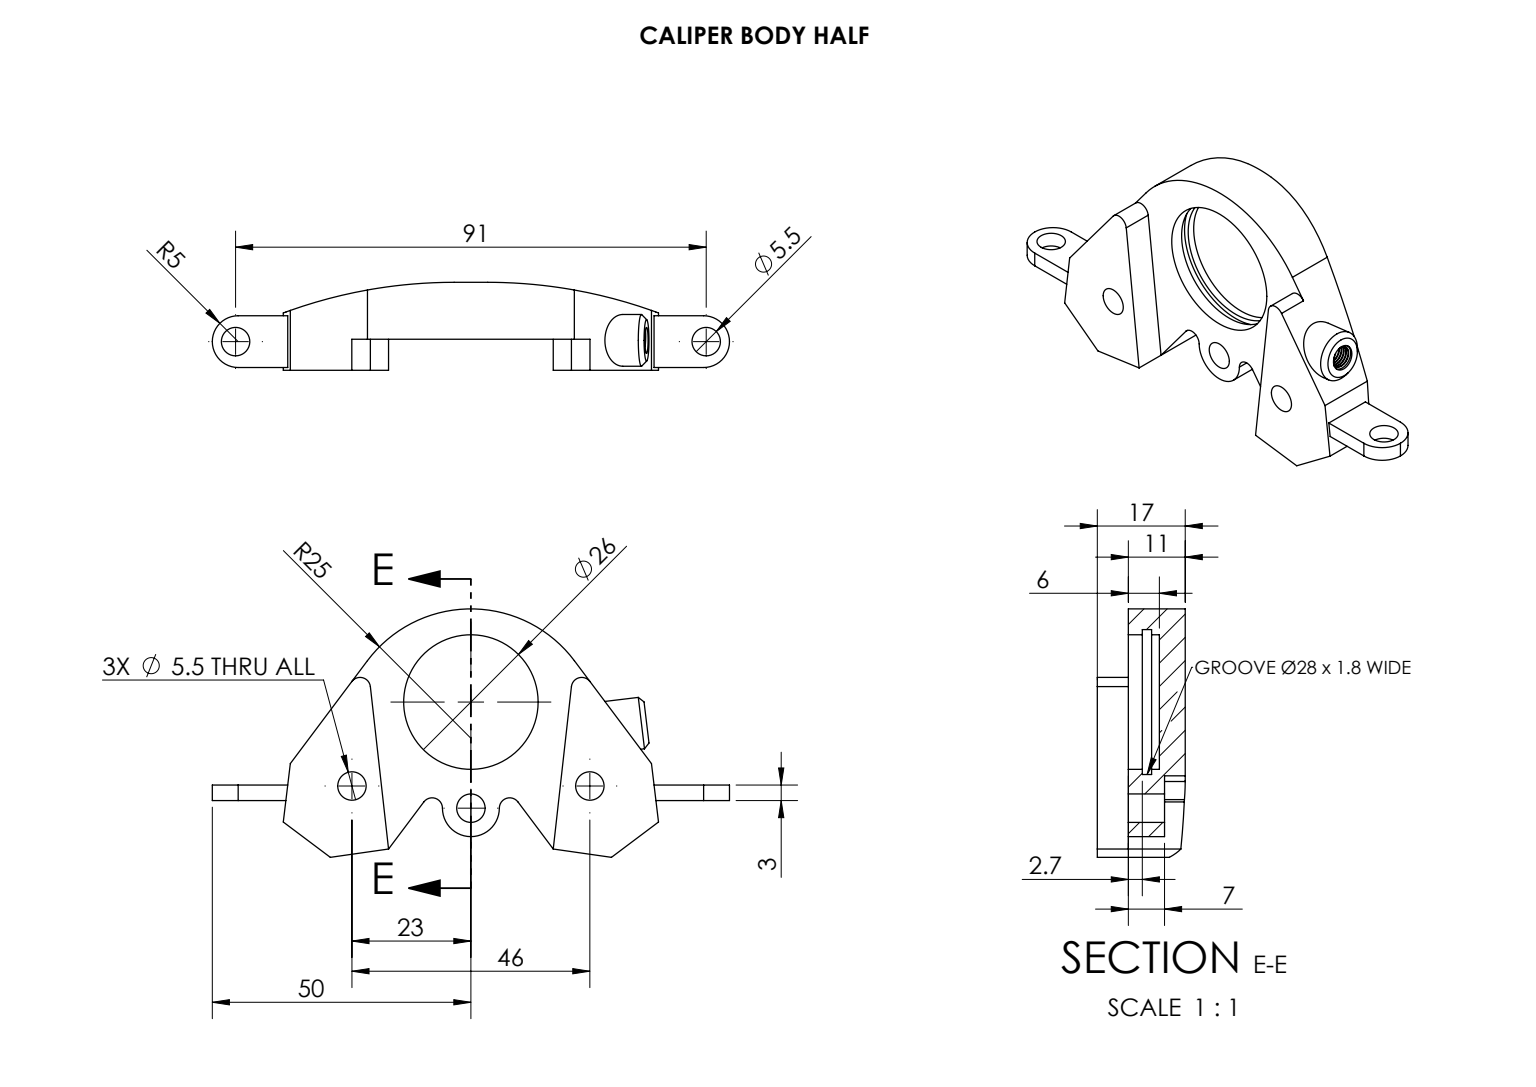
ISO-10303-21;
HEADER;
FILE_DESCRIPTION (('STEP AP214'),
    '1' );
FILE_NAME ('Caliper Body Half.step',
    '2026-09-24T10:28:59',
    ( '' ),
    ( '' ),
    'SwSTEP 2.0',
    'SolidWorks 2026',
    '' );
FILE_SCHEMA (( 'AUTOMOTIVE_DESIGN' ));
ENDSEC;

DATA;
#1=DIRECTION ( 'NONE',  ( 0.000000000000000000, 0.000000000000000000, 1.000000000000000000 ) ) ;
#7=CARTESIAN_POINT ( 'NONE',  ( 27.21934464581372737, -3.303641803799556964, -8.283357778048658915 ) ) ;
#8=CARTESIAN_POINT ( 'NONE',  ( 31.38469755857769528, -2.374701023479507178, -4.705209693361161349 ) ) ;
#10=DIRECTION ( 'NONE',  ( -0.1196152422706611984, 0.9928203230275510771, 0.000000000000000000 ) ) ;
#13=VECTOR ( 'NONE', #4443, 1000.000000000000000 ) ;
#14=EDGE_CURVE ( 'NONE', #9007, #1609, #16081, .T. ) ;
#19=AXIS2_PLACEMENT_3D ( 'NONE', #16442, #1032, #9441 ) ;
#22=CARTESIAN_POINT ( 'NONE',  ( 30.63309003953906995, -6.864245478665264244, -5.783357778048663356 ) ) ;
#23=ORIENTED_EDGE ( 'NONE', *, *, #13213, .T. ) ;
#25=ORIENTED_EDGE ( 'NONE', *, *, #5037, .F. ) ;
#26=CARTESIAN_POINT ( 'NONE',  ( 30.41294626588012306, -6.253601060580800564, -6.861505862736167138 ) ) ;
#29=VERTEX_POINT ( 'NONE', #10521 ) ;
#30=CARTESIAN_POINT ( 'NONE',  ( 26.73899421642883567, -2.634607751922174224, -4.533357778048659803 ) ) ;
#31=VECTOR ( 'NONE', #7104, 1000.000000000000114 ) ;
#36=EDGE_LOOP ( 'NONE', ( #1932, #7211, #3460, #1817 ) ) ;
#37=CARTESIAN_POINT ( 'NONE',  ( 16.95685998530892746, -17.86641812890577796, -16.00584995567978908 ) ) ;
#42=AXIS2_PLACEMENT_3D ( 'NONE', #3726, #1281, #2807 ) ;
#47=EDGE_CURVE ( 'NONE', #1330, #15856, #15716, .T. ) ;
#48=ORIENTED_EDGE ( 'NONE', *, *, #12351, .T. ) ;
#49=CARTESIAN_POINT ( 'NONE',  ( 33.55383270609817714, -5.448088258586239796, -3.283357778048667797 ) ) ;
#50=CARTESIAN_POINT ( 'NONE',  ( 29.97942892559193950, -4.424919740341219487, -3.627061608673664672 ) ) ;
#51=VECTOR ( 'NONE', #5337, 1000.000000000000000 ) ;
#52=FACE_OUTER_BOUND ( 'NONE', #13800, .T. ) ;
#70=CARTESIAN_POINT ( 'NONE',  ( 26.01652455409633902, -4.902371455920928156, -5.783357778048663356 ) ) ;
#75=ADVANCED_FACE ( 'NONE', ( #15989 ), #17272, .F. ) ;
#77=CIRCLE ( 'NONE', #17181, 2.000000000000001776 ) ;
#78=CARTESIAN_POINT ( 'NONE',  ( 16.79147592569384173, -15.38964587861223166, -16.02981638571824163 ) ) ;
#91=CARTESIAN_POINT ( 'NONE',  ( 26.87106449706838873, -6.053357334259913181, -3.627061608673667781 ) ) ;
#92=DIRECTION ( 'NONE',  ( 0.000000000000000000, 0.000000000000000000, 1.000000000000000000 ) ) ;
#93=CARTESIAN_POINT ( 'NONE',  ( 25.76466184735054910, -2.811881907026620553, -6.248149982130924762 ) ) ;
#94=CARTESIAN_POINT ( 'NONE',  ( 34.91600907648203389, -11.88801210197604341, -11.56671555609732671 ) ) ;
#99=CARTESIAN_POINT ( 'NONE',  ( 25.11802603177690330, -16.03270077640482683, -0.5379818257722508434 ) ) ;
#101=CARTESIAN_POINT ( 'NONE',  ( 28.51030546511822195, -6.055733689321201041, -3.283357778048667797 ) ) ;
#103=CARTESIAN_POINT ( 'NONE',  ( 30.62726312072365431, -1.838986382273682718, -5.783357778048658027 ) ) ;
#106=EDGE_CURVE ( 'NONE', #16432, #2761, #668, .T. ) ;
#110=ORIENTED_EDGE ( 'NONE', *, *, #14522, .T. ) ;
#113=ORIENTED_EDGE ( 'NONE', *, *, #12527, .T. ) ;
#115=ORIENTED_EDGE ( 'NONE', *, *, #562, .T. ) ;
#116=CARTESIAN_POINT ( 'NONE',  ( 28.26310972651430120, -2.123820177930694442, -5.783357778048658915 ) ) ;
#120=CARTESIAN_POINT ( 'NONE',  ( 30.15026255541241440, -6.285249260098253465, -4.705209693361168455 ) ) ;
#127=ADVANCED_FACE ( 'NONE', ( #4081 ), #12055, .F. ) ;
#134=CARTESIAN_POINT ( 'NONE',  ( -3.248936832696171617, 7.999999999999989342, -17.00000000000000000 ) ) ;
#138=CARTESIAN_POINT ( 'NONE',  ( 27.02867472334902033, -6.034368414549446058, -3.627061608673668225 ) ) ;
#139=CARTESIAN_POINT ( 'NONE',  ( 33.14105852333657509, -6.224726188408045147, -4.533357778048668685 ) ) ;
#140=CARTESIAN_POINT ( 'NONE',  ( -2.016448651773435938E-27, -20.49999999999999645, -13.00000000000000178 ) ) ;
#141=CARTESIAN_POINT ( 'NONE',  ( 31.03206908560819954, -5.751910973953721751, -3.283357778048667797 ) ) ;
#144=CARTESIAN_POINT ( 'NONE',  ( 30.66050125466253107, -2.889050389913576655, -3.283357778048662023 ) ) ;
#146=ORIENTED_EDGE ( 'NONE', *, *, #8317, .T. ) ;
#163=CARTESIAN_POINT ( 'NONE',  ( 28.29479612530171551, -12.89112598890823946, -13.63906826012424922 ) ) ;
#164=DIRECTION ( 'NONE',  ( 1.000000000000000000, 0.000000000000000000, 0.000000000000000000 ) ) ;
#167=EDGE_LOOP ( 'NONE', ( #6855, #14181, #5684, #15430, #4604, #9201, #7856, #12095, #740, #13288, #12189, #5777, #2747, #13452, #12769, #7783, #17571, #8793, #8444, #8354, #17242, #15258, #14922, #10965, #8092, #5094, #9620, #17228, #363 ) ) ;
#169=FACE_BOUND ( 'NONE', #9729, .T. ) ;
#170=ORIENTED_EDGE ( 'NONE', *, *, #10749, .T. ) ;
#176=CARTESIAN_POINT ( 'NONE',  ( 25.99795558426325215, -4.648046406214923820, -3.627061608673664228 ) ) ;
#177=FACE_OUTER_BOUND ( 'NONE', #11097, .T. ) ;
#181=CARTESIAN_POINT ( 'NONE',  ( 31.97277696464621854, -6.702839660918840536, -5.783357778048663356 ) ) ;
#182=EDGE_CURVE ( 'NONE', #5342, #17048, #16351, .T. ) ;
#183=DIRECTION ( 'NONE',  ( 1.000000000000000000, 0.000000000000000000, 0.000000000000000000 ) ) ;
#185=CARTESIAN_POINT ( 'NONE',  ( -27.17934203385504333, -30.00000000000000355, -13.93658524716016878 ) ) ;
#186=CARTESIAN_POINT ( 'NONE',  ( 29.18195272205665347, -2.340279496617377664, -4.533357778048659803 ) ) ;
#188=CARTESIAN_POINT ( 'NONE',  ( 31.41114436565740320, -6.133337902414513820, -4.705209693361168455 ) ) ;
#194=EDGE_CURVE ( 'NONE', #11172, #2496, #13438, .T. ) ;
#206=( BOUNDED_CURVE ( )  B_SPLINE_CURVE ( 2, ( #6130, #9128, #12848, #438, #15840, #5943, #14486, #14392, #13119 ),
 .UNSPECIFIED., .F., .T. ) 
 B_SPLINE_CURVE_WITH_KNOTS ( ( 3, 2, 2, 2, 3 ),
 ( 0.6730769230769231282, 0.6794871794871795156, 0.6923076923076922906, 0.7051282051282051766, 0.7115384615384615641 ),
 .UNSPECIFIED. ) 
 CURVE ( )  GEOMETRIC_REPRESENTATION_ITEM ( )  RATIONAL_B_SPLINE_CURVE ( ( 0.9330127018922192983, 0.9330127018922198534, 1.000000000000000000, 0.8660254037844387076, 1.000000000000000000, 0.8660254037844387076, 1.000000000000000000, 0.9330127018922194093, 0.9330127018922194093 ) ) 
 REPRESENTATION_ITEM ( '' )  );
#208=CARTESIAN_POINT ( 'NONE',  ( 28.86293393808771057, -2.678523738846987357, -4.705209693361161349 ) ) ;
#213=ORIENTED_EDGE ( 'NONE', *, *, #17178, .T. ) ;
#218=EDGE_CURVE ( 'NONE', #17680, #17749, #13335, .T. ) ;
#222=CARTESIAN_POINT ( 'NONE',  ( -25.11802603177690330, -19.03270077640482683, -10.53798182577225084 ) ) ;
#227=VERTEX_POINT ( 'NONE', #1284 ) ;
#229=CARTESIAN_POINT ( 'NONE',  ( 25.93488947238681774, -5.606027099510431988, -7.939653947423663816 ) ) ;
#231=CARTESIAN_POINT ( 'NONE',  ( 31.74131510559286085, -5.666460835049168310, -3.283357778048667797 ) ) ;
#236=DIRECTION ( 'NONE',  ( 0.000000000000000000, 0.000000000000000000, 1.000000000000000000 ) ) ;
#244=CARTESIAN_POINT ( 'NONE',  ( 26.00347982711925710, -2.723222710571018279, -7.033357778048658027 ) ) ;
#257=CARTESIAN_POINT ( 'NONE',  ( 19.43845002722867221, 2.988003976273735596, -6.000000000000000000 ) ) ;
#261=VECTOR ( 'NONE', #7073, 1000.000000000000227 ) ;
#263=CARTESIAN_POINT ( 'NONE',  ( -9.099998387031003944, -19.29508120620799616, -16.81964500401478091 ) ) ;
#270=CARTESIAN_POINT ( 'NONE',  ( 23.00000000000000000, -16.21813761408365195, -13.00000000000000178 ) ) ;
#278=EDGE_CURVE ( 'NONE', #1298, #15606, #15319, .T. ) ;
#282=CARTESIAN_POINT ( 'NONE',  ( 28.88938074516742205, -6.437160617781993999, -4.705209693361168455 ) ) ;
#287=DIRECTION ( 'NONE',  ( -0.1196152422706621005, -0.9928203230275509661, 0.000000000000000000 ) ) ;
#292=CARTESIAN_POINT ( 'NONE',  ( -35.77680296528374271, -19.03270077640482683, -10.53798182577225084 ) ) ;
#294=CARTESIAN_POINT ( 'NONE',  ( -19.22778933661430756, -11.21824206523807099, -15.64718775662042560 ) ) ;
#295=ORIENTED_EDGE ( 'NONE', *, *, #12061, .T. ) ;
#298=CARTESIAN_POINT ( 'NONE',  ( 26.51200394741821498, -4.842675973971495296, -7.939653947423662039 ) ) ;
#301=CARTESIAN_POINT ( 'NONE',  ( 30.45225960443380231, -4.367952981209816343, -3.627061608673664672 ) ) ;
#307=EDGE_CURVE ( 'NONE', #987, #12566, #1185, .T. ) ;
#319=DIRECTION ( 'NONE',  ( -0.000000000000000000, 1.000000000000000000, 0.000000000000000000 ) ) ;
#325=CARTESIAN_POINT ( 'NONE',  ( 27.28266178881210280, -7.257709054644824853, -5.783357778048669573 ) ) ;
#326=ADVANCED_FACE ( 'NONE', ( #3086 ), #2732, .F. ) ;
#327=CARTESIAN_POINT ( 'NONE',  ( 31.11087420047036289, -5.742416513891037688, -3.283357778048667797 ) ) ;
#329=FACE_BOUND ( 'NONE', #8817, .T. ) ;
#331=CARTESIAN_POINT ( 'NONE',  ( 29.04699097144805364, -6.418171698071525100, -4.705209693361169343 ) ) ;
#338=VECTOR ( 'NONE', #16087, 1000.000000000000000 ) ;
#343=CARTESIAN_POINT ( 'NONE',  ( -36.27615609941022257, -23.17738945083361557, 0.000000000000000000 ) ) ;
#349=CARTESIAN_POINT ( 'NONE',  ( 33.56434302664245450, -9.029166375164061620, -5.783357778048662468 ) ) ;
#350=FACE_OUTER_BOUND ( 'NONE', #12268, .T. ) ;
#353=CARTESIAN_POINT ( 'NONE',  ( -23.00000000000000000, -16.21813761408365195, -13.00000000000000178 ) ) ;
#354=AXIS2_PLACEMENT_3D ( 'NONE', #5840, #1963, #15742 ) ;
#363=ORIENTED_EDGE ( 'NONE', *, *, #1585, .T. ) ;
#376=AXIS2_PLACEMENT_3D ( 'NONE', #11104, #8407, #9745 ) ;
#380=CARTESIAN_POINT ( 'NONE',  ( 29.62036837594175154, -3.214238380052812261, -3.627061608673662896 ) ) ;
#382=DIRECTION ( 'NONE',  ( -0.000000000000000000, -0.000000000000000000, 1.000000000000000000 ) ) ;
#383=CARTESIAN_POINT ( 'NONE',  ( 25.97837335112617652, -4.585712065882579402, -3.626324104489874411 ) ) ;
#386=FACE_OUTER_BOUND ( 'NONE', #5358, .T. ) ;
#393=CYLINDRICAL_SURFACE ( 'NONE', #607, 6.249999999999998224 ) ;
#396=CARTESIAN_POINT ( 'NONE',  ( 28.54354359905709160, -7.105797696961086096, -5.783357778048669573 ) ) ;
#398=CARTESIAN_POINT ( 'NONE',  ( 31.25770402584614516, -1.763030703431812674, -5.783357778048658027 ) ) ;
#399=CARTESIAN_POINT ( 'NONE',  ( 33.95908713831674675, -3.945449517755636126, -5.783357778048663356 ) ) ;
#400=CARTESIAN_POINT ( 'NONE',  ( 25.71748644841968456, -2.420320648352051851, -5.783357778048663356 ) ) ;
#401=DIRECTION ( 'NONE',  ( 0.000000000000000000, 0.000000000000000000, -1.000000000000000000 ) ) ;
#402=ORIENTED_EDGE ( 'NONE', *, *, #10796, .T. ) ;
#404=DIRECTION ( 'NONE',  ( -0.6000000000000000888, -0.7999999999999999334, 0.000000000000000000 ) ) ;
#405=ORIENTED_EDGE ( 'NONE', *, *, #3183, .F. ) ;
#411=CARTESIAN_POINT ( 'NONE',  ( 25.71748644841968456, -2.420320648352051851, -5.783357778048663356 ) ) ;
#420=CARTESIAN_POINT ( 'NONE',  ( 25.76326615456878244, -3.051972493152843580, -6.861505862736158257 ) ) ;
#421=CARTESIAN_POINT ( 'NONE',  ( 30.38277803966508372, -1.468696967828331701, -5.783357778048658027 ) ) ;
#424=CARTESIAN_POINT ( 'NONE',  ( 29.76058531221316628, -5.705227139567997874, -7.939653947423664704 ) ) ;
#436=CARTESIAN_POINT ( 'NONE',  ( 25.98779870451785001, -2.387753359738024272, -6.453230759126469707 ) ) ;
#438=CARTESIAN_POINT ( 'NONE',  ( 28.51030546511822195, -6.055733689321201041, -3.283357778048667797 ) ) ;
#443=EDGE_CURVE ( 'NONE', #1609, #16681, #2190, .T. ) ;
#453=ORIENTED_EDGE ( 'NONE', *, *, #654, .T. ) ;
#456=CARTESIAN_POINT ( 'NONE',  ( 26.45077056032005913, -6.103994453487816330, -7.939653947423662927 ) ) ;
#458=FACE_BOUND ( 'NONE', #16476, .T. ) ;
#466=CARTESIAN_POINT ( 'NONE',  ( 33.56515079149260572, -5.873822666371450119, -6.861505862736167138 ) ) ;
#468=DIRECTION ( 'NONE',  ( -1.000000000000000000, 0.000000000000000000, 0.000000000000000000 ) ) ;
#474=CARTESIAN_POINT ( 'NONE',  ( -45.00000000000000711, -19.03270077640483038, -5.537981825772250843 ) ) ;
#479=CARTESIAN_POINT ( 'NONE',  ( 25.86833963875586306, -3.039313213345869791, -4.705209693361160461 ) ) ;
#481=CARTESIAN_POINT ( 'NONE',  ( 30.88125018618674744, -3.062327022369072171, -3.627061608673662896 ) ) ;
#487=CARTESIAN_POINT ( 'NONE',  ( -23.00000000000000000, -16.21813761408365195, 0.000000000000000000 ) ) ;
#491=ORIENTED_EDGE ( 'NONE', *, *, #2769, .T. ) ;
#492=FACE_OUTER_BOUND ( 'NONE', #1631, .T. ) ;
#495=CARTESIAN_POINT ( 'NONE',  ( -36.27615609941022257, -23.17738945083361557, 0.000000000000000000 ) ) ;
#496=VERTEX_POINT ( 'NONE', #3169 ) ;
#497=DIRECTION ( 'NONE',  ( 0.000000000000000000, 0.000000000000000000, 1.000000000000000000 ) ) ;
#498=ADVANCED_FACE ( 'NONE', ( #4791 ), #9064, .T. ) ;
#505=DIRECTION ( 'NONE',  ( 0.7999999999999999334, -0.6000000000000001998, 0.000000000000000000 ) ) ;
#510=EDGE_CURVE ( 'NONE', #9324, #14027, #3441, .T. ) ;
#512=VERTEX_POINT ( 'NONE', #11862 ) ;
#521=CARTESIAN_POINT ( 'NONE',  ( 26.79905070906539777, -3.354278923027479209, -3.283357778048662023 ) ) ;
#538=DIRECTION ( 'NONE',  ( -1.000000000000000000, 0.000000000000000000, 0.000000000000000000 ) ) ;
#546=ORIENTED_EDGE ( 'NONE', *, *, #3072, .T. ) ;
#548=VERTEX_POINT ( 'NONE', #6338 ) ;
#550=CARTESIAN_POINT ( 'NONE',  ( 25.62757597683262034, -3.695291012717980994, -7.939653947423660263 ) ) ;
#559=CARTESIAN_POINT ( 'NONE',  ( 32.54050588463559990, -2.235448945602741766, -6.861505862736159145 ) ) ;
#562=EDGE_CURVE ( 'NONE', #5268, #9522, #10410, .T. ) ;
#565=CARTESIAN_POINT ( 'NONE',  ( 26.63030083514515312, -6.709335133632020387, -6.861505862736167138 ) ) ;
#566=CARTESIAN_POINT ( 'NONE',  ( 27.89118264539014547, -6.557423775948280742, -6.861505862736167138 ) ) ;
#570=CARTESIAN_POINT ( 'NONE',  ( 27.51889869220010354, -3.467423976192371082, -7.939653947423660263 ) ) ;
#572=CARTESIAN_POINT ( 'NONE',  ( 33.52375369703867847, -2.544085015380856518, -8.283357778048660691 ) ) ;
#573=DIRECTION ( 'NONE',  ( 0.000000000000000000, 0.000000000000000000, 1.000000000000000000 ) ) ;
#575=VECTOR ( 'NONE', #16775, 1000.000000000000000 ) ;
#582=EDGE_LOOP ( 'NONE', ( #8490, #11002, #7089, #14364 ) ) ;
#589=CARTESIAN_POINT ( 'NONE',  ( 27.89480254248674740, -2.495355674045408367, -7.033357778048658027 ) ) ;
#607=AXIS2_PLACEMENT_3D ( 'NONE', #12704, #14260, #1658 ) ;
#608=EDGE_CURVE ( 'NONE', #17849, #6537, #15603, .T. ) ;
#610=VECTOR ( 'NONE', #16049, 1000.000000000000000 ) ;
#613=B_SPLINE_CURVE_WITH_KNOTS ( 'NONE', 3,
 ( #7742, #1957, #7477, #13001 ),
 .UNSPECIFIED., .F., .F.,
 ( 4, 4 ),
 ( 4.336808689942017736E-19, 0.0003446252387907799432 ),
 .UNSPECIFIED. ) ;
#615=CARTESIAN_POINT ( 'NONE',  ( 33.46007730730551799, -5.886481946178435010, -4.705209693361169343 ) ) ;
#618=DIRECTION ( 'NONE',  ( -0.000000000000000000, 0.000000000000000000, -1.000000000000000000 ) ) ;
#621=AXIS2_PLACEMENT_3D ( 'NONE', #3165, #7357, #17152 ) ;
#622=CARTESIAN_POINT ( 'NONE',  ( 26.85044460880409645, -7.319979551716484067, -5.783357778048668685 ) ) ;
#630=FACE_OUTER_BOUND ( 'NONE', #1139, .T. ) ;
#637=CARTESIAN_POINT ( 'NONE',  ( 26.31284730449749532, -7.327874027665321144, -6.311983372246984914 ) ) ;
#640=EDGE_CURVE ( 'NONE', #12566, #987, #8142, .T. ) ;
#644=CARTESIAN_POINT ( 'NONE',  ( 26.46816385032927599, -3.594016774262162706, -3.627061608673662896 ) ) ;
#646=DIRECTION ( 'NONE',  ( 0.9928203230275512992, 0.1196152422706614898, -0.000000000000000000 ) ) ;
#650=CARTESIAN_POINT ( 'NONE',  ( 29.08935247050201767, -2.014077381790315702, -5.783357778048658027 ) ) ;
#651=CARTESIAN_POINT ( 'NONE',  ( 30.65370992780335868, -5.597623261208692469, -3.627061608673667781 ) ) ;
#654=EDGE_CURVE ( 'NONE', #11172, #12535, #8280, .T. ) ;
#656=CARTESIAN_POINT ( 'NONE',  ( 25.76466184735054910, -2.811881907026620553, -6.248149982130924762 ) ) ;
#660=CARTESIAN_POINT ( 'NONE',  ( 25.60565592828815440, -3.070961412863312034, -6.861505862736159145 ) ) ;
#661=DIRECTION ( 'NONE',  ( 0.9928203230275511881, 0.1196152422706614760, 0.000000000000000000 ) ) ;
#662=CARTESIAN_POINT ( 'NONE',  ( 27.21934464581372737, -3.303641803799556964, -8.283357778048660691 ) ) ;
#665=DIRECTION ( 'NONE',  ( -1.000000000000000000, 0.000000000000000000, 0.000000000000000000 ) ) ;
#668=( BOUNDED_CURVE ( )  B_SPLINE_CURVE ( 2, ( #3728, #6807, #10599, #14882, #17820, #3994, #2388, #2468, #7905 ),
 .UNSPECIFIED., .F., .T. ) 
 B_SPLINE_CURVE_WITH_KNOTS ( ( 3, 2, 2, 2, 3 ),
 ( 0.5961538461538461453, 0.6025641025641025328, 0.6153846153846154188, 0.6282051282051281937, 0.6346153846153846922 ),
 .UNSPECIFIED. ) 
 CURVE ( )  GEOMETRIC_REPRESENTATION_ITEM ( )  RATIONAL_B_SPLINE_CURVE ( ( 0.9330127018922194093, 0.9330127018922194093, 1.000000000000000000, 0.8660254037844387076, 1.000000000000000000, 0.8660254037844387076, 1.000000000000000000, 0.9330127018922187432, 0.9330127018922192983 ) ) 
 REPRESENTATION_ITEM ( '' )  );
#669=ORIENTED_EDGE ( 'NONE', *, *, #13024, .T. ) ;
#672=CARTESIAN_POINT ( 'NONE',  ( 33.78529456515154550, -6.484467084455913799, -5.783357778048663356 ) ) ;
#680=CARTESIAN_POINT ( 'NONE',  ( 28.76917853929504432, -3.116917426439186123, -3.283357778048662023 ) ) ;
#681=DIRECTION ( 'NONE',  ( 0.000000000000000000, 3.469446951953614189E-16, -1.000000000000000000 ) ) ;
#687=CARTESIAN_POINT ( 'NONE',  ( 27.42949161418789217, -3.278323244185609830, -3.283357778048662023 ) ) ;
#689=VECTOR ( 'NONE', #8945, 999.9999999999998863 ) ;
#703=CARTESIAN_POINT ( 'NONE',  ( 16.75000000000000000, -16.21813761408365195, -16.03574476417184513 ) ) ;
#706=CYLINDRICAL_SURFACE ( 'NONE', #12142, 2.499999999999999112 ) ;
#708=ORIENTED_EDGE ( 'NONE', *, *, #6551, .F. ) ;
#720=CARTESIAN_POINT ( 'NONE',  ( -18.31859240410168255, -20.37927276054855596, -15.79761704335050077 ) ) ;
#724=( BOUNDED_CURVE ( )  B_SPLINE_CURVE ( 2, ( #2368, #1077, #16328, #7886, #2524, #10922, #2617, #16488, #13677 ),
 .UNSPECIFIED., .F., .T. ) 
 B_SPLINE_CURVE_WITH_KNOTS ( ( 3, 2, 2, 2, 3 ),
 ( 0.5576923076923077094, 0.5641025641025640969, 0.5769230769230768718, 0.5897435897435897578, 0.5961538461538461453 ),
 .UNSPECIFIED. ) 
 CURVE ( )  GEOMETRIC_REPRESENTATION_ITEM ( )  RATIONAL_B_SPLINE_CURVE ( ( 0.9330127018922194093, 0.9330127018922194093, 1.000000000000000000, 0.8660254037844387076, 1.000000000000000000, 0.8660254037844387076, 1.000000000000000000, 0.9330127018922194093, 0.9330127018922194093 ) ) 
 REPRESENTATION_ITEM ( '' )  );
#728=ORIENTED_EDGE ( 'NONE', *, *, #15440, .F. ) ;
#730=CARTESIAN_POINT ( 'NONE',  ( 27.62849893492243325, -6.589071975465733644, -4.705209693361168455 ) ) ;
#736=EDGE_LOOP ( 'NONE', ( #2850, #16797, #4603, #10052 ) ) ;
#739=CARTESIAN_POINT ( 'NONE',  ( 30.25080928106424594, -3.138282701210941994, -3.627061608673662896 ) ) ;
#740=ORIENTED_EDGE ( 'NONE', *, *, #17456, .F. ) ;
#742=CARTESIAN_POINT ( 'NONE',  ( 45.50000000000000000, -16.03270077640482683, -8.287981825772241962 ) ) ;
#745=CARTESIAN_POINT ( 'NONE',  ( 27.65911562847151117, -5.958412735707574015, -3.627061608673668225 ) ) ;
#747=CARTESIAN_POINT ( 'NONE',  ( 27.47505859511117521, -2.218764776483033163, -5.783357778048658027 ) ) ;
#754=ORIENTED_EDGE ( 'NONE', *, *, #7062, .T. ) ;
#756=EDGE_CURVE ( 'NONE', #1298, #13310, #2088, .T. ) ;
#760=DIRECTION ( 'NONE',  ( 0.000000000000000000, 0.000000000000000000, -1.000000000000000000 ) ) ;
#761=VERTEX_POINT ( 'NONE', #2823 ) ;
#762=LINE ( 'NONE', #10269, #2689 ) ;
#765=CARTESIAN_POINT ( 'NONE',  ( 32.04575515724927470, -1.668086104879473730, -5.783357778048658915 ) ) ;
#767=CARTESIAN_POINT ( 'NONE',  ( 27.95866967485789090, -6.122194908100387245, -3.283357778048667797 ) ) ;
#774=FACE_OUTER_BOUND ( 'NONE', #2018, .T. ) ;
#782=EDGE_LOOP ( 'NONE', ( #7919, #8135, #1228, #9710 ) ) ;
#798=ORIENTED_EDGE ( 'NONE', *, *, #7563, .F. ) ;
#799=ORIENTED_EDGE ( 'NONE', *, *, #2607, .T. ) ;
#805=CARTESIAN_POINT ( 'NONE',  ( -16.96458082634299558, -17.85487492059188597, -16.00470661676384054 ) ) ;
#810=CARTESIAN_POINT ( 'NONE',  ( 30.00264913441657555, -6.940201157507134511, -5.783357778048657138 ) ) ;
#813=CARTESIAN_POINT ( 'NONE',  ( 33.35047706458318828, -2.764833946905071560, -7.939653947423660263 ) ) ;
#815=EDGE_LOOP ( 'NONE', ( #969, #7998, #5616, #17835 ) ) ;
#820=AXIS2_PLACEMENT_3D ( 'NONE', #12110, #886, #3877 ) ;
#824=CARTESIAN_POINT ( 'NONE',  ( 31.53813789838894621, -6.745008222462202774, -5.783357778048668685 ) ) ;
#826=EDGE_CURVE ( 'NONE', #11736, #17680, #13359, .T. ) ;
#828=CARTESIAN_POINT ( 'NONE',  ( 31.00199007654869732, -2.847907730748336697, -8.283357778048660691 ) ) ;
#835=CARTESIAN_POINT ( 'NONE',  ( 32.47301885516785092, -2.670677813450649474, -3.283357778048662023 ) ) ;
#836=CARTESIAN_POINT ( 'NONE',  ( 26.99805802979993885, -6.665027654307603022, -4.705209693361168455 ) ) ;
#838=CARTESIAN_POINT ( 'NONE',  ( -50.00000000000000000, -16.03270077640482683, -5.537981825772250843 ) ) ;
#846=ORIENTED_EDGE ( 'NONE', *, *, #2531, .T. ) ;
#847=DIRECTION ( 'NONE',  ( -0.000000000000000000, 1.000000000000000000, -0.000000000000000000 ) ) ;
#854=CARTESIAN_POINT ( 'NONE',  ( 30.25524682244395436, -4.391689130744175884, -3.283357778048664688 ) ) ;
#857=DIRECTION ( 'NONE',  ( 1.000000000000000000, 0.000000000000000000, 0.000000000000000000 ) ) ;
#859=ORIENTED_EDGE ( 'NONE', *, *, #7991, .T. ) ;
#866=ORIENTED_EDGE ( 'NONE', *, *, #16999, .T. ) ;
#868=EDGE_LOOP ( 'NONE', ( #110, #4824, #5826, #15634 ) ) ;
#871=DIRECTION ( 'NONE',  ( 0.9928203230275510771, 0.1196152422706614621, -0.000000000000000000 ) ) ;
#877=CARTESIAN_POINT ( 'NONE',  ( 32.72003615946069743, -2.840789625746940938, -7.939653947423660263 ) ) ;
#878=( BOUNDED_CURVE ( )  B_SPLINE_CURVE ( 3, ( #12266, #2658, #4104, #17834 ),
 .UNSPECIFIED., .F., .T. ) 
 B_SPLINE_CURVE_WITH_KNOTS ( ( 4, 4 ),
 ( 4.715434792643774742, 4.769085813125753859 ),
 .UNSPECIFIED. ) 
 CURVE ( )  GEOMETRIC_REPRESENTATION_ITEM ( )  RATIONAL_B_SPLINE_CURVE ( ( 1.000000000000000000, 0.9997601450507493936, 0.9997601450507493936, 1.000000000000000000 ) ) 
 REPRESENTATION_ITEM ( '' )  );
#885=CARTESIAN_POINT ( 'NONE',  ( 32.47301885516785092, -2.670677813450649918, -3.283357778048662023 ) ) ;
#886=DIRECTION ( 'NONE',  ( 0.000000000000000000, 1.000000000000000000, 3.469446951953614189E-16 ) ) ;
#900=CARTESIAN_POINT ( 'NONE',  ( 27.26436163736424945, -2.571311352887278190, -7.033357778048658027 ) ) ;
#905=CARTESIAN_POINT ( 'NONE',  ( 27.23882169172318513, -6.009049854935478052, -7.939653947423664704 ) ) ;
#907=CARTESIAN_POINT ( 'NONE',  ( 29.74110826630371207, -2.999819088432076786, -8.283357778048660691 ) ) ;
#910=CARTESIAN_POINT ( 'NONE',  ( 31.02146712245815507, -5.553315781884258229, -7.939653947423664704 ) ) ;
#913=CARTESIAN_POINT ( 'NONE',  ( -9.099998387031003944, -19.29508120620799616, -12.00000000000000000 ) ) ;
#917=ORIENTED_EDGE ( 'NONE', *, *, #307, .T. ) ;
#919=COLOUR_RGB ( '', 0.40784314, 0.44705882, 0.49803922) ;
#920=CARTESIAN_POINT ( 'NONE',  ( 33.42946061375642586, -6.517141185936593750, -5.783357778048668685 ) ) ;
#923=CARTESIAN_POINT ( 'NONE',  ( 31.24221605398236079, -5.726592414339752857, -8.283357778048664244 ) ) ;
#927=CARTESIAN_POINT ( 'NONE',  ( 30.80688261270428541, -4.325227911964988792, -3.283357778048664688 ) ) ;
#929=CARTESIAN_POINT ( 'NONE',  ( 28.14933959732260149, -3.391468297350501260, -7.939653947423660263 ) ) ;
#931=DIRECTION ( 'NONE',  ( 1.000000000000000000, 0.000000000000000000, 0.000000000000000000 ) ) ;
#933=CARTESIAN_POINT ( 'NONE',  ( 20.00000000000000000, 7.999999999999996447, -15.51150668642334374 ) ) ;
#938=EDGE_CURVE ( 'NONE', #6497, #761, #8426, .T. ) ;
#941=ORIENTED_EDGE ( 'NONE', *, *, #14365, .T. ) ;
#943=DIRECTION ( 'NONE',  ( -0.9937818688019538493, -0.1113444980252557837, 0.000000000000000000 ) ) ;
#947=VERTEX_POINT ( 'NONE', #13962 ) ;
#948=CARTESIAN_POINT ( 'NONE',  ( 26.92924972366625980, -7.310485091653801781, -5.783357778048657138 ) ) ;
#951=AXIS2_PLACEMENT_3D ( 'NONE', #9490, #8145, #8230 ) ;
#952=CARTESIAN_POINT ( 'NONE',  ( 29.98885399772409954, -6.604504582617394703, -4.533357778048668685 ) ) ;
#953=FACE_OUTER_BOUND ( 'NONE', #4533, .T. ) ;
#958=CARTESIAN_POINT ( 'NONE',  ( 25.76466184735054910, -2.811881907026620553, -6.248149982130924762 ) ) ;
#963=VERTEX_POINT ( 'NONE', #7084 ) ;
#969=ORIENTED_EDGE ( 'NONE', *, *, #6749, .F. ) ;
#970=CARTESIAN_POINT ( 'NONE',  ( -14.00000000000000178, 0.000000000000000000, -10.50000000000000000 ) ) ;
#974=CARTESIAN_POINT ( 'NONE',  ( 33.54323074294813267, -5.249493066516778050, -7.939653947423664704 ) ) ;
#977=DIRECTION ( 'NONE',  ( 0.000000000000000000, 1.000000000000000000, 0.000000000000000000 ) ) ;
#978=DIRECTION ( 'NONE',  ( 0.9928203230275511881, 0.1196152422706614482, 0.000000000000000000 ) ) ;
#980=CARTESIAN_POINT ( 'NONE',  ( 30.08145424927873535, -6.930706697444451336, -5.783357778048663356 ) ) ;
#981=CARTESIAN_POINT ( 'NONE',  ( 33.06225340847440464, -6.234220648470727433, -4.533357778048668685 ) ) ;
#985=EDGE_CURVE ( 'NONE', #8671, #5626, #17505, .T. ) ;
#987=VERTEX_POINT ( 'NONE', #5692 ) ;
#992=EDGE_CURVE ( 'NONE', #12531, #11629, #15318, .T. ) ;
#993=ORIENTED_EDGE ( 'NONE', *, *, #16072, .T. ) ;
#995=CARTESIAN_POINT ( 'NONE',  ( -1.917618200156724081E-28, -7.000000000000001776, 0.000000000000000000 ) ) ;
#997=CARTESIAN_POINT ( 'NONE',  ( 45.50000000000000000, -19.03270077640483038, -2.787981825772258837 ) ) ;
#1002=CARTESIAN_POINT ( 'NONE',  ( 26.37178701114681800, -2.351687214456304353, -5.783357778048658027 ) ) ;
#1005=CARTESIAN_POINT ( 'NONE',  ( 32.08959525433819238, -2.916745304588811649, -7.939653947423660263 ) ) ;
#1014=CARTESIAN_POINT ( 'NONE',  ( 27.49697864365563760, -2.843094376337701679, -6.861505862736159145 ) ) ;
#1015=( BOUNDED_CURVE ( )  B_SPLINE_CURVE ( 2, ( #2395, #4004, #11890, #2216, #3919, #7910, #7995, #9432, #7729 ),
 .UNSPECIFIED., .F., .T. ) 
 B_SPLINE_CURVE_WITH_KNOTS ( ( 3, 2, 2, 2, 3 ),
 ( 0.1346153846153846367, 0.1410256410256410242, 0.1538461538461538547, 0.1666666666666666574, 0.1730769230769231004 ),
 .UNSPECIFIED. ) 
 CURVE ( )  GEOMETRIC_REPRESENTATION_ITEM ( )  RATIONAL_B_SPLINE_CURVE ( ( 0.9330127018922194093, 0.9330127018922196314, 1.000000000000000000, 0.8660254037844387076, 1.000000000000000000, 0.8660254037844387076, 1.000000000000000000, 0.9330127018922190762, 0.9330127018922194093 ) ) 
 REPRESENTATION_ITEM ( '' )  );
#1016=CARTESIAN_POINT ( 'NONE',  ( 26.14833026707293939, -5.996374093462653931, -8.004211544232147091 ) ) ;
#1019=EDGE_CURVE ( 'NONE', #12756, #8671, #10603, .T. ) ;
#1020=CARTESIAN_POINT ( 'NONE',  ( 33.13353876934984754, -5.498725377814142945, -8.283357778048662468 ) ) ;
#1023=CARTESIAN_POINT ( 'NONE',  ( 32.02836186724004364, -4.178063784105134459, -7.939653947423662039 ) ) ;
#1024=CARTESIAN_POINT ( 'NONE',  ( -13.00000000000000178, 1.592040838891559293E-15, -12.00000000000000000 ) ) ;
#1025=FACE_OUTER_BOUND ( 'NONE', #3424, .T. ) ;
#1026=CARTESIAN_POINT ( 'NONE',  ( 18.99795248260418745, 9.336063356527739998, -15.69100717631305031 ) ) ;
#1030=FACE_OUTER_BOUND ( 'NONE', #16056, .T. ) ;
#1032=DIRECTION ( 'NONE',  ( 0.9928203230275512992, 0.1196152422706614898, -0.000000000000000000 ) ) ;
#1040=CARTESIAN_POINT ( 'NONE',  ( 27.46709037723411839, -6.908327297984874882, -4.533357778048668685 ) ) ;
#1041=DIRECTION ( 'NONE',  ( 1.000000000000000000, 0.000000000000000000, 0.000000000000000000 ) ) ;
#1053=ORIENTED_EDGE ( 'NONE', *, *, #7902, .T. ) ;
#1056=EDGE_CURVE ( 'NONE', #13311, #2108, #11302, .T. ) ;
#1058=CARTESIAN_POINT ( 'NONE',  ( 30.30787278169304244, -6.266260340387784566, -4.705209693361169343 ) ) ;
#1063=CARTESIAN_POINT ( 'NONE',  ( 0.000000000000000000, 0.000000000000000000, -10.50000000000000000 ) ) ;
#1064=ADVANCED_FACE ( 'NONE', ( #3085 ), #7359, .F. ) ;
#1073=ORIENTED_EDGE ( 'NONE', *, *, #2262, .F. ) ;
#1075=LINE ( 'NONE', #6598, #7885 ) ;
#1077=CARTESIAN_POINT ( 'NONE',  ( 28.50956232500783472, -2.083930644370540985, -6.453230759126464378 ) ) ;
#1079=EDGE_CURVE ( 'NONE', #5626, #14839, #12411, .T. ) ;
#1081=CARTESIAN_POINT ( 'NONE',  ( 27.86926259684567597, -5.933094176093606897, -7.939653947423664704 ) ) ;
#1082=CARTESIAN_POINT ( 'NONE',  ( 29.71979337562451207, -1.938121702948446323, -5.783357778048664244 ) ) ;
#1083=CARTESIAN_POINT ( 'NONE',  ( 30.80679339554874119, -2.444327062417882779, -6.861505862736158257 ) ) ;
#1089=CARTESIAN_POINT ( 'NONE',  ( -2.016448651773435938E-27, -20.49999999999999645, -17.00000000000000000 ) ) ;
#1091=CIRCLE ( 'NONE', #3704, 2.000000000000001776 ) ;
#1092=ORIENTED_EDGE ( 'NONE', *, *, #6411, .F. ) ;
#1094=CARTESIAN_POINT ( 'NONE',  ( 27.75549246765397271, -7.200742295513424374, -5.783357778048668685 ) ) ;
#1100=CARTESIAN_POINT ( 'NONE',  ( 30.67935139548315604, -7.248220074880824981, -5.783357778048669573 ) ) ;
#1101=CIRCLE ( 'NONE', #12980, 2.749999999999988454 ) ;
#1111=ADVANCED_FACE ( 'NONE', ( #3631 ), #15964, .F. ) ;
#1112=ORIENTED_EDGE ( 'NONE', *, *, #278, .T. ) ;
#1114=ORIENTED_EDGE ( 'NONE', *, *, #13801, .T. ) ;
#1115=DIRECTION ( 'NONE',  ( -0.1196152422706611984, 0.9928203230275510771, 0.000000000000000000 ) ) ;
#1119=FILL_AREA_STYLE ('',( #13542 ) ) ;
#1120=CARTESIAN_POINT ( 'NONE',  ( 32.81641299864316608, -4.083119185552795294, -7.939653947423662039 ) ) ;
#1122=CARTESIAN_POINT ( 'NONE',  ( 27.10304229683147526, -4.771467524953526329, -3.283357778048664688 ) ) ;
#1123=FACE_BOUND ( 'NONE', #12437, .T. ) ;
#1131=DIRECTION ( 'NONE',  ( -0.5999999999999999778, 0.7999999999999999334, -0.000000000000000000 ) ) ;
#1137=CARTESIAN_POINT ( 'NONE',  ( 13.00000000000000178, 0.000000000000000000, -6.000000000000000000 ) ) ;
#1138=EDGE_CURVE ( 'NONE', #9324, #12386, #9302, .T. ) ;
#1139=EDGE_LOOP ( 'NONE', ( #14257, #12890, #1424, #3754, #13267, #12091 ) ) ;
#1140=CARTESIAN_POINT ( 'NONE',  ( 32.87199790123699472, -1.558343308739095656, -5.783357778048663356 ) ) ;
#1141=EDGE_CURVE ( 'NONE', #11286, #5484, #11940, .T. ) ;
#1142=CARTESIAN_POINT ( 'NONE',  ( 29.14753769709988518, -3.271205139184214516, -3.627061608673662008 ) ) ;
#1145=DIRECTION ( 'NONE',  ( -0.000000000000000000, -0.000000000000000000, 1.000000000000000000 ) ) ;
#1157=ADVANCED_FACE ( 'NONE', ( #14513 ), #7792, .T. ) ;
#1161=VERTEX_POINT ( 'NONE', #7972 ) ;
#1168=CARTESIAN_POINT ( 'NONE',  ( 29.39961944441754227, -3.040961747597316744, -3.283357778048662023 ) ) ;
#1175=CARTESIAN_POINT ( 'NONE',  ( 23.43390247958827288, -9.970148115950962620, -14.83177094038517652 ) ) ;
#1178=CARTESIAN_POINT ( 'NONE',  ( 33.13163345120441505, -4.045141346131868154, -3.627061608673664672 ) ) ;
#1181=AXIS2_PLACEMENT_3D ( 'NONE', #7932, #13466, #1041 ) ;
#1185=CIRCLE ( 'NONE', #14801, 2.749999999999991118 ) ;
#1189=CARTESIAN_POINT ( 'NONE',  ( 28.14933959732260149, -3.391468297350500372, -7.939653947423660263 ) ) ;
#1191=CARTESIAN_POINT ( 'NONE',  ( -45.50000000000000000, -16.03270077640482683, -8.287981825772238409 ) ) ;
#1194=EDGE_CURVE ( 'NONE', #17090, #11418, #15122, .T. ) ;
#1195=DIRECTION ( 'NONE',  ( 0.000000000000000000, 0.000000000000000000, 1.000000000000000000 ) ) ;
#1196=CARTESIAN_POINT ( 'NONE',  ( 29.07687923786957285, -2.352938776424351008, -7.033357778048658027 ) ) ;
#1201=CARTESIAN_POINT ( 'NONE',  ( 30.49166216014303643, -4.363205751385915931, -8.283357778048662468 ) ) ;
#1202=CARTESIAN_POINT ( 'NONE',  ( 27.90727577511918867, -2.156494279411373061, -5.783357778048670461 ) ) ;
#1203=( BOUNDED_CURVE ( )  B_SPLINE_CURVE ( 2, ( #13490, #8126, #10907, #3786, #6418, #7870, #10825, #15012, #6769 ),
 .UNSPECIFIED., .F., .T. ) 
 B_SPLINE_CURVE_WITH_KNOTS ( ( 3, 2, 2, 2, 3 ),
 ( 0.6730769230769231282, 0.6794871794871795156, 0.6923076923076922906, 0.7051282051282051766, 0.7115384615384615641 ),
 .UNSPECIFIED. ) 
 CURVE ( )  GEOMETRIC_REPRESENTATION_ITEM ( )  RATIONAL_B_SPLINE_CURVE ( ( 0.9330127018922192983, 0.9330127018922198534, 1.000000000000000000, 0.8660254037844387076, 1.000000000000000000, 0.8660254037844387076, 1.000000000000000000, 0.9330127018922194093, 0.9330127018922194093 ) ) 
 REPRESENTATION_ITEM ( '' )  );
#1207=AXIS2_PLACEMENT_3D ( 'NONE', #15325, #4498, #15560 ) ;
#1217=CARTESIAN_POINT ( 'NONE',  ( 29.15206445563513071, -6.405512418264540209, -6.861505862736167138 ) ) ;
#1218=DIRECTION ( 'NONE',  ( 0.9928203230275511881, 0.1196152422706614898, 0.000000000000000000 ) ) ;
#1220=CIRCLE ( 'NONE', #12162, 25.00000000000000000 ) ;
#1221=CARTESIAN_POINT ( 'NONE',  ( 26.00347982711925710, -2.723222710571018279, -7.033357778048658027 ) ) ;
#1228=ORIENTED_EDGE ( 'NONE', *, *, #11996, .F. ) ;
#1233=ORIENTED_EDGE ( 'NONE', *, *, #16362, .F. ) ;
#1238=CARTESIAN_POINT ( 'NONE',  ( 9.099998387031005720, -19.29508120620799971, -16.81964500401478091 ) ) ;
#1239=CARTESIAN_POINT ( 'NONE',  ( 29.34898802046944155, -4.500875419183088866, -3.627061608673664672 ) ) ;
#1241=DIRECTION ( 'NONE',  ( -0.8243186046180107640, -0.5661261679878573094, 0.000000000000000000 ) ) ;
#1242=CIRCLE ( 'NONE', #15137, 2.749999999999991118 ) ;
#1245=LINE ( 'NONE', #16555, #5173 ) ;
#1249=CARTESIAN_POINT ( 'NONE',  ( -3.538288549924106796, -15.34800872113743431, -13.00000000000000178 ) ) ;
#1251=AXIS2_PLACEMENT_3D ( 'NONE', #8210, #8025, #13562 ) ;
#1253=ADVANCED_FACE ( 'NONE', ( #5403 ), #4162, .T. ) ;
#1255=ORIENTED_EDGE ( 'NONE', *, *, #3739, .F. ) ;
#1259=VERTEX_POINT ( 'NONE', #14780 ) ;
#1265=DIRECTION ( 'NONE',  ( -1.000000000000000000, 0.000000000000000000, 0.000000000000000000 ) ) ;
#1268=EDGE_CURVE ( 'NONE', #4798, #16432, #724, .T. ) ;
#1269=CARTESIAN_POINT ( 'NONE',  ( 27.95350797341489368, -12.38528642892598342, -13.73189064827997541 ) ) ;
#1272=CARTESIAN_POINT ( 'NONE',  ( 32.82963640218302004, -5.962437625020304388, -4.705209693361169343 ) ) ;
#1274=VERTEX_POINT ( 'NONE', #13589 ) ;
#1279=CARTESIAN_POINT ( 'NONE',  ( 28.34209327568754944, -5.876127416962207306, -7.939653947423662927 ) ) ;
#1280=CARTESIAN_POINT ( 'NONE',  ( 25.80685721358263152, -3.162108319002908896, -4.519686641326834398 ) ) ;
#1281=DIRECTION ( 'NONE',  ( 0.000000000000000000, 0.000000000000000000, -1.000000000000000000 ) ) ;
#1284=CARTESIAN_POINT ( 'NONE',  ( -5.499998387031001634, -20.49508120620799900, -6.000000000000000000 ) ) ;
#1286=ADVANCED_FACE ( 'NONE', ( #5143 ), #13418, .F. ) ;
#1287=CARTESIAN_POINT ( 'NONE',  ( 29.32081432955537892, -3.050456207659999475, -3.283357778048662023 ) ) ;
#1292=CARTESIAN_POINT ( 'NONE',  ( 26.01652455409633902, -4.902371455920928156, -5.783357778048663356 ) ) ;
#1293=ORIENTED_EDGE ( 'NONE', *, *, #12859, .F. ) ;
#1298=VERTEX_POINT ( 'NONE', #3975 ) ;
#1299=FACE_OUTER_BOUND ( 'NONE', #12715, .T. ) ;
#1301=CARTESIAN_POINT ( 'NONE',  ( 29.13014440709066832, -5.781182818409868140, -7.939653947423662927 ) ) ;
#1306=CARTESIAN_POINT ( 'NONE',  ( 25.63782166807609997, -6.407846580969937200, -7.820349034508990549 ) ) ;
#1316=CARTESIAN_POINT ( 'NONE',  ( 32.46178999037268653, -4.125844254797621957, -8.283357778048662468 ) ) ;
#1319=VERTEX_POINT ( 'NONE', #11722 ) ;
#1320=CARTESIAN_POINT ( 'NONE',  ( 30.80679339554874119, -2.444327062417882779, -6.861505862736158257 ) ) ;
#1322=DIRECTION ( 'NONE',  ( 1.000000000000000000, 0.000000000000000000, 0.000000000000000000 ) ) ;
#1327=DIRECTION ( 'NONE',  ( 0.9928203230275510771, 0.1196152422706614621, -0.000000000000000000 ) ) ;
#1328=CARTESIAN_POINT ( 'NONE',  ( 26.24741491880506672, -3.420740141806666301, -3.283357778048662023 ) ) ;
#1330=VERTEX_POINT ( 'NONE', #12825 ) ;
#1331=EDGE_LOOP ( 'NONE', ( #7762, #3457, #12304, #16903, #9576 ) ) ;
#1333=ADVANCED_FACE ( 'NONE', ( #8924 ), #14465, .F. ) ;
#1336=VERTEX_POINT ( 'NONE', #17292 ) ;
#1340=DIRECTION ( 'NONE',  ( -0.1196152422706611984, 0.9928203230275510771, 0.000000000000000000 ) ) ;
#1348=CARTESIAN_POINT ( 'NONE',  ( 29.78250536075762867, -6.329556739422670830, -6.861505862736167138 ) ) ;
#1351=CARTESIAN_POINT ( 'NONE',  ( 26.01652455409633902, -4.902371455920928156, -5.783357778048663356 ) ) ;
#1353=ORIENTED_EDGE ( 'NONE', *, *, #11046, .T. ) ;
#1358=CARTESIAN_POINT ( 'NONE',  ( 29.01637427789896151, -7.048830937829682064, -5.783357778048668685 ) ) ;
#1367=CARTESIAN_POINT ( 'NONE',  ( 28.12379965168153362, -6.829206799398704675, -7.033357778048666908 ) ) ;
#1370=CARTESIAN_POINT ( 'NONE',  ( 30.15026255541241440, -6.285249260098253465, -4.705209693361168455 ) ) ;
#1371=CARTESIAN_POINT ( 'NONE',  ( 36.27615609941022257, -23.17738945083361557, -11.07596365154449636 ) ) ;
#1375=AXIS2_PLACEMENT_3D ( 'NONE', #3181, #1841, #8814 ) ;
#1377=VERTEX_POINT ( 'NONE', #4564 ) ;
#1383=DIRECTION ( 'NONE',  ( 0.000000000000000000, -1.000000000000000000, -3.469446951953614189E-16 ) ) ;
#1387=CARTESIAN_POINT ( 'NONE',  ( 31.65190802758064592, -5.477360103042387074, -7.939653947423662927 ) ) ;
#1390=CARTESIAN_POINT ( 'NONE',  ( 26.20620856698912604, -7.060238655668615415, -4.533357778048668685 ) ) ;
#1400=LINE ( 'NONE', #9630, #8117 ) ;
#1402=ORIENTED_EDGE ( 'NONE', *, *, #10595, .F. ) ;
#1406=CARTESIAN_POINT ( 'NONE',  ( 32.90015225647083952, -1.554951264938056132, -5.113484796970854340 ) ) ;
#1407=CARTESIAN_POINT ( 'NONE',  ( 31.67382807612511542, -6.101689702897060030, -6.861505862736167138 ) ) ;
#1412=CARTESIAN_POINT ( 'NONE',  ( 34.91600907648203389, -11.88801210197604341, 0.000000000000000000 ) ) ;
#1417=VECTOR ( 'NONE', #15217, 1000.000000000000000 ) ;
#1419=AXIS2_PLACEMENT_3D ( 'NONE', #3389, #11806, #15730 ) ;
#1420=EDGE_CURVE ( 'NONE', #963, #1502, #1958, .T. ) ;
#1423=CARTESIAN_POINT ( 'NONE',  ( -45.50000000000000000, -16.03270077640482683, -2.787981825772262390 ) ) ;
#1424=ORIENTED_EDGE ( 'NONE', *, *, #11515, .F. ) ;
#1427=CYLINDRICAL_SURFACE ( 'NONE', #8088, 2.499999999999999112 ) ;
#1433=EDGE_CURVE ( 'NONE', #7967, #2890, #1775, .T. ) ;
#1436=CARTESIAN_POINT ( 'NONE',  ( 16.96391960790757736, -14.58372395263535282, -16.00480323547922978 ) ) ;
#1439=CARTESIAN_POINT ( 'NONE',  ( 28.39010325924584421, -2.735490497978389612, -4.705209693361160461 ) ) ;
#1441=DIRECTION ( 'NONE',  ( 0.000000000000000000, 0.000000000000000000, -1.000000000000000000 ) ) ;
#1446=EDGE_LOOP ( 'NONE', ( #9533, #453, #14937, #5270 ) ) ;
#1448=CARTESIAN_POINT ( 'NONE',  ( 28.45891156537951971, -2.090033060632186412, -5.783357778048670461 ) ) ;
#1449=DIRECTION ( 'NONE',  ( -0.8243186046180107640, 0.5661261679878573094, 0.000000000000000000 ) ) ;
#1451=CARTESIAN_POINT ( 'NONE',  ( 25.85239768453567066, -3.540099486550932983, -4.114102314938801186 ) ) ;
#1456=CARTESIAN_POINT ( 'NONE',  ( 30.04891049036066164, -7.324175753722694360, -5.783357778048669573 ) ) ;
#1459=EDGE_CURVE ( 'NONE', #8286, #11901, #12912, .T. ) ;
#1460=CARTESIAN_POINT ( 'NONE',  ( 29.38830135902312080, -2.615227339812091767, -6.861505862736159145 ) ) ;
#1462=PLANE ( 'NONE',  #17617 ) ;
#1463=DIRECTION ( 'NONE',  ( -0.000000000000000000, -1.000000000000000000, -0.000000000000000000 ) ) ;
#1474=CARTESIAN_POINT ( 'NONE',  ( -21.42089235853292806, -10.15736413759261048, -15.24668633003922658 ) ) ;
#1477=CARTESIAN_POINT ( 'NONE',  ( 29.55043834383900148, -5.730545699181964991, -3.627061608673668225 ) ) ;
#1478=DIRECTION ( 'NONE',  ( 1.000000000000000000, 0.000000000000000000, 0.000000000000000000 ) ) ;
#1482=CARTESIAN_POINT ( 'NONE',  ( 31.28415083292585663, -5.521667582366822202, -3.627061608673667781 ) ) ;
#1484=EDGE_CURVE ( 'NONE', #16203, #1319, #11637, .T. ) ;
#1489=CARTESIAN_POINT ( 'NONE',  ( 21.42986351335030548, -22.27113001973728146, -15.24426822127429659 ) ) ;
#1492=AXIS2_PLACEMENT_3D ( 'NONE', #7438, #13143, #12958 ) ;
#1496=AXIS2_PLACEMENT_3D ( 'NONE', #7257, #16878, #15316 ) ;
#1497=VERTEX_POINT ( 'NONE', #10357 ) ;
#1499=CARTESIAN_POINT ( 'NONE',  ( 32.29220775574281532, -1.628196571319322050, -6.453230759126467042 ) ) ;
#1502=VERTEX_POINT ( 'NONE', #948 ) ;
#1504=CARTESIAN_POINT ( 'NONE',  ( 27.26074174026764751, -6.633379454790151009, -6.861505862736167138 ) ) ;
#1506=CARTESIAN_POINT ( 'NONE',  ( 31.95146207396702565, -5.641142275435198528, -8.283357778048662468 ) ) ;
#1514=CARTESIAN_POINT ( 'NONE',  ( 27.27683486999669427, -2.232449958253242883, -5.783357778048658027 ) ) ;
#1520=CIRCLE ( 'NONE', #12232, 2.749999999999988454 ) ;
#1531=CARTESIAN_POINT ( 'NONE',  ( -34.91600907648203389, -11.88801210197604341, -11.56671555609732671 ) ) ;
#1533=CARTESIAN_POINT ( 'NONE',  ( 27.11150007966593733, -11.49307575575171469, -13.95470972894434780 ) ) ;
#1540=CARTESIAN_POINT ( 'NONE',  ( 29.89119874204131122, -2.254829357712824667, -4.533357778048659803 ) ) ;
#1547=FACE_OUTER_BOUND ( 'NONE', #13456, .T. ) ;
#1548=CARTESIAN_POINT ( 'NONE',  ( 25.75668387115780078, -2.745663783273349257, -5.690028976746116740 ) ) ;
#1549=CARTESIAN_POINT ( 'NONE',  ( -5.499998387031001634, -20.49508120620799900, -13.00000000000000178 ) ) ;
#1554=CARTESIAN_POINT ( 'NONE',  ( 27.38828526237195504, -6.917821758047558056, -4.533357778048668685 ) ) ;
#1557=CARTESIAN_POINT ( 'NONE',  ( 29.64681518302145591, -6.972875258987813574, -5.783357778048668685 ) ) ;
#1559=DIRECTION ( 'NONE',  ( 0.000000000000000000, 3.469446951953614189E-16, -1.000000000000000000 ) ) ;
#1564=ORIENTED_EDGE ( 'NONE', *, *, #1138, .T. ) ;
#1569=EDGE_CURVE ( 'NONE', #1274, #12756, #5097, .T. ) ;
#1571=CARTESIAN_POINT ( 'NONE',  ( -5.499998387031001634, -20.49508120620799900, -12.00000000000000000 ) ) ;
#1573=( BOUNDED_SURFACE ( )  B_SPLINE_SURFACE ( 1, 2, ( 
 ( #12339, #15155, #10777, #3833, #14804, #5258, #13707, #12060, #9430, #14886, #3734, #3917, #2392, #15059, #2472, #13529, #10864, #11981, #10684, #17564, #10605, #16172, #16262, #7908, #13443, #4001, #13616, #9515, #14968, #6813, #1023, #2555, #12256, #5343, #4270, #3174, #12784, #13970, #8, #12518, #15236, #11044, #4530, #8713, #16887, #4185, #188, #16693, #11409, #10048, #2814, #103, #9686, #8528, #16974, #5697, #9771, #8340, #12608, #15509, #6989, #4355, #15324, #16609, #11213, #13873, #9959, #2902, #8433, #5795, #1370, #5611, #5886, #380, #15598, #11126, #1460, #6894, #4449, #3006, #11310, #1557, #3091, #12422, #7090, #5525, #7267, #16787, #9867, #15421, #14060, #1646, #7180, #12689, #282, #8613, #14145, #1735, #17067, #13058, #11596, #6345, #17447, #15694, #12965, #4620, #3450, #4981, #10143, #7629, #10508, #17163, #11868, #8892, #6257, #8979, #17349, #13151, #730, #14523, #11775, #5972, #16069, #4711, #14426, #3543, #3275, #7536, #15784, #3638, #14247, #8808, #2010, #644, #14339, #4886, #10416, #9073, #1925, #15974, #14617, #13236, #7445, #2197, #11496, #2106, #10238, #6167, #11690, #550, #1833, #6067, #3361 ),
 ( #15875, #17260, #7710, #4796, #10318, #813, #7365, #12880, #466, #6608, #13330, #13685, #1178, #9160, #3716, #6444, #13427, #16153, #7977, #17886, #8059, #2532, #1272, #5324, #6792, #6697, #14699, #9240, #11962, #1005, #14786, #13513, #5414, #13596, #12234, #12320, #10848, #2375, #16416, #3981, #17806, #17546, #10929, #6530, #14952, #16495, #5066, #2281, #7799, #10668, #12044, #7892, #1083, #17631, #5149, #910, #9497, #10586, #8153, #12138, #17717, #3814, #16242, #15037, #3896, #9329, #5239, #14868, #2457, #10759, #16337, #9413, #2626, #11453, #11361, #15549, #4168, #16931, #6871, #424, #1348, #4067, #13850, #3130, #5839, #15215, #12734, #9667, #4489, #2718, #2795, #10095, #8239, #8320, #331, #11023, #8664, #14192, #1439, #17020, #10003, #11779, #4574, #13771, #5929, #1785, #12402, #9577, #5501, #6966, #7316, #12836, #16586, #15132, #16238, #1081, #566, #14263, #15713, #13423, #5146, #14865, #3711, #9235, #8731, #10665, #13328, #905, #5988, #10251, #5234, #1853, #11514, #10163, #10583, #1002, #10755, #17628, #6527, #16150, #12135, #5063, #14444, #12041, #8908, #3291, #479, #11615, #17180, #6439, #11960, #7381, #6087 ) ),
 .UNSPECIFIED., .F., .F., .T. ) 
 B_SPLINE_SURFACE_WITH_KNOTS ( ( 2, 2 ),
 ( 3, 2, 2, 2, 2, 2, 2, 2, 2, 2, 2, 2, 2, 2, 2, 2, 2, 2, 2, 2, 2, 2, 2, 2, 2, 2, 2, 2, 2, 2, 2, 2, 2, 2, 2, 2, 2, 2, 2, 2, 2, 2, 2, 2, 2, 2, 2, 2, 2, 2, 2, 2, 2, 2, 2, 2, 2, 2, 2, 2, 2, 2, 2, 2, 2, 2, 2, 2, 2, 2, 2, 2, 2, 2, 2, 2, 3 ),
 ( 0.000000000000000000, 1.000000000000000000 ),
 ( 0.000000000000000000, 0.01282051282051282007, 0.02564102564102564014, 0.03846153846153846367, 0.05128205128205128027, 0.06410256410256409687, 0.07692307692307692735, 0.08974358974358974395, 0.1025641025641025605, 0.1153846153846153910, 0.1282051282051281937, 0.1410256410256410242, 0.1538461538461538547, 0.1666666666666666574, 0.1794871794871794879, 0.1923076923076923184, 0.2051282051282051211, 0.2179487179487179516, 0.2307692307692307820, 0.2435897435897435848, 0.2564102564102563875, 0.2692307692307692180, 0.2820512820512820484, 0.2948717948717948789, 0.3076923076923077094, 0.3205128205128205399, 0.3333333333333333148, 0.3461538461538461453, 0.3589743589743589758, 0.3717948717948718063, 0.3846153846153846367, 0.3974358974358974117, 0.4102564102564102422, 0.4230769230769230727, 0.4358974358974359031, 0.4487179487179487336, 0.4615384615384615641, 0.4743589743589743390, 0.4871794871794871695, 0.5000000000000000000, 0.5128205128205127750, 0.5256410256410256610, 0.5384615384615384359, 0.5512820512820513219, 0.5641025641025640969, 0.5769230769230768718, 0.5897435897435897578, 0.6025641025641025328, 0.6153846153846154188, 0.6282051282051281937, 0.6410256410256410797, 0.6538461538461538547, 0.6666666666666666297, 0.6794871794871795156, 0.6923076923076922906, 0.7051282051282051766, 0.7179487179487179516, 0.7307692307692307265, 0.7435897435897436125, 0.7564102564102563875, 0.7692307692307692735, 0.7820512820512820484, 0.7948717948717948234, 0.8076923076923077094, 0.8205128205128204844, 0.8333333333333333703, 0.8461538461538461453, 0.8589743589743589203, 0.8717948717948718063, 0.8846153846153845812, 0.8974358974358974672, 0.9102564102564102422, 0.9230769230769231282, 0.9358974358974359031, 0.9487179487179486781, 0.9615384615384615641, 0.9690838366659333403 ),
 .UNSPECIFIED. ) 
 GEOMETRIC_REPRESENTATION_ITEM ( )  RATIONAL_B_SPLINE_SURFACE ( (
 ( 1.000000000000000000, 0.8660254037844387076, 1.000000000000000000, 0.8660254037844387076, 1.000000000000000000, 0.8660254037844387076, 1.000000000000000000, 0.8660254037844387076, 1.000000000000000000, 0.8660254037844387076, 1.000000000000000000, 0.8660254037844387076, 1.000000000000000000, 0.8660254037844387076, 1.000000000000000000, 0.8660254037844387076, 1.000000000000000000, 0.8660254037844387076, 1.000000000000000000, 0.8660254037844387076, 1.000000000000000000, 0.8660254037844387076, 1.000000000000000000, 0.8660254037844387076, 1.000000000000000000, 0.8660254037844387076, 1.000000000000000000, 0.8660254037844387076, 1.000000000000000000, 0.8660254037844387076, 1.000000000000000000, 0.8660254037844387076, 1.000000000000000000, 0.8660254037844387076, 1.000000000000000000, 0.8660254037844387076, 1.000000000000000000, 0.8660254037844387076, 1.000000000000000000, 0.8660254037844387076, 1.000000000000000000, 0.8660254037844387076, 1.000000000000000000, 0.8660254037844387076, 1.000000000000000000, 0.8660254037844387076, 1.000000000000000000, 0.8660254037844387076, 1.000000000000000000, 0.8660254037844387076, 1.000000000000000000, 0.8660254037844387076, 1.000000000000000000, 0.8660254037844387076, 1.000000000000000000, 0.8660254037844387076, 1.000000000000000000, 0.8660254037844387076, 1.000000000000000000, 0.8660254037844387076, 1.000000000000000000, 0.8660254037844387076, 1.000000000000000000, 0.8660254037844387076, 1.000000000000000000, 0.8660254037844387076, 1.000000000000000000, 0.8660254037844387076, 1.000000000000000000, 0.8660254037844387076, 1.000000000000000000, 0.8660254037844387076, 1.000000000000000000, 0.8660254037844387076, 1.000000000000000000, 0.8660254037844387076, 1.000000000000000000, 0.8660254037844387076, 1.000000000000000000, 0.8660254037844387076, 1.000000000000000000, 0.8660254037844387076, 1.000000000000000000, 0.8660254037844387076, 1.000000000000000000, 0.8660254037844387076, 1.000000000000000000, 0.8660254037844387076, 1.000000000000000000, 0.8660254037844387076, 1.000000000000000000, 0.8660254037844387076, 1.000000000000000000, 0.8660254037844387076, 1.000000000000000000, 0.8660254037844387076, 1.000000000000000000, 0.8660254037844387076, 1.000000000000000000, 0.8660254037844387076, 1.000000000000000000, 0.8660254037844387076, 1.000000000000000000, 0.8660254037844387076, 1.000000000000000000, 0.8660254037844387076, 1.000000000000000000, 0.8660254037844387076, 1.000000000000000000, 0.8660254037844387076, 1.000000000000000000, 0.8660254037844387076, 1.000000000000000000, 0.8660254037844387076, 1.000000000000000000, 0.8660254037844387076, 1.000000000000000000, 0.8660254037844387076, 1.000000000000000000, 0.8660254037844387076, 1.000000000000000000, 0.8660254037844387076, 1.000000000000000000, 0.8660254037844387076, 1.000000000000000000, 0.8660254037844387076, 1.000000000000000000, 0.8660254037844387076, 1.000000000000000000, 0.8660254037844387076, 1.000000000000000000, 0.8660254037844387076, 1.000000000000000000, 0.8660254037844387076, 1.000000000000000000, 0.8660254037844387076, 1.000000000000000000, 0.8660254037844387076, 1.000000000000000000, 0.8660254037844387076, 1.000000000000000000, 0.8660254037844387076, 1.000000000000000000, 0.8660254037844387076, 1.000000000000000000, 0.8660254037844387076, 1.000000000000000000, 0.8660254037844387076, 1.000000000000000000, 0.8660254037844387076, 1.000000000000000000, 0.9211506902921580142, 0.9351132093492240394),
 ( 1.000000000000000000, 0.8660254037844387076, 1.000000000000000000, 0.8660254037844387076, 1.000000000000000000, 0.8660254037844387076, 1.000000000000000000, 0.8660254037844387076, 1.000000000000000000, 0.8660254037844387076, 1.000000000000000000, 0.8660254037844387076, 1.000000000000000000, 0.8660254037844387076, 1.000000000000000000, 0.8660254037844387076, 1.000000000000000000, 0.8660254037844387076, 1.000000000000000000, 0.8660254037844387076, 1.000000000000000000, 0.8660254037844387076, 1.000000000000000000, 0.8660254037844387076, 1.000000000000000000, 0.8660254037844387076, 1.000000000000000000, 0.8660254037844387076, 1.000000000000000000, 0.8660254037844387076, 1.000000000000000000, 0.8660254037844387076, 1.000000000000000000, 0.8660254037844387076, 1.000000000000000000, 0.8660254037844387076, 1.000000000000000000, 0.8660254037844387076, 1.000000000000000000, 0.8660254037844387076, 1.000000000000000000, 0.8660254037844387076, 1.000000000000000000, 0.8660254037844387076, 1.000000000000000000, 0.8660254037844387076, 1.000000000000000000, 0.8660254037844387076, 1.000000000000000000, 0.8660254037844387076, 1.000000000000000000, 0.8660254037844387076, 1.000000000000000000, 0.8660254037844387076, 1.000000000000000000, 0.8660254037844387076, 1.000000000000000000, 0.8660254037844387076, 1.000000000000000000, 0.8660254037844387076, 1.000000000000000000, 0.8660254037844387076, 1.000000000000000000, 0.8660254037844387076, 1.000000000000000000, 0.8660254037844387076, 1.000000000000000000, 0.8660254037844387076, 1.000000000000000000, 0.8660254037844387076, 1.000000000000000000, 0.8660254037844387076, 1.000000000000000000, 0.8660254037844387076, 1.000000000000000000, 0.8660254037844387076, 1.000000000000000000, 0.8660254037844387076, 1.000000000000000000, 0.8660254037844387076, 1.000000000000000000, 0.8660254037844387076, 1.000000000000000000, 0.8660254037844387076, 1.000000000000000000, 0.8660254037844387076, 1.000000000000000000, 0.8660254037844387076, 1.000000000000000000, 0.8660254037844387076, 1.000000000000000000, 0.8660254037844387076, 1.000000000000000000, 0.8660254037844387076, 1.000000000000000000, 0.8660254037844387076, 1.000000000000000000, 0.8660254037844387076, 1.000000000000000000, 0.8660254037844387076, 1.000000000000000000, 0.8660254037844387076, 1.000000000000000000, 0.8660254037844387076, 1.000000000000000000, 0.8660254037844387076, 1.000000000000000000, 0.8660254037844387076, 1.000000000000000000, 0.8660254037844387076, 1.000000000000000000, 0.8660254037844387076, 1.000000000000000000, 0.8660254037844387076, 1.000000000000000000, 0.8660254037844387076, 1.000000000000000000, 0.8660254037844387076, 1.000000000000000000, 0.8660254037844387076, 1.000000000000000000, 0.8660254037844387076, 1.000000000000000000, 0.8660254037844387076, 1.000000000000000000, 0.8660254037844387076, 1.000000000000000000, 0.8660254037844387076, 1.000000000000000000, 0.8660254037844387076, 1.000000000000000000, 0.8660254037844387076, 1.000000000000000000, 0.8660254037844387076, 1.000000000000000000, 0.8660254037844387076, 1.000000000000000000, 0.8660254037844387076, 1.000000000000000000, 0.8660254037844387076, 1.000000000000000000, 0.8660254037844387076, 1.000000000000000000, 0.8660254037844387076, 1.000000000000000000, 0.8660254037844387076, 1.000000000000000000, 0.8660254037844387076, 1.000000000000000000, 0.8660254037844387076, 1.000000000000000000, 0.9211506902921580142, 0.9351132093492240394) ) ) 
 REPRESENTATION_ITEM ( '' )  SURFACE ( )  );
#1574=CARTESIAN_POINT ( 'NONE',  ( 30.80679339554874119, -2.444327062417882779, -6.861505862736158257 ) ) ;
#1577=EDGE_LOOP ( 'NONE', ( #14715, #6873, #14999, #11550, #16139 ) ) ;
#1578=CARTESIAN_POINT ( 'NONE',  ( 30.23341599105502908, -5.648260380436597394, -7.939653947423664704 ) ) ;
#1579=CYLINDRICAL_SURFACE ( 'NONE', #8368, 2.499999999999999112 ) ;
#1585=EDGE_CURVE ( 'NONE', #2866, #3447, #17811, .T. ) ;
#1590=CARTESIAN_POINT ( 'NONE',  ( 26.30109267735093681, -7.264319738512599933, -6.611283024552371934 ) ) ;
#1592=PLANE ( 'NONE',  #14781 ) ;
#1597=CARTESIAN_POINT ( 'NONE',  ( 26.49878054387835746, -2.963357534503999968, -4.705209693361160461 ) ) ;
#1598=CARTESIAN_POINT ( 'NONE',  ( 32.58190297908952004, -5.565186596593329149, -8.283357778048662468 ) ) ;
#1606=CARTESIAN_POINT ( 'NONE',  ( -45.50000000000000000, -16.03270077640482683, -5.537981825772250843 ) ) ;
#1608=( BOUNDED_CURVE ( )  B_SPLINE_CURVE ( 3, ( #6366, #5085, #11796, #10685 ),
 .UNSPECIFIED., .F., .T. ) 
 B_SPLINE_CURVE_WITH_KNOTS ( ( 4, 4 ),
 ( 3.141592653589793116, 6.283185307179586232 ),
 .UNSPECIFIED. ) 
 CURVE ( )  GEOMETRIC_REPRESENTATION_ITEM ( )  RATIONAL_B_SPLINE_CURVE ( ( 1.000000000000000000, 0.3333333333333333703, 0.3333333333333333703, 1.000000000000000000 ) ) 
 REPRESENTATION_ITEM ( '' )  );
#1609=VERTEX_POINT ( 'NONE', #5715 ) ;
#1614=DIRECTION ( 'NONE',  ( 0.000000000000000000, 1.000000000000000000, -0.000000000000000000 ) ) ;
#1618=LINE ( 'NONE', #2973, #11821 ) ;
#1621=DIRECTION ( 'NONE',  ( 0.9928203230275512992, 0.1196152422706614898, -0.000000000000000000 ) ) ;
#1625=CARTESIAN_POINT ( 'NONE',  ( -9.099998387031005720, -19.29508120620799971, -6.000000000000000000 ) ) ;
#1628=ORIENTED_EDGE ( 'NONE', *, *, #11996, .T. ) ;
#1630=LINE ( 'NONE', #7346, #7510 ) ;
#1631=EDGE_LOOP ( 'NONE', ( #11424, #1747, #3079, #10057 ) ) ;
#1632=ORIENTED_EDGE ( 'NONE', *, *, #12695, .T. ) ;
#1636=CARTESIAN_POINT ( 'NONE',  ( 26.21417678486618641, -2.370676134166772808, -5.783357778048658915 ) ) ;
#1639=DIRECTION ( 'NONE',  ( 0.7999999999999999334, 0.6000000000000000888, -0.000000000000000000 ) ) ;
#1646=CARTESIAN_POINT ( 'NONE',  ( 28.97253418081003673, -5.800171738120336151, -7.939653947423664704 ) ) ;
#1653=VERTEX_POINT ( 'NONE', #15613 ) ;
#1654=CARTESIAN_POINT ( 'NONE',  ( 16.75000000000000000, -16.21813761408365195, -13.00000000000000178 ) ) ;
#1656=EDGE_CURVE ( 'NONE', #12969, #2761, #3193, .T. ) ;
#1658=DIRECTION ( 'NONE',  ( -1.000000000000000000, 0.000000000000000000, 0.000000000000000000 ) ) ;
#1660=CARTESIAN_POINT ( 'NONE',  ( 28.98992747081926069, -3.290194058894681639, -3.627061608673662896 ) ) ;
#1661=CARTESIAN_POINT ( 'NONE',  ( 26.82722439997946395, -4.804698134550569044, -3.627061608673664672 ) ) ;
#1663=AXIS2_PLACEMENT_3D ( 'NONE', #7669, #2236, #10710 ) ;
#1664=CARTESIAN_POINT ( 'NONE',  ( 30.13703915187255689, -4.405930820630744371, -7.939653947423662039 ) ) ;
#1669=CARTESIAN_POINT ( 'NONE',  ( 29.91004888286193619, -6.613999042680076990, -4.533357778048668685 ) ) ;
#1670=VERTEX_POINT ( 'NONE', #7725 ) ;
#1680=DIRECTION ( 'NONE',  ( 0.000000000000000000, 1.000000000000000000, 0.000000000000000000 ) ) ;
#1682=CARTESIAN_POINT ( 'NONE',  ( 26.67454832010805532, -2.305013593294074514, -5.113484796970851676 ) ) ;
#1683=CARTESIAN_POINT ( 'NONE',  ( 33.83155592109562804, -6.868441680671474536, -5.783357778048669573 ) ) ;
#1684=CARTESIAN_POINT ( 'NONE',  ( 32.61569110240115776, -6.288022587442930522, -7.033357778048666908 ) ) ;
#1687=DIRECTION ( 'NONE',  ( 0.000000000000000000, 0.000000000000000000, 1.000000000000000000 ) ) ;
#1692=VECTOR ( 'NONE', #7368, 1000.000000000000000 ) ;
#1695=( BOUNDED_CURVE ( )  B_SPLINE_CURVE ( 2, ( #5317, #3629, #900, #16145, #10750, #2522, #17878, #6688, #12221 ),
 .UNSPECIFIED., .F., .T. ) 
 B_SPLINE_CURVE_WITH_KNOTS ( ( 3, 2, 2, 2, 3 ),
 ( 0.7115384615384615641, 0.7179487179487179516, 0.7307692307692307265, 0.7435897435897436125, 0.7500000000000000000 ),
 .UNSPECIFIED. ) 
 CURVE ( )  GEOMETRIC_REPRESENTATION_ITEM ( )  RATIONAL_B_SPLINE_CURVE ( ( 0.9330127018922194093, 0.9330127018922194093, 1.000000000000000000, 0.8660254037844387076, 1.000000000000000000, 0.8660254037844387076, 1.000000000000000000, 0.9330127018922194093, 0.9330127018922194093 ) ) 
 REPRESENTATION_ITEM ( '' )  );
#1704=DIRECTION ( 'NONE',  ( 0.9899494936611662466, 0.1414213562373111965, 0.000000000000000000 ) ) ;
#1705=CARTESIAN_POINT ( 'NONE',  ( -50.00000000000000000, -19.03270077640483038, -5.537981825772250843 ) ) ;
#1714=CONICAL_SURFACE ( 'NONE', #17075, 3.999999999999986677, 0.7853981633974400633 ) ;
#1716=EDGE_CURVE ( 'NONE', #17066, #14839, #5080, .T. ) ;
#1724=LINE ( 'NONE', #7254, #3871 ) ;
#1729=CARTESIAN_POINT ( 'NONE',  ( 31.29094215978502902, -2.813094711071706389, -3.283357778048662023 ) ) ;
#1730=DIRECTION ( 'NONE',  ( 0.000000000000000000, 0.000000000000000000, -1.000000000000000000 ) ) ;
#1735=CARTESIAN_POINT ( 'NONE',  ( 28.35948656569675919, -3.366149737736551906, -3.627061608673662896 ) ) ;
#1737=CARTESIAN_POINT ( 'NONE',  ( 32.34851646621051202, -1.621412483717243447, -5.113484796970854340 ) ) ;
#1747=ORIENTED_EDGE ( 'NONE', *, *, #9946, .T. ) ;
#1750=CARTESIAN_POINT ( 'NONE',  ( 45.50000000000000000, -19.03270077640483038, -5.537981825772250843 ) ) ;
#1751=ORIENTED_EDGE ( 'NONE', *, *, #14289, .F. ) ;
#1752=CARTESIAN_POINT ( 'NONE',  ( -19.91444112663254984, -10.77903654349075246, -15.52697452096630748 ) ) ;
#1753=ORIENTED_EDGE ( 'NONE', *, *, #14588, .F. ) ;
#1755=CARTESIAN_POINT ( 'NONE',  ( 27.02414796481377124, -2.900061135469103490, -6.861505862736158257 ) ) ;
#1756=CARTESIAN_POINT ( 'NONE',  ( 31.93198502805756789, -2.935734224299280548, -7.939653947423660263 ) ) ;
#1759=DIRECTION ( 'NONE',  ( -1.000000000000000000, 0.000000000000000000, -0.000000000000000000 ) ) ;
#1761=EDGE_CURVE ( 'NONE', #6497, #8021, #12796, .T. ) ;
#1767=EDGE_CURVE ( 'NONE', #2633, #13499, #4683, .T. ) ;
#1770=CARTESIAN_POINT ( 'NONE',  ( 2.749999999999992895, -20.49999999999999645, -6.000000000000000000 ) ) ;
#1773=EDGE_LOOP ( 'NONE', ( #5510, #13248, #5935, #4030 ) ) ;
#1775=LINE ( 'NONE', #11444, #15386 ) ;
#1777=CARTESIAN_POINT ( 'NONE',  ( 26.90793483298705979, -6.248787706170159773, -8.283357778048664244 ) ) ;
#1778=VECTOR ( 'NONE', #16902, 1000.000000000000000 ) ;
#1780=CARTESIAN_POINT ( 'NONE',  ( 26.60838078660069428, -6.085005533777348319, -7.939653947423664704 ) ) ;
#1781=CARTESIAN_POINT ( 'NONE',  ( 31.83134908525019213, -4.201799933639492224, -8.283357778048662468 ) ) ;
#1785=CARTESIAN_POINT ( 'NONE',  ( 28.54354359905709870, -7.105797696961086096, -5.783357778048669573 ) ) ;
#1787=VECTOR ( 'NONE', #1827, 1000.000000000000000 ) ;
#1789=CARTESIAN_POINT ( 'NONE',  ( 20.00000000000000355, 7.999999999999996447, 0.000000000000000000 ) ) ;
#1795=ORIENTED_EDGE ( 'NONE', *, *, #16836, .F. ) ;
#1799=ORIENTED_EDGE ( 'NONE', *, *, #8255, .T. ) ;
#1801=ORIENTED_EDGE ( 'NONE', *, *, #8627, .T. ) ;
#1804=EDGE_CURVE ( 'NONE', #5110, #16117, #13702, .T. ) ;
#1810=AXIS2_PLACEMENT_3D ( 'NONE', #6953, #1621, #1340 ) ;
#1815=CARTESIAN_POINT ( 'NONE',  ( 29.79859849048667897, -1.928627242885762705, -5.783357778048664244 ) ) ;
#1816=VECTOR ( 'NONE', #17366, 1000.000000000000000 ) ;
#1817=ORIENTED_EDGE ( 'NONE', *, *, #14108, .F. ) ;
#1822=FACE_OUTER_BOUND ( 'NONE', #10493, .T. ) ;
#1823=CARTESIAN_POINT ( 'NONE',  ( -19.49912934580633106, 8.667827538924893105, -15.60122950519025409 ) ) ;
#1825=CARTESIAN_POINT ( 'NONE',  ( -28.59532824046058153, -19.01044845393195715, -13.55637998813296186 ) ) ;
#1827=DIRECTION ( 'NONE',  ( -0.000000000000000000, -0.000000000000000000, -1.000000000000000000 ) ) ;
#1829=CIRCLE ( 'NONE', #10767, 2.000000000000001776 ) ;
#1831=CARTESIAN_POINT ( 'NONE',  ( 26.14503574297738098, -5.691300421908874085, -8.283357778048664244 ) ) ;
#1833=CARTESIAN_POINT ( 'NONE',  ( 25.72395281601508898, -4.937620572523835349, -7.939653947423662039 ) ) ;
#1835=DIRECTION ( 'NONE',  ( 0.000000000000000000, 1.000000000000000000, 3.469446951953614189E-16 ) ) ;
#1837=LINE ( 'NONE', #9962, #1692 ) ;
#1841=DIRECTION ( 'NONE',  ( 0.000000000000000000, -0.000000000000000000, 1.000000000000000000 ) ) ;
#1844=ORIENTED_EDGE ( 'NONE', *, *, #1716, .F. ) ;
#1845=VERTEX_POINT ( 'NONE', #6808 ) ;
#1848=CARTESIAN_POINT ( 'NONE',  ( -17.40654580017221065, -13.42197210625884551, -15.93919332483364748 ) ) ;
#1850=EDGE_CURVE ( 'NONE', #16681, #13069, #16352, .T. ) ;
#1852=CARTESIAN_POINT ( 'NONE',  ( 27.89118264539014547, -6.557423775948280742, -6.861505862736167138 ) ) ;
#1853=CARTESIAN_POINT ( 'NONE',  ( 27.02867472334902033, -6.034368414549446058, -3.627061608673668225 ) ) ;
#1854=CARTESIAN_POINT ( 'NONE',  ( 29.60297508593253468, -5.724216059278466773, -7.939653947423664704 ) ) ;
#1856=CARTESIAN_POINT ( 'NONE',  ( 27.80031630502317341, -2.169380783275094426, -6.453230759126464378 ) ) ;
#1870=DIRECTION ( 'NONE',  ( 1.000000000000000000, 0.000000000000000000, -0.000000000000000000 ) ) ;
#1876=CARTESIAN_POINT ( 'NONE',  ( 31.64365984991007252, -1.316785610144591390, -5.783357778048658027 ) ) ;
#1878=ADVANCED_FACE ( 'NONE', ( #2643, #4266 ), #14964, .T. ) ;
#1890=DIRECTION ( 'NONE',  ( 0.000000000000000000, 0.000000000000000000, 1.000000000000000000 ) ) ;
#1891=ORIENTED_EDGE ( 'NONE', *, *, #9946, .F. ) ;
#1892=FACE_OUTER_BOUND ( 'NONE', #9347, .T. ) ;
#1895=CARTESIAN_POINT ( 'NONE',  ( 26.07857582428556853, -4.894895503279006022, -8.283357778048662468 ) ) ;
#1899=EDGE_CURVE ( 'NONE', #11176, #14870, #17899, .T. ) ;
#1908=EDGE_LOOP ( 'NONE', ( #4539, #14023, #8623, #6291 ) ) ;
#1914=CARTESIAN_POINT ( 'NONE',  ( -21.62109127008995557, -22.31747812791595464, -15.20678566061929615 ) ) ;
#1916=EDGE_CURVE ( 'NONE', #2334, #3411, #9512, .T. ) ;
#1917=DIRECTION ( 'NONE',  ( -1.000000000000000000, 0.000000000000000000, 0.000000000000000000 ) ) ;
#1925=CARTESIAN_POINT ( 'NONE',  ( 26.35439372113758694, -4.861664893681965083, -7.939653947423662039 ) ) ;
#1928=DIRECTION ( 'NONE',  ( 0.7999999999999999334, 0.6000000000000001998, -0.000000000000000000 ) ) ;
#1932=ORIENTED_EDGE ( 'NONE', *, *, #640, .T. ) ;
#1939=CARTESIAN_POINT ( 'NONE',  ( 28.28955653359400557, -5.882457056865704637, -3.627061608673668225 ) ) ;
#1941=CARTESIAN_POINT ( 'NONE',  ( 27.60205212784272177, -2.830435096530727446, -4.705209693361161349 ) ) ;
#1943=CARTESIAN_POINT ( 'NONE',  ( 33.79776779778399032, -6.145605689821873163, -7.033357778048666908 ) ) ;
#1952=CARTESIAN_POINT ( 'NONE',  ( -1.917618200156724081E-28, -7.000000000000001776, -17.00000000000000000 ) ) ;
#1954=VERTEX_POINT ( 'NONE', #185 ) ;
#1956=ORIENTED_EDGE ( 'NONE', *, *, #7800, .T. ) ;
#1957=CARTESIAN_POINT ( 'NONE',  ( 3.347071143357317702, -15.22052928361023127, -17.00000000000000000 ) ) ;
#1958=LINE ( 'NONE', #11102, #6988 ) ;
#1959=CARTESIAN_POINT ( 'NONE',  ( 26.78782184427022983, -4.809445364374452581, -8.283357778048662468 ) ) ;
#1960=CARTESIAN_POINT ( 'NONE',  ( 29.35841309260160159, -6.680460261459264970, -4.533357778048668685 ) ) ;
#1961=CARTESIAN_POINT ( 'NONE',  ( -3.248936832696171617, -15.16081378324841111, -17.00000000000000000 ) ) ;
#1963=DIRECTION ( 'NONE',  ( -0.000000000000000000, -0.000000000000000000, 1.000000000000000000 ) ) ;
#1964=CARTESIAN_POINT ( 'NONE',  ( 27.29063000668916672, -2.568146533142987575, -4.533357778048659803 ) ) ;
#1970=ORIENTED_EDGE ( 'NONE', *, *, #11657, .T. ) ;
#1980=CARTESIAN_POINT ( 'NONE',  ( 32.96626681528915981, -4.065064760026301016, -5.783357778048663356 ) ) ;
#1982=VECTOR ( 'NONE', #12816, 1000.000000000000000 ) ;
#1987=AXIS2_PLACEMENT_3D ( 'NONE', #1351, #6533, #17634 ) ;
#1991=ORIENTED_EDGE ( 'NONE', *, *, #15992, .T. ) ;
#1992=CIRCLE ( 'NONE', #6018, 2.749999999999988454 ) ;
#2006=CARTESIAN_POINT ( 'NONE',  ( 25.11802603177690330, -16.03270077640482683, -10.53798182577225084 ) ) ;
#2007=CARTESIAN_POINT ( 'NONE',  ( 30.00264913441657555, -6.940201157507134511, -5.783357778048657138 ) ) ;
#2010=CARTESIAN_POINT ( 'NONE',  ( 26.66961417369883591, -4.823687054261037055, -3.627061608673664672 ) ) ;
#2012=VERTEX_POINT ( 'NONE', #11208 ) ;
#2017=DIRECTION ( 'NONE',  ( -0.9928203230275510771, 0.1196152422706621282, 0.000000000000000000 ) ) ;
#2018=EDGE_LOOP ( 'NONE', ( #2444, #12565, #15569, #11349, #7141 ) ) ;
#2019=CARTESIAN_POINT ( 'NONE',  ( 32.67202617590239555, -5.981426544730773287, -4.705209693361168455 ) ) ;
#2021=AXIS2_PLACEMENT_3D ( 'NONE', #4297, #4559, #14280 ) ;
#2025=CARTESIAN_POINT ( 'NONE',  ( 27.26074174026764751, -6.633379454790151009, -6.861505862736167138 ) ) ;
#2027=CARTESIAN_POINT ( 'NONE',  ( 16.75000000000000000, -16.21813761408365195, -16.03574476417184513 ) ) ;
#2029=CARTESIAN_POINT ( 'NONE',  ( 27.73357241910951743, -6.576412695658750529, -6.861505862736166250 ) ) ;
#2033=AXIS2_PLACEMENT_3D ( 'NONE', #2874, #15205, #8310 ) ;
#2045=CARTESIAN_POINT ( 'NONE',  ( 26.01652455409633902, -4.902371455920928156, -5.783357778048663356 ) ) ;
#2050=CARTESIAN_POINT ( 'NONE',  ( 28.63031693179632242, -2.406740715396564756, -4.533357778048659803 ) ) ;
#2056=( BOUNDED_CURVE ( )  B_SPLINE_CURVE ( 2, ( #622, #2352, #7871, #13307, #14848, #6512, #15946, #7692, #13401 ),
 .UNSPECIFIED., .F., .T. ) 
 B_SPLINE_CURVE_WITH_KNOTS ( ( 3, 2, 2, 2, 3 ),
 ( 0.9038461538461538547, 0.9102564102564102422, 0.9230769230769231282, 0.9358974358974359031, 0.9423076923076922906 ),
 .UNSPECIFIED. ) 
 CURVE ( )  GEOMETRIC_REPRESENTATION_ITEM ( )  RATIONAL_B_SPLINE_CURVE ( ( 0.9330127018922194093, 0.9330127018922194093, 1.000000000000000000, 0.8660254037844387076, 1.000000000000000000, 0.8660254037844387076, 1.000000000000000000, 0.9330127018922194093, 0.9330127018922194093 ) ) 
 REPRESENTATION_ITEM ( '' )  );
#2059=DIRECTION ( 'NONE',  ( 0.9928203230275511881, 0.1196152422706614482, 0.000000000000000000 ) ) ;
#2063=ORIENTED_EDGE ( 'NONE', *, *, #10851, .T. ) ;
#2074=CARTESIAN_POINT ( 'NONE',  ( 32.28234893270314387, -5.401404424200516807, -7.939653947423664704 ) ) ;
#2079=CARTESIAN_POINT ( 'NONE',  ( 0.000000000000000000, 0.000000000000000000, -8.700000000000001066 ) ) ;
#2082=EDGE_CURVE ( 'NONE', #6537, #13858, #8523, .T. ) ;
#2084=AXIS2_PLACEMENT_3D ( 'NONE', #8243, #5992, #7288 ) ;
#2088=CIRCLE ( 'NONE', #6117, 13.00000000000000178 ) ;
#2090=DIRECTION ( 'NONE',  ( -0.1196152422706611984, 0.9928203230275510771, 0.000000000000000000 ) ) ;
#2092=CARTESIAN_POINT ( 'NONE',  ( 15.92260893619738837, -28.39189527176317540, -16.15082599432113142 ) ) ;
#2094=CARTESIAN_POINT ( 'NONE',  ( -17.40358024347774091, -19.00834140588416332, -15.93963985190277910 ) ) ;
#2096=AXIS2_PLACEMENT_3D ( 'NONE', #4505, #9013, #2405 ) ;
#2098=CARTESIAN_POINT ( 'NONE',  ( -8.632250723006720250, -18.84644399697197770, -13.00000000000000178 ) ) ;
#2104=VERTEX_POINT ( 'NONE', #16884 ) ;
#2106=CARTESIAN_POINT ( 'NONE',  ( 25.83772294520678159, -3.669972453104032084, -3.627061608673662896 ) ) ;
#2108=VERTEX_POINT ( 'NONE', #10045 ) ;
#2114=CARTESIAN_POINT ( 'NONE',  ( 29.07687923786957285, -2.352938776424351008, -7.033357778048658027 ) ) ;
#2115=CARTESIAN_POINT ( 'NONE',  ( 30.04066231269008469, -3.163601260824890904, -7.939653947423660263 ) ) ;
#2122=EDGE_CURVE ( 'NONE', #11176, #13499, #11590, .T. ) ;
#2124=CARTESIAN_POINT ( 'NONE',  ( 27.04606801335823718, -3.524390735323772006, -7.939653947423660263 ) ) ;
#2126=CARTESIAN_POINT ( 'NONE',  ( 25.81099976294218479, -6.186279776075334524, -7.540300355390971987 ) ) ;
#2127=CARTESIAN_POINT ( 'NONE',  ( 27.84978555093622177, -3.227686124957687586, -8.283357778048660691 ) ) ;
#2128=CARTESIAN_POINT ( 'NONE',  ( 27.18555652250208610, -2.580805812949960920, -7.033357778048658027 ) ) ;
#2133=ADVANCED_FACE ( 'NONE', ( #14241 ), #17160, .F. ) ;
#2136=CARTESIAN_POINT ( 'NONE',  ( 28.53771668024168662, -2.080538600569502794, -5.783357778048658027 ) ) ;
#2144=CARTESIAN_POINT ( 'NONE',  ( 32.82963640218302004, -5.962437625020304388, -4.705209693361169343 ) ) ;
#2145=LINE ( 'NONE', #2321, #7341 ) ;
#2148=CARTESIAN_POINT ( 'NONE',  ( 28.09753128235661279, -6.832371619143005503, -4.533357778048668685 ) ) ;
#2149=DIRECTION ( 'NONE',  ( 0.9928203230275512992, 0.1196152422706614482, 0.000000000000000000 ) ) ;
#2164=ORIENTED_EDGE ( 'NONE', *, *, #6228, .F. ) ;
#2168=EDGE_CURVE ( 'NONE', #15348, #7502, #4785, .T. ) ;
#2169=CARTESIAN_POINT ( 'NONE',  ( 32.50119254608192421, -4.121097024973739309, -3.627061608673664672 ) ) ;
#2170=( BOUNDED_CURVE ( )  B_SPLINE_CURVE ( 2, ( #3547, #12323, #8596, #16419, #8158, #5418, #12405, #11027, #9671 ),
 .UNSPECIFIED., .F., .T. ) 
 B_SPLINE_CURVE_WITH_KNOTS ( ( 3, 2, 2, 2, 3 ),
 ( 0.2500000000000000000, 0.2564102564102563875, 0.2692307692307692180, 0.2820512820512820484, 0.2884615384615384914 ),
 .UNSPECIFIED. ) 
 CURVE ( )  GEOMETRIC_REPRESENTATION_ITEM ( )  RATIONAL_B_SPLINE_CURVE ( ( 0.9330127018922194093, 0.9330127018922195203, 1.000000000000000000, 0.8660254037844387076, 1.000000000000000000, 0.8660254037844387076, 1.000000000000000000, 0.9330127018922190762, 0.9330127018922194093 ) ) 
 REPRESENTATION_ITEM ( '' )  );
#2175=CARTESIAN_POINT ( 'NONE',  ( 31.61111609099199171, -1.710254666422835745, -5.783357778048662468 ) ) ;
#2177=ORIENTED_EDGE ( 'NONE', *, *, #13897, .T. ) ;
#2183=CARTESIAN_POINT ( 'NONE',  ( -9.099998387031003944, -19.29508120620799616, -16.81964500401478091 ) ) ;
#2185=CARTESIAN_POINT ( 'NONE',  ( -45.50000000000000000, -19.03270077640483038, -8.287981825772241962 ) ) ;
#2190=LINE ( 'NONE', #7621, #15372 ) ;
#2193=( BOUNDED_CURVE ( )  B_SPLINE_CURVE ( 2, ( #3270, #15780, #8802, #14334, #11589, #3355, #8887, #5320, #13505 ),
 .UNSPECIFIED., .F., .T. ) 
 B_SPLINE_CURVE_WITH_KNOTS ( ( 3, 2, 2, 2, 3 ),
 ( 0.5192307692307692735, 0.5256410256410256610, 0.5384615384615384359, 0.5512820512820513219, 0.5576923076923077094 ),
 .UNSPECIFIED. ) 
 CURVE ( )  GEOMETRIC_REPRESENTATION_ITEM ( )  RATIONAL_B_SPLINE_CURVE ( ( 0.9330127018922192983, 0.9330127018922198534, 1.000000000000000000, 0.8660254037844387076, 1.000000000000000000, 0.8660254037844387076, 1.000000000000000000, 0.9330127018922194093, 0.9330127018922194093 ) ) 
 REPRESENTATION_ITEM ( '' )  );
#2194=FACE_OUTER_BOUND ( 'NONE', #12338, .T. ) ;
#2197=CARTESIAN_POINT ( 'NONE',  ( 26.24062359194589078, -6.129313013101781671, -3.627061608673667781 ) ) ;
#2200=DIRECTION ( 'NONE',  ( 0.000000000000000000, 0.000000000000000000, 1.000000000000000000 ) ) ;
#2205=CARTESIAN_POINT ( 'NONE',  ( 31.38469755857769528, -2.374701023479507178, -4.705209693361161349 ) ) ;
#2206=ORIENTED_EDGE ( 'NONE', *, *, #3217, .T. ) ;
#2207=DIRECTION ( 'NONE',  ( 0.000000000000000000, 0.000000000000000000, -1.000000000000000000 ) ) ;
#2208=CARTESIAN_POINT ( 'NONE',  ( 26.03655646321512052, -5.068638614726478586, -8.187879365734106685 ) ) ;
#2209=EDGE_CURVE ( 'NONE', #17076, #8205, #13389, .T. ) ;
#2212=CARTESIAN_POINT ( 'NONE',  ( 31.00199007654869732, -2.847907730748336252, -8.283357778048658915 ) ) ;
#2214=CARTESIAN_POINT ( 'NONE',  ( 26.88845778707760914, -3.543379655034240905, -7.939653947423660263 ) ) ;
#2216=CARTESIAN_POINT ( 'NONE',  ( 32.37175601071535169, -5.590505156207296267, -3.283357778048667797 ) ) ;
#2221=EDGE_LOOP ( 'NONE', ( #4763, #5855, #16871, #3173 ) ) ;
#2224=DIRECTION ( 'NONE',  ( 0.000000000000000000, 0.000000000000000000, 1.000000000000000000 ) ) ;
#2229=DIRECTION ( 'NONE',  ( 0.000000000000000000, 0.000000000000000000, 1.000000000000000000 ) ) ;
#2232=CARTESIAN_POINT ( 'NONE',  ( 30.12771560522282499, -7.314681293660012074, -5.783357778048669573 ) ) ;
#2233=FACE_OUTER_BOUND ( 'NONE', #13086, .T. ) ;
#2236=DIRECTION ( 'NONE',  ( 0.9928203230275512992, 0.1196152422706614898, -0.000000000000000000 ) ) ;
#2242=ORIENTED_EDGE ( 'NONE', *, *, #608, .T. ) ;
#2245=( NAMED_UNIT ( * ) PLANE_ANGLE_UNIT ( ) SI_UNIT ( $, .RADIAN. ) );
#2251=CARTESIAN_POINT ( 'NONE',  ( 32.06767520579373354, -2.292415704734142690, -6.861505862736158257 ) ) ;
#2253=EDGE_CURVE ( 'NONE', #1497, #8671, #17443, .T. ) ;
#2257=AXIS2_PLACEMENT_3D ( 'NONE', #15530, #4553, #404 ) ;
#2258=CARTESIAN_POINT ( 'NONE',  ( 26.82912971812489644, -6.258282166232842947, -8.283357778048664244 ) ) ;
#2262=EDGE_CURVE ( 'NONE', #7372, #496, #3710, .T. ) ;
#2271=DIRECTION ( 'NONE',  ( 1.000000000000000000, 0.000000000000000000, 0.000000000000000000 ) ) ;
#2274=CARTESIAN_POINT ( 'NONE',  ( 33.04340326765378677, -1.875050963503474222, -4.533357778048659803 ) ) ;
#2281=CARTESIAN_POINT ( 'NONE',  ( 31.44176105920648823, -5.502678662656354192, -3.627061608673668225 ) ) ;
#2290=CARTESIAN_POINT ( 'NONE',  ( 32.77257290155422709, -2.834459985843462260, -3.627061608673662896 ) ) ;
#2299=CARTESIAN_POINT ( 'NONE',  ( 32.22908376348204484, -1.973160382215000785, -7.033357778048658027 ) ) ;
#2302=CARTESIAN_POINT ( 'NONE',  ( 28.13194630731337753, -5.901445976576171759, -3.627061608673667781 ) ) ;
#2312=DIRECTION ( 'NONE',  ( 0.000000000000000000, 0.000000000000000000, 1.000000000000000000 ) ) ;
#2313=CARTESIAN_POINT ( 'NONE',  ( -19.71718888926883650, -28.93397812220196030, -15.64003640126278682 ) ) ;
#2320=ORIENTED_EDGE ( 'NONE', *, *, #17453, .T. ) ;
#2321=CARTESIAN_POINT ( 'NONE',  ( -45.00000000000000711, -16.03270077640482683, -0.5379818257722508434 ) ) ;
#2323=ADVANCED_FACE ( 'NONE', ( #2619 ), #6958, .F. ) ;
#2324=CARTESIAN_POINT ( 'NONE',  ( 27.53837573810956130, -6.172832027328289506, -8.283357778048662468 ) ) ;
#2325=CARTESIAN_POINT ( 'NONE',  ( -3.538288549924106796, -15.34800872113743431, -16.99955934415556769 ) ) ;
#2333=ADVANCED_FACE ( 'NONE', ( #3809 ), #12134, .F. ) ;
#2334=VERTEX_POINT ( 'NONE', #10754 ) ;
#2335=AXIS2_PLACEMENT_3D ( 'NONE', #8561, #1680, #16923 ) ;
#2344=CARTESIAN_POINT ( 'NONE',  ( 33.76207435632690590, -3.969185667289998332, -3.627061608673664672 ) ) ;
#2347=CARTESIAN_POINT ( 'NONE',  ( 33.95908713831673964, -3.945449517755637903, -5.783357778048663356 ) ) ;
#2348=CARTESIAN_POINT ( 'NONE',  ( 30.09392748191118017, -6.591845302810410701, -7.033357778048666908 ) ) ;
#2351=CARTESIAN_POINT ( 'NONE',  ( -23.00000000000000000, -16.21813761408365195, 0.000000000000000000 ) ) ;
#2352=CARTESIAN_POINT ( 'NONE',  ( 26.82229025357024454, -7.323371595517525812, -5.113484796970862334 ) ) ;
#2356=ORIENTED_EDGE ( 'NONE', *, *, #12370, .T. ) ;
#2361=ORIENTED_EDGE ( 'NONE', *, *, #11040, .F. ) ;
#2366=CARTESIAN_POINT ( 'NONE',  ( -2.016448651773435938E-27, -20.49999999999999645, -6.000000000000000000 ) ) ;
#2368=CARTESIAN_POINT ( 'NONE',  ( 28.53771668024168662, -2.080538600569502794, -5.783357778048658027 ) ) ;
#2372=AXIS2_PLACEMENT_3D ( 'NONE', #8904, #6081, #2207 ) ;
#2375=CARTESIAN_POINT ( 'NONE',  ( 31.66930131758986988, -2.967382423816733894, -3.627061608673662008 ) ) ;
#2377=ORIENTED_EDGE ( 'NONE', *, *, #5084, .T. ) ;
#2384=MECHANICAL_DESIGN_GEOMETRIC_PRESENTATION_REPRESENTATION('',(#3231),#5206);
#2385=CARTESIAN_POINT ( 'NONE',  ( 29.60297508593253468, -5.724216059278466773, -7.939653947423662927 ) ) ;
#2388=CARTESIAN_POINT ( 'NONE',  ( 27.99987602667382802, -2.482696394238434578, -4.533357778048659803 ) ) ;
#2391=CARTESIAN_POINT ( 'NONE',  ( 30.49166216014303643, -4.363205751385915931, -8.283357778048662468 ) ) ;
#2392=CARTESIAN_POINT ( 'NONE',  ( 32.97402322492378346, -4.064130265842336165, -3.627061608673664672 ) ) ;
#2394=LINE ( 'NONE', #1024, #338 ) ;
#2395=CARTESIAN_POINT ( 'NONE',  ( 32.60321786976872005, -6.626883982076972934, -5.783357778048663356 ) ) ;
#2396=CARTESIAN_POINT ( 'NONE',  ( 27.17934203385504333, -30.00000000000000355, -13.93658524716016878 ) ) ;
#2399=AXIS2_PLACEMENT_3D ( 'NONE', #2434, #10734, #2509 ) ;
#2400=VECTOR ( 'NONE', #12040, 1000.000000000000000 ) ;
#2405=DIRECTION ( 'NONE',  ( 0.000000000000000000, 0.000000000000000000, 1.000000000000000000 ) ) ;
#2406=CARTESIAN_POINT ( 'NONE',  ( 33.13163345120441505, -4.045141346131868154, -3.627061608673664672 ) ) ;
#2409=CARTESIAN_POINT ( 'NONE',  ( 25.61697401368257587, -3.496695820648536568, -3.283357778048662023 ) ) ;
#2415=ORIENTED_EDGE ( 'NONE', *, *, #10044, .T. ) ;
#2419=DIRECTION ( 'NONE',  ( 0.000000000000000000, 0.000000000000000000, -1.000000000000000000 ) ) ;
#2420=DIRECTION ( 'NONE',  ( -1.000000000000000000, 0.000000000000000000, 0.000000000000000000 ) ) ;
#2425=AXIS2_PLACEMENT_3D ( 'NONE', #3894, #12492, #17884 ) ;
#2426=CARTESIAN_POINT ( 'NONE',  ( 31.69574812466957781, -6.726019302751734763, -5.783357778048669573 ) ) ;
#2430=PLANE ( 'NONE',  #8384 ) ;
#2434=CARTESIAN_POINT ( 'NONE',  ( -20.00000000000000000, -30.00000000000000355, -17.00000000000000000 ) ) ;
#2435=CARTESIAN_POINT ( 'NONE',  ( 31.34233605952372415, -6.778795339760710803, -5.783357778048663356 ) ) ;
#2444=ORIENTED_EDGE ( 'NONE', *, *, #992, .F. ) ;
#2450=ADVANCED_FACE ( 'NONE', ( #5496 ), #13939, .F. ) ;
#2455=ORIENTED_EDGE ( 'NONE', *, *, #12047, .T. ) ;
#2457=CARTESIAN_POINT ( 'NONE',  ( 30.41294626588012306, -6.253601060580800564, -6.861505862736167138 ) ) ;
#2459=ORIENTED_EDGE ( 'NONE', *, *, #6673, .F. ) ;
#2463=ORIENTED_EDGE ( 'NONE', *, *, #10233, .T. ) ;
#2465=CARTESIAN_POINT ( 'NONE',  ( 28.13194630731337753, -5.901445976576172647, -3.627061608673667781 ) ) ;
#2468=CARTESIAN_POINT ( 'NONE',  ( 27.93543013035303701, -2.153102235610331316, -5.113484796970857893 ) ) ;
#2470=CARTESIAN_POINT ( 'NONE',  ( 32.89331279191618762, -2.620040694222726785, -8.283357778048658915 ) ) ;
#2472=CARTESIAN_POINT ( 'NONE',  ( 32.64557936882268052, -2.222789665795767089, -4.705209693361161349 ) ) ;
#2473=CARTESIAN_POINT ( 'NONE',  ( -35.74085044863416272, -23.57886868891566223, -11.27079897466147607 ) ) ;
#2474=CARTESIAN_POINT ( 'NONE',  ( 30.66124439477291475, -6.860853434864224276, -6.453230759126470595 ) ) ;
#2484=DIRECTION ( 'NONE',  ( 1.000000000000000000, 0.000000000000000000, 0.000000000000000000 ) ) ;
#2485=EDGE_CURVE ( 'NONE', #987, #4619, #6458, .T. ) ;
#2486=CARTESIAN_POINT ( 'NONE',  ( 26.83664947211162399, -6.984282976826746037, -4.533357778048668685 ) ) ;
#2490=CARTESIAN_POINT ( 'NONE',  ( 27.95193767517966776, -20.05341752217977103, -13.73231903009881627 ) ) ;
#2496=VERTEX_POINT ( 'NONE', #6178 ) ;
#2502=CARTESIAN_POINT ( 'NONE',  ( 29.55043834383899437, -5.730545699181964991, -3.627061608673668225 ) ) ;
#2503=LINE ( 'NONE', #8213, #15307 ) ;
#2506=ORIENTED_EDGE ( 'NONE', *, *, #17430, .T. ) ;
#2508=EDGE_CURVE ( 'NONE', #9311, #17066, #4894, .T. ) ;
#2509=DIRECTION ( 'NONE',  ( 0.9396926207859104263, 0.000000000000000000, -0.3420201433256631063 ) ) ;
#2510=CARTESIAN_POINT ( 'NONE',  ( 30.88568772756644520, -4.315733451902305617, -3.283357778048664688 ) ) ;
#2516=ORIENTED_EDGE ( 'NONE', *, *, #14445, .F. ) ;
#2518=CARTESIAN_POINT ( 'NONE',  ( -2.749999999999992895, -20.49999999999999645, -6.000000000000000000 ) ) ;
#2522=CARTESIAN_POINT ( 'NONE',  ( 27.53837573810955419, -6.172832027328289506, -8.283357778048664244 ) ) ;
#2524=CARTESIAN_POINT ( 'NONE',  ( 28.67914455963771303, -4.581578327848842669, -8.283357778048662468 ) ) ;
#2531=EDGE_CURVE ( 'NONE', #5172, #3447, #14651, .T. ) ;
#2532=CARTESIAN_POINT ( 'NONE',  ( 32.95662993491455950, -6.574107945067995118, -5.783357778048669573 ) ) ;
#2535=CARTESIAN_POINT ( 'NONE',  ( 35.74085044863416982, -23.57886868891565513, -11.27079897466147251 ) ) ;
#2544=CARTESIAN_POINT ( 'NONE',  ( 28.87615734162756453, -4.557842178314484016, -7.939653947423662039 ) ) ;
#2549=DIRECTION ( 'NONE',  ( -0.000000000000000000, 1.000000000000000000, 0.000000000000000000 ) ) ;
#2550=CARTESIAN_POINT ( 'NONE',  ( 31.59864285835955400, -2.049116061056871274, -7.033357778048658027 ) ) ;
#2553=VERTEX_POINT ( 'NONE', #13174 ) ;
#2555=CARTESIAN_POINT ( 'NONE',  ( 32.12473870642251939, -5.420393343910986594, -7.939653947423664704 ) ) ;
#2561=VECTOR ( 'NONE', #287, 1000.000000000000114 ) ;
#2569=CARTESIAN_POINT ( 'NONE',  ( 29.34898802046944155, -4.500875419183088866, -3.627061608673664672 ) ) ;
#2572=CARTESIAN_POINT ( 'NONE',  ( 26.97551107961034944, -7.694459687869362519, -5.783357778048669573 ) ) ;
#2576=AXIS2_PLACEMENT_3D ( 'NONE', #15181, #3944, #2420 ) ;
#2591=CARTESIAN_POINT ( 'NONE',  ( 29.66420847303068697, -4.462897579762144851, -7.939653947423662039 ) ) ;
#2592=CARTESIAN_POINT ( 'NONE',  ( -8.632250723006720250, -18.84644399697197770, -13.00000000000000178 ) ) ;
#2606=ORIENTED_EDGE ( 'NONE', *, *, #13713, .F. ) ;
#2607=EDGE_CURVE ( 'NONE', #15344, #11718, #10187, .T. ) ;
#2615=DIRECTION ( 'NONE',  ( 1.000000000000000000, 0.000000000000000000, 0.000000000000000000 ) ) ;
#2617=CARTESIAN_POINT ( 'NONE',  ( 28.83304567166618781, -6.743756660494150346, -7.033357778048666908 ) ) ;
#2619=FACE_OUTER_BOUND ( 'NONE', #582, .T. ) ;
#2621=CARTESIAN_POINT ( 'NONE',  ( 19.22414633752738666, -11.22056979495215145, -15.64782563911137814 ) ) ;
#2625=EDGE_LOOP ( 'NONE', ( #3898, #4989 ) ) ;
#2626=CARTESIAN_POINT ( 'NONE',  ( 29.97942892559193950, -4.424919740341219487, -3.627061608673664672 ) ) ;
#2630=CARTESIAN_POINT ( 'NONE',  ( 33.95908713831673964, -3.945449517755637014, -5.783357778048663356 ) ) ;
#2633=VERTEX_POINT ( 'NONE', #2396 ) ;
#2635=CARTESIAN_POINT ( 'NONE',  ( 26.98483462626008134, -4.785709214840094816, -7.939653947423662039 ) ) ;
#2636=EDGE_CURVE ( 'NONE', #7694, #1336, #12263, .T. ) ;
#2643=FACE_BOUND ( 'NONE', #2625, .T. ) ;
#2644=CARTESIAN_POINT ( 'NONE',  ( 29.04309111455793513, -1.630102785574754742, -5.783357778048658027 ) ) ;
#2646=EDGE_LOOP ( 'NONE', ( #1255, #9227, #4565, #15437 ) ) ;
#2658=CARTESIAN_POINT ( 'NONE',  ( 5.237433445017501299, -16.51494876461869410, -16.99438405180048761 ) ) ;
#2659=ORIENTED_EDGE ( 'NONE', *, *, #10282, .T. ) ;
#2660=( NAMED_UNIT ( * ) SI_UNIT ( $, .STERADIAN. ) SOLID_ANGLE_UNIT ( ) );
#2661=CARTESIAN_POINT ( 'NONE',  ( 30.30787278169304244, -6.266260340387784566, -4.705209693361169343 ) ) ;
#2662=CARTESIAN_POINT ( 'NONE',  ( 26.01652455409633902, -4.902371455920928156, -5.783357778048663356 ) ) ;
#2664=CARTESIAN_POINT ( 'NONE',  ( 32.75517961154501023, -5.344437665069116328, -7.939653947423664704 ) ) ;
#2667=CIRCLE ( 'NONE', #7875, 25.00000000000000000 ) ;
#2671=CARTESIAN_POINT ( 'NONE',  ( 24.43282520912215006, -22.30499949230690504, -14.60822674442184699 ) ) ;
#2677=CARTESIAN_POINT ( 'NONE',  ( 32.61569110240115776, -6.288022587442930522, -7.033357778048666908 ) ) ;
#2678=VECTOR ( 'NONE', #9218, 1000.000000000000000 ) ;
#2682=CARTESIAN_POINT ( 'NONE',  ( 29.15206445563513071, -6.405512418264540209, -6.861505862736167138 ) ) ;
#2685=DIRECTION ( 'NONE',  ( -1.000000000000000000, -1.501955125927555231E-12, 0.000000000000000000 ) ) ;
#2689=VECTOR ( 'NONE', #14563, 1000.000000000000000 ) ;
#2699=AXIS2_PLACEMENT_3D ( 'NONE', #13941, #7069, #164 ) ;
#2701=EDGE_CURVE ( 'NONE', #6328, #3112, #1520, .T. ) ;
#2707=CARTESIAN_POINT ( 'NONE',  ( 32.92264866086529906, -1.552240892477451784, -6.453230759126466154 ) ) ;
#2714=CARTESIAN_POINT ( 'NONE',  ( 0.000000000000000000, 0.000000000000000000, -6.000000000000000000 ) ) ;
#2717=EDGE_CURVE ( 'NONE', #11807, #11418, #4188, .T. ) ;
#2718=CARTESIAN_POINT ( 'NONE',  ( 28.93739072872572393, -3.296523698798161650, -7.939653947423660263 ) ) ;
#2723=ORIENTED_EDGE ( 'NONE', *, *, #17198, .T. ) ;
#2726=CARTESIAN_POINT ( 'NONE',  ( 28.35948656569676629, -3.366149737736551906, -3.627061608673662896 ) ) ;
#2727=DIRECTION ( 'NONE',  ( 0.5661261679878573094, 0.8243186046180107640, -0.000000000000000000 ) ) ;
#2732=CYLINDRICAL_SURFACE ( 'NONE', #12468, 13.00000000000000178 ) ;
#2734=CARTESIAN_POINT ( 'NONE',  ( 27.87986455999572399, -6.131689368163069531, -3.283357778048667797 ) ) ;
#2735=( BOUNDED_CURVE ( )  B_SPLINE_CURVE ( 2, ( #17460, #9085, #12978, #14627, #14351, #5983, #14711, #17269, #10247 ),
 .UNSPECIFIED., .F., .F. ) 
 B_SPLINE_CURVE_WITH_KNOTS ( ( 3, 2, 2, 2, 3 ),
 ( 0.4807692307692307820, 0.4871794871794871695, 0.5000000000000000000, 0.5128205128205127750, 0.5192307692307692735 ),
 .UNSPECIFIED. ) 
 CURVE ( )  GEOMETRIC_REPRESENTATION_ITEM ( )  RATIONAL_B_SPLINE_CURVE ( ( 0.9330127018922194093, 0.9330127018922196314, 1.000000000000000000, 0.8660254037844387076, 1.000000000000000000, 0.8660254037844387076, 1.000000000000000000, 0.9330127018922187432, 0.9330127018922192983 ) ) 
 REPRESENTATION_ITEM ( '' )  );
#2738=CYLINDRICAL_SURFACE ( 'NONE', #11178, 2.499999999999999112 ) ;
#2746=DIRECTION ( 'NONE',  ( 0.000000000000000000, 0.000000000000000000, 1.000000000000000000 ) ) ;
#2747=ORIENTED_EDGE ( 'NONE', *, *, #3548, .F. ) ;
#2748=DIRECTION ( 'NONE',  ( 0.000000000000000000, 0.000000000000000000, 1.000000000000000000 ) ) ;
#2751=CARTESIAN_POINT ( 'NONE',  ( 30.29464937815318493, -4.386941900920275472, -7.939653947423662039 ) ) ;
#2754=CARTESIAN_POINT ( 'NONE',  ( 25.96969170380761582, -2.000386719721422235, -5.783357778048658027 ) ) ;
#2755=DIRECTION ( 'NONE',  ( 1.000000000000000000, 0.000000000000000000, -0.000000000000000000 ) ) ;
#2756=DIRECTION ( 'NONE',  ( 0.000000000000000000, -1.000000000000000000, 0.000000000000000000 ) ) ;
#2760=CARTESIAN_POINT ( 'NONE',  ( 20.27597925817430635, -21.85809165190032743, -15.46244260681514326 ) ) ;
#2761=VERTEX_POINT ( 'NONE', #1202 ) ;
#2769=EDGE_CURVE ( 'NONE', #14246, #7494, #9602, .T. ) ;
#2771=CARTESIAN_POINT ( 'NONE',  ( 33.78529456515154550, -6.484467084455914687, -5.783357778048663356 ) ) ;
#2772=CARTESIAN_POINT ( 'NONE',  ( 28.91999743871649997, -5.806501378023834370, -3.627061608673668225 ) ) ;
#2775=CARTESIAN_POINT ( 'NONE',  ( 31.17093069310692499, -6.462087684996337345, -4.533357778048668685 ) ) ;
#2778=CARTESIAN_POINT ( 'NONE',  ( 26.01595305975170547, -2.384361315936983416, -5.783357778048670461 ) ) ;
#2784=VERTEX_POINT ( 'NONE', #13973 ) ;
#2792=DIRECTION ( 'NONE',  ( -1.000000000000000000, 0.000000000000000000, 0.000000000000000000 ) ) ;
#2795=CARTESIAN_POINT ( 'NONE',  ( 29.03376756790819613, -4.538853258604016006, -7.939653947423662039 ) ) ;
#2797=CARTESIAN_POINT ( 'NONE',  ( 30.68374079916737429, -6.858143062403621926, -5.113484796970860558 ) ) ;
#2804=DIRECTION ( 'NONE',  ( 0.6000000000000001998, 0.7999999999999999334, 0.000000000000000000 ) ) ;
#2807=DIRECTION ( 'NONE',  ( -1.000000000000000000, 0.000000000000000000, 0.000000000000000000 ) ) ;
#2810=ADVANCED_FACE ( 'NONE', ( #16359 ), #3920, .F. ) ;
#2812=CARTESIAN_POINT ( 'NONE',  ( 26.55511561737958814, -2.656761491791831187, -7.033357778048658027 ) ) ;
#2814=CARTESIAN_POINT ( 'NONE',  ( 30.75425665345519732, -2.450656702321377001, -4.705209693361161349 ) ) ;
#2822=CARTESIAN_POINT ( 'NONE',  ( 26.31556265977298992, -7.384422263489805793, -5.783357778048663356 ) ) ;
#2823=CARTESIAN_POINT ( 'NONE',  ( 2.749999999999988454, -20.49999999999999645, -13.00000000000000355 ) ) ;
#2826=ORIENTED_EDGE ( 'NONE', *, *, #13713, .T. ) ;
#2829=CARTESIAN_POINT ( 'NONE',  ( 31.56875459193803124, -6.114348982704044921, -4.705209693361169343 ) ) ;
#2830=CARTESIAN_POINT ( 'NONE',  ( 29.39282811755836633, -5.749534618892433002, -3.627061608673667781 ) ) ;
#2831=EDGE_CURVE ( 'NONE', #16316, #7502, #3825, .T. ) ;
#2832=DIRECTION ( 'NONE',  ( 1.000000000000000000, 0.000000000000000000, 0.000000000000000000 ) ) ;
#2850=ORIENTED_EDGE ( 'NONE', *, *, #3407, .T. ) ;
#2851=CARTESIAN_POINT ( 'NONE',  ( 27.91310269393460430, -7.181753375802955475, -5.783357778048669573 ) ) ;
#2853=DIRECTION ( 'NONE',  ( 0.000000000000000000, -1.000000000000000000, 0.000000000000000000 ) ) ;
#2864=EDGE_LOOP ( 'NONE', ( #12798, #17774, #14164, #12910, #16398, #6826, #3386, #16138, #12474, #5065, #5356 ) ) ;
#2866=VERTEX_POINT ( 'NONE', #8811 ) ;
#2869=ORIENTED_EDGE ( 'NONE', *, *, #510, .F. ) ;
#2874=CARTESIAN_POINT ( 'NONE',  ( 23.00000000000000000, -16.21813761408365195, -13.00000000000000178 ) ) ;
#2878=DIRECTION ( 'NONE',  ( -0.1196152422706611984, 0.9928203230275510771, 0.000000000000000000 ) ) ;
#2881=CARTESIAN_POINT ( 'NONE',  ( 26.29446227649215473, -10.90310086042137350, -14.16253947949896563 ) ) ;
#2886=CARTESIAN_POINT ( 'NONE',  ( 30.71189515440122975, -6.854751018602581958, -5.783357778048663356 ) ) ;
#2887=EDGE_CURVE ( 'NONE', #10072, #11560, #9139, .T. ) ;
#2890=VERTEX_POINT ( 'NONE', #12787 ) ;
#2894=CARTESIAN_POINT ( 'NONE',  ( 25.81704846941310549, -3.246696919197674447, -4.409389677717624245 ) ) ;
#2895=EDGE_CURVE ( 'NONE', #2890, #14870, #14678, .T. ) ;
#2901=CARTESIAN_POINT ( 'NONE',  ( 27.45957062324739795, -6.182326487390973568, -8.283357778048662468 ) ) ;
#2902=CARTESIAN_POINT ( 'NONE',  ( 30.23341599105502908, -5.648260380436597394, -7.939653947423664704 ) ) ;
#2903=CARTESIAN_POINT ( 'NONE',  ( 28.21828588914510050, -7.155181690169023057, -6.453230759126468818 ) ) ;
#2904=DIRECTION ( 'NONE',  ( 0.9928203230275512992, 0.1196152422706614898, -0.000000000000000000 ) ) ;
#2915=VERTEX_POINT ( 'NONE', #7776 ) ;
#2916=CARTESIAN_POINT ( 'NONE',  ( -25.76257153370368869, -10.59741316493651730, -14.29454127969954591 ) ) ;
#2919=CARTESIAN_POINT ( 'NONE',  ( 30.81132015408399027, -5.578634341498224458, -3.627061608673668225 ) ) ;
#2922=ORIENTED_EDGE ( 'NONE', *, *, #10483, .F. ) ;
#2923=ORIENTED_EDGE ( 'NONE', *, *, #1056, .T. ) ;
#2924=CARTESIAN_POINT ( 'NONE',  ( 29.38830135902312080, -2.615227339812091767, -6.861505862736159145 ) ) ;
#2926=DIRECTION ( 'NONE',  ( 0.000000000000000000, 0.000000000000000000, -1.000000000000000000 ) ) ;
#2931=CARTESIAN_POINT ( 'NONE',  ( 17.31832318566733164, -18.83027996791590652, -15.95242868103980172 ) ) ;
#2932=VERTEX_POINT ( 'NONE', #4358 ) ;
#2934=VECTOR ( 'NONE', #4348, 1000.000000000000114 ) ;
#2948=CARTESIAN_POINT ( 'NONE',  ( 26.05393439953038381, -7.587479618990243146, -6.529799540429926274 ) ) ;
#2950=CARTESIAN_POINT ( 'NONE',  ( 32.55182397003001427, -2.661183353387966299, -3.283357778048662023 ) ) ;
#2955=LINE ( 'NONE', #8765, #15707 ) ;
#2956=CARTESIAN_POINT ( 'NONE',  ( 30.52163964716380917, -2.178873678870954400, -4.533357778048659803 ) ) ;
#2966=PRESENTATION_STYLE_ASSIGNMENT (( #9831 ) ) ;
#2967=CARTESIAN_POINT ( 'NONE',  ( 29.25000000000000000, -16.21813761408365195, -13.00000000000000178 ) ) ;
#2968=EDGE_CURVE ( 'NONE', #10333, #7372, #1837, .T. ) ;
#2973=CARTESIAN_POINT ( 'NONE',  ( -27.17934203385504333, -30.00000000000000355, 0.000000000000000000 ) ) ;
#2978=CARTESIAN_POINT ( 'NONE',  ( 26.59574320524588842, -2.314508053356755024, -5.113484796970857893 ) ) ;
#2985=ORIENTED_EDGE ( 'NONE', *, *, #1916, .F. ) ;
#2986=FACE_BOUND ( 'NONE', #16908, .T. ) ;
#2991=( GEOMETRIC_REPRESENTATION_CONTEXT ( 3 ) GLOBAL_UNCERTAINTY_ASSIGNED_CONTEXT ( ( #15507 ) ) GLOBAL_UNIT_ASSIGNED_CONTEXT ( ( #16275, #3846, #3749 ) ) REPRESENTATION_CONTEXT ( 'NONE', 'WORKASPACE' ) );
#2995=CARTESIAN_POINT ( 'NONE',  ( 29.34405387406022570, -7.019548880150045633, -5.113484796970862334 ) ) ;
#2996=CARTESIAN_POINT ( 'NONE',  ( -16.75000000000000000, -16.21813761408365195, -13.00000000000000178 ) ) ;
#3003=EDGE_CURVE ( 'NONE', #1161, #3273, #1203, .T. ) ;
#3004=UNCERTAINTY_MEASURE_WITH_UNIT (LENGTH_MEASURE( 1.000000000000000082E-05 ), #4939, 'distance_accuracy_value', 'NONE');
#3005=CARTESIAN_POINT ( 'NONE',  ( 28.55151181693415907, -2.416235175459247486, -4.533357778048659803 ) ) ;
#3006=CARTESIAN_POINT ( 'NONE',  ( 29.60297508593253468, -5.724216059278466773, -7.939653947423664704 ) ) ;
#3007=FACE_OUTER_BOUND ( 'NONE', #15954, .T. ) ;
#3009=CARTESIAN_POINT ( 'NONE',  ( 26.28374211850152875, -7.120308096563231715, -4.880631602441031447 ) ) ;
#3014=ORIENTED_EDGE ( 'NONE', *, *, #1141, .F. ) ;
#3017=CARTESIAN_POINT ( 'NONE',  ( 30.40162818048570514, -5.827866652795590241, -3.283357778048667797 ) ) ;
#3018=ORIENTED_EDGE ( 'NONE', *, *, #1433, .T. ) ;
#3019=CARTESIAN_POINT ( 'NONE',  ( 0.000000000000000000, 0.000000000000000000, -12.00000000000000000 ) ) ;
#3021=CARTESIAN_POINT ( 'NONE',  ( 27.86926259684567597, -5.933094176093607786, -7.939653947423662927 ) ) ;
#3023=CARTESIAN_POINT ( 'NONE',  ( 28.75786045390062995, -2.691183018653962034, -6.861505862736159145 ) ) ;
#3028=CARTESIAN_POINT ( 'NONE',  ( 29.11750682573587312, -2.010685337989277954, -5.113484796970851676 ) ) ;
#3037=EDGE_LOOP ( 'NONE', ( #5627, #13441, #17351, #13158 ) ) ;
#3039=EDGE_CURVE ( 'NONE', #14228, #15335, #10920, .T. ) ;
#3043=CARTESIAN_POINT ( 'NONE',  ( 26.41562710823574278, -3.600346414165641828, -7.939653947423660263 ) ) ;
#3044=CARTESIAN_POINT ( 'NONE',  ( 32.97211790677835097, -2.610546234160043610, -8.283357778048658915 ) ) ;
#3047=CARTESIAN_POINT ( 'NONE',  ( 31.23537658942770889, -6.791681843624433945, -5.113484796970860558 ) ) ;
#3050=LINE ( 'NONE', #11087, #9772 ) ;
#3052=( BOUNDED_CURVE ( )  B_SPLINE_CURVE ( 3, ( #7136, #4312, #12648, #4577 ),
 .UNSPECIFIED., .F., .T. ) 
 B_SPLINE_CURVE_WITH_KNOTS ( ( 4, 4 ),
 ( 1.436990331221392081, 1.509167199807614601 ),
 .UNSPECIFIED. ) 
 CURVE ( )  GEOMETRIC_REPRESENTATION_ITEM ( )  RATIONAL_B_SPLINE_CURVE ( ( 1.000000000000000000, 0.9995659220841806025, 0.9995659220841806025, 1.000000000000000000 ) ) 
 REPRESENTATION_ITEM ( '' )  );
#3053=ORIENTED_EDGE ( 'NONE', *, *, #8958, .T. ) ;
#3054=ORIENTED_EDGE ( 'NONE', *, *, #278, .F. ) ;
#3057=CARTESIAN_POINT ( 'NONE',  ( 45.00000000000000711, 0.000000000000000000, -5.537981825772250843 ) ) ;
#3060=VERTEX_POINT ( 'NONE', #1249 ) ;
#3067=EDGE_CURVE ( 'NONE', #15606, #4693, #9489, .T. ) ;
#3072=EDGE_CURVE ( 'NONE', #9324, #3060, #4044, .T. ) ;
#3074=CARTESIAN_POINT ( 'NONE',  ( 3.248936832696173393, -30.00000000000000355, 78.00000000000000000 ) ) ;
#3076=ORIENTED_EDGE ( 'NONE', *, *, #8489, .F. ) ;
#3079=ORIENTED_EDGE ( 'NONE', *, *, #6758, .T. ) ;
#3080=CARTESIAN_POINT ( 'NONE',  ( 28.48706592061337162, -2.086641016831144668, -5.113484796970857893 ) ) ;
#3085=FACE_OUTER_BOUND ( 'NONE', #11150, .T. ) ;
#3086=FACE_OUTER_BOUND ( 'NONE', #9549, .T. ) ;
#3088=EDGE_CURVE ( 'NONE', #7031, #15783, #17355, .T. ) ;
#3090=CARTESIAN_POINT ( 'NONE',  ( 26.86291784143654127, -6.981118157082444320, -7.033357778048666908 ) ) ;
#3091=CARTESIAN_POINT ( 'NONE',  ( 29.51982165028991645, -6.361204938940122844, -4.705209693361168455 ) ) ;
#3093=CARTESIAN_POINT ( 'NONE',  ( 26.31175009776946538, -7.352777558617343168, -6.181997573440047411 ) ) ;
#3096=DIRECTION ( 'NONE',  ( 1.000000000000000000, 0.000000000000000000, 0.000000000000000000 ) ) ;
#3102=CARTESIAN_POINT ( 'NONE',  ( -23.83446850436624587, -10.01089291621719646, -14.74374009921848483 ) ) ;
#3103=ORIENTED_EDGE ( 'NONE', *, *, #13488, .T. ) ;
#3106=CARTESIAN_POINT ( 'NONE',  ( 29.49337484321020497, -2.602568060005117090, -4.705209693361161349 ) ) ;
#3112=VERTEX_POINT ( 'NONE', #11936 ) ;
#3121=VERTEX_POINT ( 'NONE', #14766 ) ;
#3123=EDGE_CURVE ( 'NONE', #14839, #8562, #15222, .T. ) ;
#3124=ORIENTED_EDGE ( 'NONE', *, *, #16637, .T. ) ;
#3126=CARTESIAN_POINT ( 'NONE',  ( 28.49970350196817392, -5.857138497251738407, -7.939653947423664704 ) ) ;
#3127=CARTESIAN_POINT ( 'NONE',  ( 31.08079519141086777, -2.838413270685653078, -8.283357778048658915 ) ) ;
#3129=FACE_BOUND ( 'NONE', #12977, .T. ) ;
#3130=CARTESIAN_POINT ( 'NONE',  ( 29.55043834383899437, -5.730545699181964991, -3.627061608673668225 ) ) ;
#3138=ORIENTED_EDGE ( 'NONE', *, *, #5131, .F. ) ;
#3152=CARTESIAN_POINT ( 'NONE',  ( -20.00000000000000000, 7.999999999999996447, -15.51150668642334374 ) ) ;
#3159=EDGE_LOOP ( 'NONE', ( #16768, #15799, #16584 ) ) ;
#3163=FACE_OUTER_BOUND ( 'NONE', #13989, .T. ) ;
#3165=CARTESIAN_POINT ( 'NONE',  ( 20.00000000000000355, 7.999999999999996447, -6.000000000000000000 ) ) ;
#3169=CARTESIAN_POINT ( 'NONE',  ( 45.00000000000000711, -16.03270077640482683, -10.53798182577225084 ) ) ;
#3171=DIRECTION ( 'NONE',  ( -1.000000000000000000, 0.000000000000000000, 0.000000000000000000 ) ) ;
#3173=ORIENTED_EDGE ( 'NONE', *, *, #1569, .F. ) ;
#3174=CARTESIAN_POINT ( 'NONE',  ( 31.91459173804834748, -5.445711903524953712, -3.627061608673667781 ) ) ;
#3175=DIRECTION ( 'NONE',  ( 0.000000000000000000, 0.000000000000000000, -1.000000000000000000 ) ) ;
#3176=CARTESIAN_POINT ( 'NONE',  ( 32.55182397003001427, -2.661183353387966299, -3.283357778048662023 ) ) ;
#3177=CARTESIAN_POINT ( 'NONE',  ( 26.31376129264122810, -7.369470708288995198, -5.989870097397514748 ) ) ;
#3178=VECTOR ( 'NONE', #4550, 1000.000000000000227 ) ;
#3179=LINE ( 'NONE', #15329, #5442 ) ;
#3181=CARTESIAN_POINT ( 'NONE',  ( -23.00000000000000000, -16.21813761408365195, -13.00000000000000178 ) ) ;
#3183=EDGE_CURVE ( 'NONE', #9522, #1377, #13265, .T. ) ;
#3184=ORIENTED_EDGE ( 'NONE', *, *, #17716, .F. ) ;
#3189=CARTESIAN_POINT ( 'NONE',  ( -17.31608032955932330, -13.61075944537037508, -15.95276485144012035 ) ) ;
#3193=LINE ( 'NONE', #8730, #11627 ) ;
#3195=CARTESIAN_POINT ( 'NONE',  ( 29.41022140756759029, -3.239556939666760726, -7.939653947423660263 ) ) ;
#3196=CARTESIAN_POINT ( 'NONE',  ( 28.11132641904908169, -7.168068194032743534, -5.783357778048668685 ) ) ;
#3197=CARTESIAN_POINT ( 'NONE',  ( 33.16732689266149237, -6.221561368663743430, -7.033357778048666908 ) ) ;
#3201=ORIENTED_EDGE ( 'NONE', *, *, #1899, .F. ) ;
#3203=AXIS2_PLACEMENT_3D ( 'NONE', #13059, #12881, #8529 ) ;
#3204=EDGE_CURVE ( 'NONE', #1502, #3497, #6750, .T. ) ;
#3213=DIRECTION ( 'NONE',  ( 0.000000000000000000, 0.000000000000000000, 1.000000000000000000 ) ) ;
#3217=EDGE_CURVE ( 'NONE', #11718, #7736, #3050, .T. ) ;
#3218=CARTESIAN_POINT ( 'NONE',  ( 32.46178999037268653, -4.125844254797621957, -8.283357778048662468 ) ) ;
#3225=CARTESIAN_POINT ( 'NONE',  ( 31.21213704492286212, -2.822589171134389563, -3.283357778048662023 ) ) ;
#3231=STYLED_ITEM ( 'NONE', ( #2966 ), #11368 ) ;
#3236=CARTESIAN_POINT ( 'NONE',  ( 26.31128205117621022, -7.047579375861630524, -7.033357778048666908 ) ) ;
#3241=CARTESIAN_POINT ( 'NONE',  ( 35.41536221060850664, -16.03270077640482683, -10.53798182577225084 ) ) ;
#3245=EDGE_CURVE ( 'NONE', #8066, #12145, #6895, .T. ) ;
#3247=CIRCLE ( 'NONE', #2096, 2.749999999999988454 ) ;
#3251=DIRECTION ( 'NONE',  ( 0.9928203230275510771, 0.1196152422706621282, -0.000000000000000000 ) ) ;
#3259=AXIS2_PLACEMENT_3D ( 'NONE', #5486, #6945, #15287 ) ;
#3261=DIRECTION ( 'NONE',  ( -0.1196152422706611984, 0.9928203230275510771, 0.000000000000000000 ) ) ;
#3264=CARTESIAN_POINT ( 'NONE',  ( -29.20851401586840979, -17.04915871481012246, -13.38439546398730329 ) ) ;
#3270=CARTESIAN_POINT ( 'NONE',  ( 29.45101334415624095, -7.006662376286321603, -5.783357778048657138 ) ) ;
#3272=CARTESIAN_POINT ( 'NONE',  ( 26.89670596474818609, -7.703954147932045693, -5.783357778048669573 ) ) ;
#3273=VERTEX_POINT ( 'NONE', #1514 ) ;
#3275=CARTESIAN_POINT ( 'NONE',  ( 26.98483462626008134, -4.785709214840094816, -7.939653947423662039 ) ) ;
#3276=CARTESIAN_POINT ( 'NONE',  ( -45.00000000000000711, -19.03270077640483038, -5.537981825772250843 ) ) ;
#3277=CARTESIAN_POINT ( 'NONE',  ( 32.69820532807177216, -4.097360875439379768, -3.283357778048664688 ) ) ;
#3287=DIRECTION ( 'NONE',  ( 0.000000000000000000, -1.000000000000000000, -3.469446951953614189E-16 ) ) ;
#3290=CARTESIAN_POINT ( 'NONE',  ( 25.99533317148741318, -3.650983533393564517, -3.627061608673662008 ) ) ;
#3291=CARTESIAN_POINT ( 'NONE',  ( 25.99533317148741318, -3.650983533393564517, -3.627061608673662008 ) ) ;
#3293=CARTESIAN_POINT ( 'NONE',  ( 28.10549950023366961, -2.142809097641162897, -5.783357778048658027 ) ) ;
#3295=CARTESIAN_POINT ( 'NONE',  ( 26.01652455409633902, -4.902371455920928156, -5.783357778048663356 ) ) ;
#3296=CARTESIAN_POINT ( 'NONE',  ( 33.48996557372703364, -1.821249024531260696, -7.033357778048658027 ) ) ;
#3300=EDGE_CURVE ( 'NONE', #14246, #13718, #3052, .T. ) ;
#3307=VERTEX_POINT ( 'NONE', #15920 ) ;
#3308=LINE ( 'NONE', #134, #6075 ) ;
#3310=CARTESIAN_POINT ( 'NONE',  ( 27.32822876973539294, -6.198150586942257512, -3.283357778048667797 ) ) ;
#3311=ADVANCED_FACE ( 'NONE', ( #774 ), #6021, .T. ) ;
#3317=( BOUNDED_CURVE ( )  B_SPLINE_CURVE ( 3, ( #2473, #15996, #10606, #13352 ),
 .UNSPECIFIED., .F., .T. ) 
 B_SPLINE_CURVE_WITH_KNOTS ( ( 4, 4 ),
 ( 4.363323129985829496, 4.457746946181837977 ),
 .UNSPECIFIED. ) 
 CURVE ( )  GEOMETRIC_REPRESENTATION_ITEM ( )  RATIONAL_B_SPLINE_CURVE ( ( 1.000000000000000000, 0.9992571499088201969, 0.9992571499088201969, 1.000000000000000000 ) ) 
 REPRESENTATION_ITEM ( '' )  );
#3326=ORIENTED_EDGE ( 'NONE', *, *, #13518, .T. ) ;
#3333=CARTESIAN_POINT ( 'NONE',  ( 5.499998817156067865, -20.49639288455253450, -6.000000000000000000 ) ) ;
#3334=CARTESIAN_POINT ( 'NONE',  ( 33.58707084003705745, -6.498152266226123963, -5.783357778048669573 ) ) ;
#3346=FACE_OUTER_BOUND ( 'NONE', #5790, .T. ) ;
#3355=CARTESIAN_POINT ( 'NONE',  ( 28.76917853929504432, -3.116917426439186123, -3.283357778048662023 ) ) ;
#3359=ORIENTED_EDGE ( 'NONE', *, *, #11795, .F. ) ;
#3361=CARTESIAN_POINT ( 'NONE',  ( 25.81100034576892455, -6.186289477007987259, -7.540293452860097112 ) ) ;
#3363=ORIENTED_EDGE ( 'NONE', *, *, #12537, .T. ) ;
#3364=CARTESIAN_POINT ( 'NONE',  ( 27.17934203385504333, -30.00000000000000355, -12.00000000000000000 ) ) ;
#3368=FACE_BOUND ( 'NONE', #15608, .T. ) ;
#3369=EDGE_CURVE ( 'NONE', #15678, #5342, #7488, .T. ) ;
#3370=CARTESIAN_POINT ( 'NONE',  ( 31.25770402584614871, -1.763030703431812451, -5.783357778048658915 ) ) ;
#3371=ORIENTED_EDGE ( 'NONE', *, *, #2209, .T. ) ;
#3373=CARTESIAN_POINT ( 'NONE',  ( -35.74085044863416272, -18.73429073671335132, -11.27079897466147607 ) ) ;
#3374=CARTESIAN_POINT ( 'NONE',  ( 27.91310269393460430, -7.181753375802955475, -5.783357778048669573 ) ) ;
#3375=ORIENTED_EDGE ( 'NONE', *, *, #4866, .T. ) ;
#3377=CARTESIAN_POINT ( 'NONE',  ( 25.58373587974369201, -2.446631813008643075, -5.783357778048658027 ) ) ;
#3379=CARTESIAN_POINT ( 'NONE',  ( 33.50243880635947846, -1.482387629897225390, -5.783357778048663356 ) ) ;
#3385=EDGE_CURVE ( 'NONE', #1497, #9311, #14765, .T. ) ;
#3386=ORIENTED_EDGE ( 'NONE', *, *, #10791, .F. ) ;
#3389=CARTESIAN_POINT ( 'NONE',  ( 0.000000000000000000, 0.000000000000000000, -8.700000000000001066 ) ) ;
#3396=ADVANCED_FACE ( 'NONE', ( #10195 ), #8766, .F. ) ;
#3397=CARTESIAN_POINT ( 'NONE',  ( 29.89119874204131122, -2.254829357712824667, -4.533357778048659803 ) ) ;
#3401=CARTESIAN_POINT ( 'NONE',  ( 27.19802975513453092, -2.241944418315925613, -5.783357778048658027 ) ) ;
#3407=EDGE_CURVE ( 'NONE', #7967, #11475, #4755, .T. ) ;
#3410=DIRECTION ( 'NONE',  ( 0.9928203230275512992, 0.1196152422706614898, -0.000000000000000000 ) ) ;
#3411=VERTEX_POINT ( 'NONE', #17115 ) ;
#3413=CARTESIAN_POINT ( 'NONE',  ( -36.95907006869318678, -17.52584492564777818, -5.783357778048662468 ) ) ;
#3416=CARTESIAN_POINT ( 'NONE',  ( 32.80318959510331212, -2.203800746085299522, -4.705209693361160461 ) ) ;
#3424=EDGE_LOOP ( 'NONE', ( #10033, #5132, #2923, #10696 ) ) ;
#3425=CARTESIAN_POINT ( 'NONE',  ( 32.06776442294927421, -4.173316554281249147, -3.283357778048664688 ) ) ;
#3434=AXIS2_PLACEMENT_3D ( 'NONE', #1063, #9390, #17867 ) ;
#3436=DIRECTION ( 'NONE',  ( -0.000000000000000000, 0.000000000000000000, -1.000000000000000000 ) ) ;
#3440=CARTESIAN_POINT ( 'NONE',  ( 31.34233605952372415, -6.778795339760710803, -5.783357778048663356 ) ) ;
#3441=LINE ( 'NONE', #2098, #6686 ) ;
#3446=CARTESIAN_POINT ( 'NONE',  ( 26.61898274975073164, -6.283600725846810953, -3.283357778048667797 ) ) ;
#3447=VERTEX_POINT ( 'NONE', #958 ) ;
#3450=CARTESIAN_POINT ( 'NONE',  ( 28.25893984004492765, -6.513116296623863377, -4.705209693361168455 ) ) ;
#3456=( BOUNDED_SURFACE ( )  B_SPLINE_SURFACE ( 1, 2, ( 
 ( #8565, #4485, #12641, #17016, #10091, #3044, #11539, #8660, #14015, #4661, #139, #12915, #4569, #2950, #6013, #9817, #14098, #15640, #3218, #1598, #1684, #8760, #10189, #11254, #7040, #7130, #14290, #1876, #7405, #14189, #1781, #1506, #15738, #5833, #11357, #231, #7220, #12555, #11163, #5741, #16832, #3127, #4397, #9911, #15460, #12730, #7312, #327, #15543, #9999, #12830, #421, #15822, #6113, #17296, #4833, #11815, #6294, #13006, #13369, #854, #8841, #3397, #11641, #13103, #8926, #7665, #17580, #7745, #2232, #952, #5019, #14469, #10541, #3666, #11906, #17206, #5100, #6206, #14649, #10620, #4748, #1960, #6484, #10361, #680, #2050, #13190, #7575, #11725, #14378, #16105, #16193, #7839, #17394, #10274, #15915, #3487, #4925, #10455, #589, #11999, #6386, #7480, #9021, #14570, #2148, #767, #16015, #3588, #13274, #17493, #9111, #9192, #14736, #2324, #16532, #6827, #1040, #12444, #1122, #9535, #30, #17665, #14819, #13804, #5279, #8008, #14903, #2572, #2486, #16281, #9278, #17921, #5540, #2754, #1221, #6738, #16371, #6560, #10972, #16450, #1390, #8099, #11065, #2409, #12080, #10706, #3852, #5188, #6912, #4019, #1306 ),
 ( #3757, #9448, #8195, #12274, #17753, #17842, #13547, #15080, #7931, #6647, #13465, #9363, #3934, #5362, #12175, #13721, #5452, #10795, #14986, #2664, #13633, #10881, #12353, #8273, #4112, #9621, #15173, #12536, #16811, #1756, #5904, #4286, #4377, #11428, #14265, #13995, #9703, #11144, #8635, #398, #10068, #16909, #4463, #4203, #16992, #8546, #14078, #1482, #5717, #481, #15253, #7012, #5628, #5810, #14165, #5990, #12803, #7286, #11331, #7383, #301, #9889, #4548, #15441, #16714, #9793, #1664, #1578, #13891, #7198, #120, #15617, #7111, #12625, #3106, #16626, #2924, #3195, #8734, #1854, #15345, #8458, #12898, #2830, #9978, #8360, #208, #11234, #3023, #12708, #15525, #17467, #14446, #13351, #4998, #6183, #10165, #4729, #7461, #3293, #14718, #929, #9091, #14355, #10341, #8910, #3654, #2302, #12985, #10253, #1941, #747, #7820, #570, #4907, #11516, #2029, #9174, #11705, #3566, #6274, #14633, #10435, #15994, #11794, #2214, #8824, #17085, #7552, #17276, #836, #6089, #4812, #13076, #4640, #15718, #11617, #15894, #3468, #17182, #7727, #13254, #6365, #15802, #11888, #10525, #16086, #3377, #660, #8999, #17373, #14544, #2126 ) ),
 .UNSPECIFIED., .F., .F., .T. ) 
 B_SPLINE_SURFACE_WITH_KNOTS ( ( 2, 2 ),
 ( 3, 2, 2, 2, 2, 2, 2, 2, 2, 2, 2, 2, 2, 2, 2, 2, 2, 2, 2, 2, 2, 2, 2, 2, 2, 2, 2, 2, 2, 2, 2, 2, 2, 2, 2, 2, 2, 2, 2, 2, 2, 2, 2, 2, 2, 2, 2, 2, 2, 2, 2, 2, 2, 2, 2, 2, 2, 2, 2, 2, 2, 2, 2, 2, 2, 2, 2, 2, 2, 2, 2, 2, 2, 2, 2, 2, 3 ),
 ( 0.000000000000000000, 1.000000000000000000 ),
 ( 0.000000000000000000, 0.01282051282051282007, 0.02564102564102564014, 0.03846153846153846367, 0.05128205128205128027, 0.06410256410256409687, 0.07692307692307692735, 0.08974358974358974395, 0.1025641025641025605, 0.1153846153846153910, 0.1282051282051281937, 0.1410256410256410242, 0.1538461538461538547, 0.1666666666666666574, 0.1794871794871794879, 0.1923076923076923184, 0.2051282051282051211, 0.2179487179487179516, 0.2307692307692307820, 0.2435897435897435848, 0.2564102564102563875, 0.2692307692307692180, 0.2820512820512820484, 0.2948717948717948789, 0.3076923076923077094, 0.3205128205128205399, 0.3333333333333333148, 0.3461538461538461453, 0.3589743589743589758, 0.3717948717948718063, 0.3846153846153846367, 0.3974358974358974117, 0.4102564102564102422, 0.4230769230769230727, 0.4358974358974359031, 0.4487179487179487336, 0.4615384615384615641, 0.4743589743589743390, 0.4871794871794871695, 0.5000000000000000000, 0.5128205128205127750, 0.5256410256410256610, 0.5384615384615384359, 0.5512820512820513219, 0.5641025641025640969, 0.5769230769230768718, 0.5897435897435897578, 0.6025641025641025328, 0.6153846153846154188, 0.6282051282051281937, 0.6410256410256410797, 0.6538461538461538547, 0.6666666666666666297, 0.6794871794871795156, 0.6923076923076922906, 0.7051282051282051766, 0.7179487179487179516, 0.7307692307692307265, 0.7435897435897436125, 0.7564102564102563875, 0.7692307692307692735, 0.7820512820512820484, 0.7948717948717948234, 0.8076923076923077094, 0.8205128205128204844, 0.8333333333333333703, 0.8461538461538461453, 0.8589743589743589203, 0.8717948717948718063, 0.8846153846153845812, 0.8974358974358974672, 0.9102564102564102422, 0.9230769230769231282, 0.9358974358974359031, 0.9487179487179486781, 0.9615384615384615641, 0.9690837704703162414 ),
 .UNSPECIFIED. ) 
 GEOMETRIC_REPRESENTATION_ITEM ( )  RATIONAL_B_SPLINE_SURFACE ( (
 ( 1.000000000000000000, 0.8660254037844387076, 1.000000000000000000, 0.8660254037844387076, 1.000000000000000000, 0.8660254037844387076, 1.000000000000000000, 0.8660254037844387076, 1.000000000000000000, 0.8660254037844387076, 1.000000000000000000, 0.8660254037844387076, 1.000000000000000000, 0.8660254037844387076, 1.000000000000000000, 0.8660254037844387076, 1.000000000000000000, 0.8660254037844387076, 1.000000000000000000, 0.8660254037844387076, 1.000000000000000000, 0.8660254037844387076, 1.000000000000000000, 0.8660254037844387076, 1.000000000000000000, 0.8660254037844387076, 1.000000000000000000, 0.8660254037844387076, 1.000000000000000000, 0.8660254037844387076, 1.000000000000000000, 0.8660254037844387076, 1.000000000000000000, 0.8660254037844387076, 1.000000000000000000, 0.8660254037844387076, 1.000000000000000000, 0.8660254037844387076, 1.000000000000000000, 0.8660254037844387076, 1.000000000000000000, 0.8660254037844387076, 1.000000000000000000, 0.8660254037844387076, 1.000000000000000000, 0.8660254037844387076, 1.000000000000000000, 0.8660254037844387076, 1.000000000000000000, 0.8660254037844387076, 1.000000000000000000, 0.8660254037844387076, 1.000000000000000000, 0.8660254037844387076, 1.000000000000000000, 0.8660254037844387076, 1.000000000000000000, 0.8660254037844387076, 1.000000000000000000, 0.8660254037844387076, 1.000000000000000000, 0.8660254037844387076, 1.000000000000000000, 0.8660254037844387076, 1.000000000000000000, 0.8660254037844387076, 1.000000000000000000, 0.8660254037844387076, 1.000000000000000000, 0.8660254037844387076, 1.000000000000000000, 0.8660254037844387076, 1.000000000000000000, 0.8660254037844387076, 1.000000000000000000, 0.8660254037844387076, 1.000000000000000000, 0.8660254037844387076, 1.000000000000000000, 0.8660254037844387076, 1.000000000000000000, 0.8660254037844387076, 1.000000000000000000, 0.8660254037844387076, 1.000000000000000000, 0.8660254037844387076, 1.000000000000000000, 0.8660254037844387076, 1.000000000000000000, 0.8660254037844387076, 1.000000000000000000, 0.8660254037844387076, 1.000000000000000000, 0.8660254037844387076, 1.000000000000000000, 0.8660254037844387076, 1.000000000000000000, 0.8660254037844387076, 1.000000000000000000, 0.8660254037844387076, 1.000000000000000000, 0.8660254037844387076, 1.000000000000000000, 0.8660254037844387076, 1.000000000000000000, 0.8660254037844387076, 1.000000000000000000, 0.8660254037844387076, 1.000000000000000000, 0.8660254037844387076, 1.000000000000000000, 0.8660254037844387076, 1.000000000000000000, 0.8660254037844387076, 1.000000000000000000, 0.8660254037844387076, 1.000000000000000000, 0.8660254037844387076, 1.000000000000000000, 0.8660254037844387076, 1.000000000000000000, 0.8660254037844387076, 1.000000000000000000, 0.8660254037844387076, 1.000000000000000000, 0.8660254037844387076, 1.000000000000000000, 0.8660254037844387076, 1.000000000000000000, 0.8660254037844387076, 1.000000000000000000, 0.8660254037844387076, 1.000000000000000000, 0.8660254037844387076, 1.000000000000000000, 0.8660254037844387076, 1.000000000000000000, 0.8660254037844387076, 1.000000000000000000, 0.8660254037844387076, 1.000000000000000000, 0.8660254037844387076, 1.000000000000000000, 0.8660254037844387076, 1.000000000000000000, 0.8660254037844387076, 1.000000000000000000, 0.8660254037844387076, 1.000000000000000000, 0.8660254037844387076, 1.000000000000000000, 0.9211513820375816231, 0.9351129643698559146),
 ( 1.000000000000000000, 0.8660254037844387076, 1.000000000000000000, 0.8660254037844387076, 1.000000000000000000, 0.8660254037844387076, 1.000000000000000000, 0.8660254037844387076, 1.000000000000000000, 0.8660254037844387076, 1.000000000000000000, 0.8660254037844387076, 1.000000000000000000, 0.8660254037844387076, 1.000000000000000000, 0.8660254037844387076, 1.000000000000000000, 0.8660254037844387076, 1.000000000000000000, 0.8660254037844387076, 1.000000000000000000, 0.8660254037844387076, 1.000000000000000000, 0.8660254037844387076, 1.000000000000000000, 0.8660254037844387076, 1.000000000000000000, 0.8660254037844387076, 1.000000000000000000, 0.8660254037844387076, 1.000000000000000000, 0.8660254037844387076, 1.000000000000000000, 0.8660254037844387076, 1.000000000000000000, 0.8660254037844387076, 1.000000000000000000, 0.8660254037844387076, 1.000000000000000000, 0.8660254037844387076, 1.000000000000000000, 0.8660254037844387076, 1.000000000000000000, 0.8660254037844387076, 1.000000000000000000, 0.8660254037844387076, 1.000000000000000000, 0.8660254037844387076, 1.000000000000000000, 0.8660254037844387076, 1.000000000000000000, 0.8660254037844387076, 1.000000000000000000, 0.8660254037844387076, 1.000000000000000000, 0.8660254037844387076, 1.000000000000000000, 0.8660254037844387076, 1.000000000000000000, 0.8660254037844387076, 1.000000000000000000, 0.8660254037844387076, 1.000000000000000000, 0.8660254037844387076, 1.000000000000000000, 0.8660254037844387076, 1.000000000000000000, 0.8660254037844387076, 1.000000000000000000, 0.8660254037844387076, 1.000000000000000000, 0.8660254037844387076, 1.000000000000000000, 0.8660254037844387076, 1.000000000000000000, 0.8660254037844387076, 1.000000000000000000, 0.8660254037844387076, 1.000000000000000000, 0.8660254037844387076, 1.000000000000000000, 0.8660254037844387076, 1.000000000000000000, 0.8660254037844387076, 1.000000000000000000, 0.8660254037844387076, 1.000000000000000000, 0.8660254037844387076, 1.000000000000000000, 0.8660254037844387076, 1.000000000000000000, 0.8660254037844387076, 1.000000000000000000, 0.8660254037844387076, 1.000000000000000000, 0.8660254037844387076, 1.000000000000000000, 0.8660254037844387076, 1.000000000000000000, 0.8660254037844387076, 1.000000000000000000, 0.8660254037844387076, 1.000000000000000000, 0.8660254037844387076, 1.000000000000000000, 0.8660254037844387076, 1.000000000000000000, 0.8660254037844387076, 1.000000000000000000, 0.8660254037844387076, 1.000000000000000000, 0.8660254037844387076, 1.000000000000000000, 0.8660254037844387076, 1.000000000000000000, 0.8660254037844387076, 1.000000000000000000, 0.8660254037844387076, 1.000000000000000000, 0.8660254037844387076, 1.000000000000000000, 0.8660254037844387076, 1.000000000000000000, 0.8660254037844387076, 1.000000000000000000, 0.8660254037844387076, 1.000000000000000000, 0.8660254037844387076, 1.000000000000000000, 0.8660254037844387076, 1.000000000000000000, 0.8660254037844387076, 1.000000000000000000, 0.8660254037844387076, 1.000000000000000000, 0.8660254037844387076, 1.000000000000000000, 0.8660254037844387076, 1.000000000000000000, 0.8660254037844387076, 1.000000000000000000, 0.8660254037844387076, 1.000000000000000000, 0.8660254037844387076, 1.000000000000000000, 0.8660254037844387076, 1.000000000000000000, 0.8660254037844387076, 1.000000000000000000, 0.8660254037844387076, 1.000000000000000000, 0.9211513820375816231, 0.9351129643698559146) ) ) 
 REPRESENTATION_ITEM ( '' )  SURFACE ( )  );
#3457=ORIENTED_EDGE ( 'NONE', *, *, #47, .T. ) ;
#3459=CARTESIAN_POINT ( 'NONE',  ( 30.12381574833269937, -2.526612381163247267, -4.705209693361161349 ) ) ;
#3460=ORIENTED_EDGE ( 'NONE', *, *, #17909, .T. ) ;
#3461=AXIS2_PLACEMENT_3D ( 'NONE', #15762, #11282, #4331 ) ;
#3465=CARTESIAN_POINT ( 'NONE',  ( 28.08810621022444920, -4.652786776866828511, -3.627061608673664672 ) ) ;
#3466=VECTOR ( 'NONE', #2832, 1000.000000000000000 ) ;
#3468=CARTESIAN_POINT ( 'NONE',  ( 26.35439372113758694, -4.861664893681965083, -7.939653947423662039 ) ) ;
#3469=CARTESIAN_POINT ( 'NONE',  ( 28.09001152836988524, -6.106370808549102414, -8.283357778048664244 ) ) ;
#3473=VECTOR ( 'NONE', #2224, 1000.000000000000000 ) ;
#3476=ORIENTED_EDGE ( 'NONE', *, *, #826, .T. ) ;
#3479=CARTESIAN_POINT ( 'NONE',  ( 8.632250723006720250, -18.84644399697197770, -16.84735068286506987 ) ) ;
#3483=CARTESIAN_POINT ( 'NONE',  ( 45.50000000000000000, -16.03270077640482683, -2.787981825772262390 ) ) ;
#3484=CARTESIAN_POINT ( 'NONE',  ( 33.54323074294813267, -5.249493066516778050, -7.939653947423662927 ) ) ;
#3487=CARTESIAN_POINT ( 'NONE',  ( 28.13873763417254992, -3.192873105281056390, -3.283357778048662023 ) ) ;
#3488=DIRECTION ( 'NONE',  ( 0.000000000000000000, 0.000000000000000000, -1.000000000000000000 ) ) ;
#3495=CARTESIAN_POINT ( 'NONE',  ( 26.01652455409633902, -4.902371455920928156, -5.783357778048663356 ) ) ;
#3497=VERTEX_POINT ( 'NONE', #9367 ) ;
#3498=EDGE_LOOP ( 'NONE', ( #17288, #16593, #4447, #7418 ) ) ;
#3502=( NAMED_UNIT ( * ) SI_UNIT ( $, .STERADIAN. ) SOLID_ANGLE_UNIT ( ) );
#3509=CARTESIAN_POINT ( 'NONE',  ( 31.97277696464621854, -6.702839660918840536, -5.783357778048663356 ) ) ;
#3512=CARTESIAN_POINT ( 'NONE',  ( 28.45891156537951971, -2.090033060632186412, -5.783357778048670461 ) ) ;
#3513=DIRECTION ( 'NONE',  ( 0.000000000000000000, 0.000000000000000000, 1.000000000000000000 ) ) ;
#3516=DIRECTION ( 'NONE',  ( 0.9928203230275510771, 0.1196152422706614621, -0.000000000000000000 ) ) ;
#3523=CYLINDRICAL_SURFACE ( 'NONE', #14981, 2.499999999999999112 ) ;
#3529=CARTESIAN_POINT ( 'NONE',  ( -22.62145100412528009, -22.46994790986326151, -15.00472644746570694 ) ) ;
#3534=VECTOR ( 'NONE', #16708, 1000.000000000000000 ) ;
#3542=EDGE_CURVE ( 'NONE', #11419, #8674, #9475, .T. ) ;
#3543=CARTESIAN_POINT ( 'NONE',  ( 26.88845778707760914, -3.543379655034240905, -7.939653947423660263 ) ) ;
#3546=CYLINDRICAL_SURFACE ( 'NONE', #8058, 2.499999999999999112 ) ;
#3547=CARTESIAN_POINT ( 'NONE',  ( 31.61111609099199171, -1.710254666422835745, -5.783357778048662468 ) ) ;
#3548=EDGE_CURVE ( 'NONE', #8691, #17122, #15328, .T. ) ;
#3550=PLANE ( 'NONE',  #12971 ) ;
#3551=CARTESIAN_POINT ( 'NONE',  ( 31.30154412293507349, -3.011689903141150815, -7.939653947423660263 ) ) ;
#3558=DIRECTION ( 'NONE',  ( -1.000000000000000000, 0.000000000000000000, 0.000000000000000000 ) ) ;
#3559=CARTESIAN_POINT ( 'NONE',  ( 25.84832697747033592, -3.506312147857040706, -7.581167935121603918 ) ) ;
#3560=DIRECTION ( 'NONE',  ( -1.000000000000000000, 0.000000000000000000, 0.000000000000000000 ) ) ;
#3562=VECTOR ( 'NONE', #871, 1000.000000000000227 ) ;
#3563=CARTESIAN_POINT ( 'NONE',  ( 32.33415724766913257, -1.960501102408027219, -4.533357778048659803 ) ) ;
#3566=CARTESIAN_POINT ( 'NONE',  ( 27.50150540219088313, -5.977401655418042914, -3.627061608673667781 ) ) ;
#3575=AXIS2_PLACEMENT_3D ( 'NONE', #5095, #17575, #9272 ) ;
#3579=CARTESIAN_POINT ( 'NONE',  ( 9.099998387031005720, -19.29508120620799971, -6.000000000000000000 ) ) ;
#3585=CARTESIAN_POINT ( 'NONE',  ( 32.19919549706052209, -6.038393303862174655, -4.705209693361169343 ) ) ;
#3588=CARTESIAN_POINT ( 'NONE',  ( 27.50829672905005907, -3.268828784122927100, -3.283357778048662023 ) ) ;
#3610=CARTESIAN_POINT ( 'NONE',  ( 32.69811611091622439, -2.216460025892273311, -6.861505862736158257 ) ) ;
#3616=CYLINDRICAL_SURFACE ( 'NONE', #8624, 5.500000000000000888 ) ;
#3621=ORIENTED_EDGE ( 'NONE', *, *, #17240, .T. ) ;
#3626=PLANE ( 'NONE',  #7195 ) ;
#3628=DIRECTION ( 'NONE',  ( 1.000000000000000000, 0.000000000000000000, 0.000000000000000000 ) ) ;
#3629=CARTESIAN_POINT ( 'NONE',  ( 27.24868051476284236, -2.235842002054281075, -6.453230759126464378 ) ) ;
#3631=FACE_OUTER_BOUND ( 'NONE', #17920, .T. ) ;
#3633=CARTESIAN_POINT ( 'NONE',  ( 45.00000000000000711, -19.03270077640483038, -0.5379818257722508434 ) ) ;
#3635=CARTESIAN_POINT ( 'NONE',  ( 29.70732014299206369, -2.276983097582480742, -7.033357778048658027 ) ) ;
#3638=CARTESIAN_POINT ( 'NONE',  ( 27.12505156253147476, -7.276697974355294640, -5.783357778048668685 ) ) ;
#3645=CARTESIAN_POINT ( 'NONE',  ( 31.71314141467879111, -4.216041623526076698, -3.627061608673664672 ) ) ;
#3646=ORIENTED_EDGE ( 'NONE', *, *, #3369, .F. ) ;
#3648=CARTESIAN_POINT ( 'NONE',  ( 45.00000000000000711, -19.03270077640482683, -10.53798182577225084 ) ) ;
#3650=CARTESIAN_POINT ( 'NONE',  ( -23.00000000000000000, -16.21813761408365195, -13.00000000000000178 ) ) ;
#3652=CARTESIAN_POINT ( 'NONE',  ( 32.53688598753899441, -6.297517047505613697, -7.033357778048666908 ) ) ;
#3654=CARTESIAN_POINT ( 'NONE',  ( 28.25893984004492765, -6.513116296623863377, -4.705209693361168455 ) ) ;
#3659=CARTESIAN_POINT ( 'NONE',  ( -34.91600907648203389, -11.88801210197604341, -12.00000000000000000 ) ) ;
#3664=CARTESIAN_POINT ( 'NONE',  ( 33.44685390376565692, -4.007163506710925027, -7.939653947423662039 ) ) ;
#3666=CARTESIAN_POINT ( 'NONE',  ( 29.26075783691881682, -2.330785036554694489, -4.533357778048659803 ) ) ;
#3672=EDGE_CURVE ( 'NONE', #15335, #14228, #10617, .T. ) ;
#3674=CARTESIAN_POINT ( 'NONE',  ( 29.25000000000000000, -16.21813761408365195, -13.37255996287876236 ) ) ;
#3676=AXIS2_PLACEMENT_3D ( 'NONE', #13531, #6629, #12155 ) ;
#3685=CARTESIAN_POINT ( 'NONE',  ( 33.15485366002904755, -6.560422763297783177, -5.783357778048663356 ) ) ;
#3686=CARTESIAN_POINT ( 'NONE',  ( 32.19919549706052209, -6.038393303862174655, -4.705209693361169343 ) ) ;
#3703=DIRECTION ( 'NONE',  ( -1.000000000000000000, 0.000000000000000000, 0.000000000000000000 ) ) ;
#3704=AXIS2_PLACEMENT_3D ( 'NONE', #17279, #401, #10071 ) ;
#3710=LINE ( 'NONE', #2006, #2400 ) ;
#3711=CARTESIAN_POINT ( 'NONE',  ( 27.12922144900085186, -2.887401855662130146, -4.705209693361160461 ) ) ;
#3712=CARTESIAN_POINT ( 'NONE',  ( 33.86058074732183343, -3.957317592522819005, -3.455209693361164902 ) ) ;
#3714=EDGE_LOOP ( 'NONE', ( #7431, #1956, #48, #9036, #10400, #4315 ) ) ;
#3716=CARTESIAN_POINT ( 'NONE',  ( 32.80318959510331212, -2.203800746085299522, -4.705209693361160461 ) ) ;
#3720=VECTOR ( 'NONE', #16876, 1000.000000000000000 ) ;
#3722=AXIS2_PLACEMENT_3D ( 'NONE', #14383, #7673, #505 ) ;
#3723=ORIENTED_EDGE ( 'NONE', *, *, #11795, .T. ) ;
#3724=CARTESIAN_POINT ( 'NONE',  ( 29.38468146192651886, -6.677295441714964142, -7.033357778048666908 ) ) ;
#3725=CARTESIAN_POINT ( 'NONE',  ( 31.39792096211754924, -4.254019462947003838, -7.939653947423662039 ) ) ;
#3726=CARTESIAN_POINT ( 'NONE',  ( 21.42601376483257880, 2.765314980223224417, -12.00000000000000000 ) ) ;
#3728=CARTESIAN_POINT ( 'NONE',  ( 28.82057243903374655, -7.082618055128190093, -5.783357778048668685 ) ) ;
#3732=CARTESIAN_POINT ( 'NONE',  ( 32.38298487551052318, -4.135338714860305132, -8.283357778048662468 ) ) ;
#3733=ORIENTED_EDGE ( 'NONE', *, *, #443, .F. ) ;
#3734=CARTESIAN_POINT ( 'NONE',  ( 33.30246708102489350, -5.905470865888903020, -4.705209693361168455 ) ) ;
#3736=CARTESIAN_POINT ( 'NONE',  ( 3.248936832696173393, -28.97437970944926633, -17.00000000000000000 ) ) ;
#3739=EDGE_CURVE ( 'NONE', #12847, #11807, #4647, .T. ) ;
#3742=EDGE_LOOP ( 'NONE', ( #11340, #14046 ) ) ;
#3749=( NAMED_UNIT ( * ) SI_UNIT ( $, .STERADIAN. ) SOLID_ANGLE_UNIT ( ) );
#3753=DIRECTION ( 'NONE',  ( 0.9928203230275510771, 0.1196152422706614621, -0.000000000000000000 ) ) ;
#3754=ORIENTED_EDGE ( 'NONE', *, *, #2082, .F. ) ;
#3757=CARTESIAN_POINT ( 'NONE',  ( 33.60446413004628141, -3.988174587000466342, -3.627061608673664672 ) ) ;
#3763=ADVANCED_FACE ( 'NONE', ( #13176 ), #10173, .T. ) ;
#3765=CARTESIAN_POINT ( 'NONE',  ( 25.76872643656706074, -21.83605427490913797, -14.29305147543152366 ) ) ;
#3778=CARTESIAN_POINT ( 'NONE',  ( 30.29464937815318493, -4.386941900920275472, -7.939653947423662039 ) ) ;
#3782=VECTOR ( 'NONE', #6710, 1000.000000000000227 ) ;
#3786=CARTESIAN_POINT ( 'NONE',  ( 27.95866967485789090, -6.122194908100387245, -3.283357778048667797 ) ) ;
#3787=CARTESIAN_POINT ( 'NONE',  ( 32.49625839967270480, -6.639770485940693412, -5.113484796970860558 ) ) ;
#3789=B_SPLINE_CURVE_WITH_KNOTS ( 'NONE', 3,
 ( #2183, #4784, #13043, #14413 ),
 .UNSPECIFIED., .F., .F.,
 ( 4, 4 ),
 ( 0.000000000000000000, 0.0006487028241592422868 ),
 .UNSPECIFIED. ) ;
#3790=AXIS2_PLACEMENT_3D ( 'NONE', #15708, #11701, #3558 ) ;
#3791=ORIENTED_EDGE ( 'NONE', *, *, #5183, .T. ) ;
#3794=ORIENTED_EDGE ( 'NONE', *, *, #13595, .F. ) ;
#3804=CARTESIAN_POINT ( 'NONE',  ( 29.62480591732145996, -4.467644809586046151, -3.283357778048664688 ) ) ;
#3809=FACE_OUTER_BOUND ( 'NONE', #5634, .T. ) ;
#3814=CARTESIAN_POINT ( 'NONE',  ( 30.40841950734487753, -3.119293781500474427, -3.627061608673662008 ) ) ;
#3821=VECTOR ( 'NONE', #4440, 1000.000000000000114 ) ;
#3822=CARTESIAN_POINT ( 'NONE',  ( 27.73357241910951743, -6.576412695658750529, -6.861505862736166250 ) ) ;
#3825=B_SPLINE_CURVE_WITH_KNOTS ( 'NONE', 3,
 ( #5439, #383, #15601, #6070, #7183, #10146, #15697, #11599, #17165, #10485, #4532, #15512, #3009, #11412, #14342, #5798, #3177, #3093 ),
 .UNSPECIFIED., .F., .F.,
 ( 4, 2, 2, 2, 2, 2, 2, 2, 4 ),
 ( 0.000000000000000000, 0.0005710890023745246154, 0.001142178004749049231, 0.001713267007123573955, 0.002284356009498098462, 0.002855445011872622969, 0.003426534014247147909, 0.003997623016621672416, 0.004568712018996196923 ),
 .UNSPECIFIED. ) ;
#3832=CARTESIAN_POINT ( 'NONE',  ( 32.92339180097568629, -5.524043937428110063, -3.283357778048667797 ) ) ;
#3833=CARTESIAN_POINT ( 'NONE',  ( 33.14902674121363901, -1.535163666906202318, -5.783357778048658027 ) ) ;
#3835=CARTESIAN_POINT ( 'NONE',  ( 25.71748644841968456, -2.420320648352051851, -5.783357778048663356 ) ) ;
#3843=CYLINDRICAL_SURFACE ( 'NONE', #5502, 2.499999999999999112 ) ;
#3846=( NAMED_UNIT ( * ) PLANE_ANGLE_UNIT ( ) SI_UNIT ( $, .RADIAN. ) );
#3847=ADVANCED_FACE ( 'NONE', ( #12697, #386 ), #15605, .F. ) ;
#3852=CARTESIAN_POINT ( 'NONE',  ( 25.37303892199676270, -2.799178389412888546, -7.033357778048658027 ) ) ;
#3853=CYLINDRICAL_SURFACE ( 'NONE', #5749, 95.00000000000000000 ) ;
#3854=DIRECTION ( 'NONE',  ( -0.000000000000000000, -0.000000000000000000, -1.000000000000000000 ) ) ;
#3864=ORIENTED_EDGE ( 'NONE', *, *, #1850, .F. ) ;
#3869=CARTESIAN_POINT ( 'NONE',  ( 30.92509028327567933, -4.310986222078405206, -7.939653947423662039 ) ) ;
#3871=VECTOR ( 'NONE', #5874, 1000.000000000000114 ) ;
#3876=EDGE_LOOP ( 'NONE', ( #12501, #917, #4888, #3375 ) ) ;
#3877=DIRECTION ( 'NONE',  ( 0.000000000000000000, 0.000000000000000000, -1.000000000000000000 ) ) ;
#3893=CARTESIAN_POINT ( 'NONE',  ( 21.42418217458643070, -10.16661967303011771, -15.24537580551290183 ) ) ;
#3894=CARTESIAN_POINT ( 'NONE',  ( 23.00000000000000000, -16.21813761408365195, 0.000000000000000000 ) ) ;
#3896=CARTESIAN_POINT ( 'NONE',  ( 30.17635249042624679, -2.520282741259753045, -6.861505862736158257 ) ) ;
#3898=ORIENTED_EDGE ( 'NONE', *, *, #4866, .F. ) ;
#3901=LINE ( 'NONE', #12237, #1417 ) ;
#3904=ORIENTED_EDGE ( 'NONE', *, *, #3183, .T. ) ;
#3905=ORIENTED_EDGE ( 'NONE', *, *, #10233, .F. ) ;
#3908=CARTESIAN_POINT ( 'NONE',  ( 26.97161122272022382, -2.906390775372597712, -4.705209693361161349 ) ) ;
#3915=CARTESIAN_POINT ( 'NONE',  ( 30.17644170758179101, -4.401183590806859947, -3.283357778048664688 ) ) ;
#3917=CARTESIAN_POINT ( 'NONE',  ( 33.17547354829333273, -5.293800545841212291, -3.627061608673667781 ) ) ;
#3919=CARTESIAN_POINT ( 'NONE',  ( 32.14656953781143756, -4.163822094218565972, -3.283357778048664688 ) ) ;
#3920=CYLINDRICAL_SURFACE ( 'NONE', #14730, 2.499999999999999112 ) ;
#3927=EDGE_LOOP ( 'NONE', ( #8850, #16570, #12153, #14710, #7826, #12028 ) ) ;
#3929=CARTESIAN_POINT ( 'NONE',  ( -27.11337801594864061, -11.49512195020015604, -13.95421129451976050 ) ) ;
#3931=PRESENTATION_STYLE_ASSIGNMENT (( #16368 ) ) ;
#3932=CARTESIAN_POINT ( 'NONE',  ( 31.04338717100262102, -6.177645381738930297, -6.861505862736167138 ) ) ;
#3934=CARTESIAN_POINT ( 'NONE',  ( 32.97402322492378346, -4.064130265842336165, -3.627061608673664672 ) ) ;
#3938=EDGE_CURVE ( 'NONE', #16041, #16203, #17217, .T. ) ;
#3939=CARTESIAN_POINT ( 'NONE',  ( 28.91480295676398171, -18.24795679052564168, -13.46730161501605316 ) ) ;
#3942=EDGE_CURVE ( 'NONE', #3060, #2784, #16108, .T. ) ;
#3944=DIRECTION ( 'NONE',  ( -0.000000000000000000, -0.000000000000000000, -1.000000000000000000 ) ) ;
#3949=CARTESIAN_POINT ( 'NONE',  ( 33.32864623319426300, -4.021405196597508613, -3.283357778048664688 ) ) ;
#3950=CARTESIAN_POINT ( 'NONE',  ( 31.02146712245815507, -5.553315781884258229, -7.939653947423664704 ) ) ;
#3963=ORIENTED_EDGE ( 'NONE', *, *, #1484, .T. ) ;
#3968=ORIENTED_EDGE ( 'NONE', *, *, #5286, .T. ) ;
#3970=ADVANCED_FACE ( 'NONE', ( #6563 ), #7933, .F. ) ;
#3973=FACE_OUTER_BOUND ( 'NONE', #14850, .T. ) ;
#3975=CARTESIAN_POINT ( 'NONE',  ( 13.00000000000000178, 0.000000000000000000, -12.00000000000000000 ) ) ;
#3977=CARTESIAN_POINT ( 'NONE',  ( 26.01652455409633902, -4.902371455920928156, -5.783357778048663356 ) ) ;
#3979=CARTESIAN_POINT ( 'NONE',  ( 22.62608969754382215, -9.966271075498049470, -15.00374444583767897 ) ) ;
#3981=CARTESIAN_POINT ( 'NONE',  ( 31.41531425212677675, -1.744041783721344219, -5.783357778048658027 ) ) ;
#3989=CARTESIAN_POINT ( 'NONE',  ( 30.23341599105502908, -5.648260380436596506, -7.939653947423662927 ) ) ;
#3990=CARTESIAN_POINT ( 'NONE',  ( 25.83973938098743517, -3.435034105423886874, -4.207126410816434792 ) ) ;
#3994=CARTESIAN_POINT ( 'NONE',  ( 28.13873763417255347, -3.192873105281056390, -3.283357778048662023 ) ) ;
#3995=CARTESIAN_POINT ( 'NONE',  ( 45.00000000000000711, -16.03270077640482683, -0.5379818257722508434 ) ) ;
#3997=CARTESIAN_POINT ( 'NONE',  ( 29.70732014299206369, -2.276983097582480742, -7.033357778048658027 ) ) ;
#3998=( BOUNDED_CURVE ( )  B_SPLINE_CURVE ( 2, ( #4465, #1856, #4730, #2127, #15618, #3469, #17277, #9000, #3196 ),
 .UNSPECIFIED., .F., .T. ) 
 B_SPLINE_CURVE_WITH_KNOTS ( ( 3, 2, 2, 2, 3 ),
 ( 0.7115384615384615641, 0.7179487179487179516, 0.7307692307692307265, 0.7435897435897436125, 0.7500000000000000000 ),
 .UNSPECIFIED. ) 
 CURVE ( )  GEOMETRIC_REPRESENTATION_ITEM ( )  RATIONAL_B_SPLINE_CURVE ( ( 0.9330127018922194093, 0.9330127018922194093, 1.000000000000000000, 0.8660254037844387076, 1.000000000000000000, 0.8660254037844387076, 1.000000000000000000, 0.9330127018922194093, 0.9330127018922194093 ) ) 
 REPRESENTATION_ITEM ( '' )  );
#4001=CARTESIAN_POINT ( 'NONE',  ( 32.14213199643172914, -2.910415664685331638, -3.627061608673662896 ) ) ;
#4004=CARTESIAN_POINT ( 'NONE',  ( 32.57506351453486815, -6.630276025878011126, -5.113484796970860558 ) ) ;
#4005=DIRECTION ( 'NONE',  ( 0.000000000000000000, 0.000000000000000000, 1.000000000000000000 ) ) ;
#4009=DIRECTION ( 'NONE',  ( -1.000000000000000000, 0.000000000000000000, 0.000000000000000000 ) ) ;
#4014=CARTESIAN_POINT ( 'NONE',  ( 29.52399153675929355, -1.971908820246954130, -5.783357778048658915 ) ) ;
#4018=( BOUNDED_CURVE ( )  B_SPLINE_CURVE ( 2, ( #11431, #12987, #9093, #16995, #11619, #10255, #3197, #8736, #13079 ),
 .UNSPECIFIED., .F., .F. ) 
 B_SPLINE_CURVE_WITH_KNOTS ( ( 3, 2, 2, 2, 3 ),
 ( 0.09615384615384617306, 0.1025641025641025605, 0.1153846153846153910, 0.1282051282051281937, 0.1346153846153846367 ),
 .UNSPECIFIED. ) 
 CURVE ( )  GEOMETRIC_REPRESENTATION_ITEM ( )  RATIONAL_B_SPLINE_CURVE ( ( 0.9330127018922194093, 0.9330127018922196314, 1.000000000000000000, 0.8660254037844387076, 1.000000000000000000, 0.8660254037844387076, 1.000000000000000000, 0.9330127018922190762, 0.9330127018922194093 ) ) 
 REPRESENTATION_ITEM ( '' )  );
#4019=CARTESIAN_POINT ( 'NONE',  ( 25.59340017005574097, -5.757764245108966783, -8.283357778048664244 ) ) ;
#4023=VECTOR ( 'NONE', #14123, 1000.000000000000000 ) ;
#4029=ORIENTED_EDGE ( 'NONE', *, *, #11209, .T. ) ;
#4030=ORIENTED_EDGE ( 'NONE', *, *, #16936, .F. ) ;
#4035=CARTESIAN_POINT ( 'NONE',  ( 30.17635249042624679, -2.520282741259753045, -6.861505862736158257 ) ) ;
#4044=LINE ( 'NONE', #6511, #11214 ) ;
#4060=DIRECTION ( 'NONE',  ( 0.6000000000000001998, 0.7999999999999999334, 0.000000000000000000 ) ) ;
#4064=DIRECTION ( 'NONE',  ( -0.1196152422706611984, 0.9928203230275510771, 0.000000000000000000 ) ) ;
#4067=CARTESIAN_POINT ( 'NONE',  ( 29.80442540930208750, -6.953886339277345563, -5.783357778048669573 ) ) ;
#4072=DIRECTION ( 'NONE',  ( -0.9928203230275514102, -0.1196152422706598939, 0.000000000000000000 ) ) ;
#4076=CARTESIAN_POINT ( 'NONE',  ( 28.25893984004492765, -6.513116296623863377, -4.705209693361168455 ) ) ;
#4081=FACE_OUTER_BOUND ( 'NONE', #782, .T. ) ;
#4083=ADVANCED_FACE ( 'NONE', ( #8197 ), #15347, .T. ) ;
#4086=CARTESIAN_POINT ( 'NONE',  ( 29.77118727536320719, -5.903822331637461396, -3.283357778048667797 ) ) ;
#4087=VECTOR ( 'NONE', #12683, 1000.000000000000000 ) ;
#4092=CARTESIAN_POINT ( 'NONE',  ( 27.92859066579839222, -3.218191664895003523, -8.283357778048660691 ) ) ;
#4101=CARTESIAN_POINT ( 'NONE',  ( 0.000000000000000000, 0.000000000000000000, -12.00000000000000000 ) ) ;
#4104=CARTESIAN_POINT ( 'NONE',  ( 6.935828204433864386, -17.68137362934027124, -16.94363565911716663 ) ) ;
#4108=CARTESIAN_POINT ( 'NONE',  ( 31.06530721954707985, -6.801974981593605918, -5.783357778048669573 ) ) ;
#4111=ORIENTED_EDGE ( 'NONE', *, *, #17646, .F. ) ;
#4112=CARTESIAN_POINT ( 'NONE',  ( 32.34358231980129261, -4.140085944684206432, -3.627061608673664672 ) ) ;
#4118=CARTESIAN_POINT ( 'NONE',  ( 25.01460733971720529, -22.13799366862516038, -14.47321228143779415 ) ) ;
#4124=ORIENTED_EDGE ( 'NONE', *, *, #5854, .T. ) ;
#4126=CARTESIAN_POINT ( 'NONE',  ( 28.74176732417158320, -7.092112515190875044, -5.783357778048657138 ) ) ;
#4127=ORIENTED_EDGE ( 'NONE', *, *, #14940, .F. ) ;
#4129=( BOUNDED_CURVE ( )  B_SPLINE_CURVE ( 2, ( #16649, #3047, #2775, #141, #5836, #13915, #9915, #8296, #12733 ),
 .UNSPECIFIED., .F., .T. ) 
 B_SPLINE_CURVE_WITH_KNOTS ( ( 3, 2, 2, 2, 3 ),
 ( 0.3653846153846154188, 0.3717948717948718063, 0.3846153846153846367, 0.3974358974358974117, 0.4038461538461538547 ),
 .UNSPECIFIED. ) 
 CURVE ( )  GEOMETRIC_REPRESENTATION_ITEM ( )  RATIONAL_B_SPLINE_CURVE ( ( 0.9330127018922194093, 0.9330127018922196314, 1.000000000000000000, 0.8660254037844387076, 1.000000000000000000, 0.8660254037844387076, 1.000000000000000000, 0.9330127018922190762, 0.9330127018922194093 ) ) 
 REPRESENTATION_ITEM ( '' )  );
#4133=CARTESIAN_POINT ( 'NONE',  ( 28.40332666278570173, -4.614808937445885384, -7.939653947423662039 ) ) ;
#4137=DIRECTION ( 'NONE',  ( 0.000000000000000000, 0.000000000000000000, -1.000000000000000000 ) ) ;
#4139=CARTESIAN_POINT ( 'NONE',  ( 29.81991338116587542, -2.990324628369393611, -8.283357778048660691 ) ) ;
#4143=CARTESIAN_POINT ( 'NONE',  ( 26.10855331130634127, -2.710563430764044490, -4.533357778048659803 ) ) ;
#4154=ORIENTED_EDGE ( 'NONE', *, *, #1019, .T. ) ;
#4162=PLANE ( 'NONE',  #8729 ) ;
#4165=CARTESIAN_POINT ( 'NONE',  ( 17.59269349951685157, -13.05689734314391970, -15.91118832497637570 ) ) ;
#4168=CARTESIAN_POINT ( 'NONE',  ( 29.54591158530375239, -2.596238420101622868, -6.861505862736158257 ) ) ;
#4173=EDGE_CURVE ( 'NONE', #2932, #29, #1091, .T. ) ;
#4176=CARTESIAN_POINT ( 'NONE',  ( 30.02326902268086428, -5.673578940050561847, -3.627061608673667781 ) ) ;
#4177=CARTESIAN_POINT ( 'NONE',  ( 29.16815758536418102, -2.004582921727632971, -5.783357778048664244 ) ) ;
#4178=CARTESIAN_POINT ( 'NONE',  ( 25.92409770820621162, -4.135217962343409326, -3.765474553462066165 ) ) ;
#4184=CARTESIAN_POINT ( 'NONE',  ( 28.48022645605872327, -3.151730446115816875, -8.283357778048658915 ) ) ;
#4185=CARTESIAN_POINT ( 'NONE',  ( 31.53813789838894621, -6.745008222462202774, -5.783357778048668685 ) ) ;
#4188=LINE ( 'NONE', #13876, #15131 ) ;
#4192=EDGE_LOOP ( 'NONE', ( #14114, #14791, #14320, #11733 ) ) ;
#4200=CARTESIAN_POINT ( 'NONE',  ( 30.15443244188179150, -1.895953141405083864, -5.783357778048658915 ) ) ;
#4203=CARTESIAN_POINT ( 'NONE',  ( 31.49429780130001433, -5.496349022752856861, -7.939653947423664704 ) ) ;
#4214=ORIENTED_EDGE ( 'NONE', *, *, #10326, .F. ) ;
#4218=DIRECTION ( 'NONE',  ( -0.9928203230275514102, -0.1196152422706598939, 0.000000000000000000 ) ) ;
#4219=CARTESIAN_POINT ( 'NONE',  ( 25.99533317148741318, -3.650983533393564517, -3.627061608673662008 ) ) ;
#4226=DIRECTION ( 'NONE',  ( 0.9928203230275510771, 0.1196152422706614621, -0.000000000000000000 ) ) ;
#4246=ADVANCED_FACE ( 'NONE', ( #8913 ), #8827, .F. ) ;
#4247=CARTESIAN_POINT ( 'NONE',  ( 27.69360539047986336, -12.07076363665953345, -13.80168160306295810 ) ) ;
#4254=EDGE_LOOP ( 'NONE', ( #6588, #9011, #7077, #4935 ) ) ;
#4257=VERTEX_POINT ( 'NONE', #8549 ) ;
#4259=DIRECTION ( 'NONE',  ( -0.1196152422706597551, 0.9928203230275514102, 0.000000000000000000 ) ) ;
#4262=CARTESIAN_POINT ( 'NONE',  ( 25.07353123778398896, 1.235291682954687165, -14.60266621045498425 ) ) ;
#4266=FACE_OUTER_BOUND ( 'NONE', #14255, .T. ) ;
#4268=CARTESIAN_POINT ( 'NONE',  ( 27.81599742762458050, -2.504850134108091098, -7.033357778048658027 ) ) ;
#4270=CARTESIAN_POINT ( 'NONE',  ( 32.04158527077989760, -6.057382223572642665, -4.705209693361168455 ) ) ;
#4271=CYLINDRICAL_SURFACE ( 'NONE', #8152, 13.00000000000000178 ) ;
#4272=CARTESIAN_POINT ( 'NONE',  ( 26.58890374069123652, -3.379597482641427231, -8.283357778048660691 ) ) ;
#4280=CARTESIAN_POINT ( 'NONE',  ( -21.03265992632394799, -10.27181489424398997, -15.32141966295701430 ) ) ;
#4281=VERTEX_POINT ( 'NONE', #14359 ) ;
#4283=CARTESIAN_POINT ( 'NONE',  ( 31.44176105920648112, -5.502678662656354192, -3.627061608673668225 ) ) ;
#4285=EDGE_CURVE ( 'NONE', #7229, #11807, #13826, .T. ) ;
#4286=CARTESIAN_POINT ( 'NONE',  ( 32.12473870642251939, -5.420393343910986594, -7.939653947423664704 ) ) ;
#4290=CARTESIAN_POINT ( 'NONE',  ( 16.75000000000000000, -16.21813761408365195, -16.03574476417184513 ) ) ;
#4297=CARTESIAN_POINT ( 'NONE',  ( 23.00000000000000000, -16.21813761408365195, -13.00000000000000178 ) ) ;
#4299=CARTESIAN_POINT ( 'NONE',  ( 26.31284730449749532, -7.327874027665321144, -6.311983372246984914 ) ) ;
#4304=CARTESIAN_POINT ( 'NONE',  ( 28.52162355051263987, -6.481468097106410475, -6.861505862736167138 ) ) ;
#4307=FACE_OUTER_BOUND ( 'NONE', #9565, .T. ) ;
#4312=CARTESIAN_POINT ( 'NONE',  ( -13.65694651542706595, -25.37101204406941335, -16.45580752066269881 ) ) ;
#4315=ORIENTED_EDGE ( 'NONE', *, *, #4173, .T. ) ;
#4316=CIRCLE ( 'NONE', #7810, 6.249999999999998224 ) ;
#4318=ADVANCED_FACE ( 'NONE', ( #14531 ), #17170, .F. ) ;
#4326=CARTESIAN_POINT ( 'NONE',  ( 32.97211790677835097, -2.610546234160043610, -8.283357778048660691 ) ) ;
#4328=CARTESIAN_POINT ( 'NONE',  ( 32.52441275490655670, -6.636378442139655220, -5.783357778048663356 ) ) ;
#4331=DIRECTION ( 'NONE',  ( 1.000000000000000000, 0.000000000000000000, 0.000000000000000000 ) ) ;
#4334=ORIENTED_EDGE ( 'NONE', *, *, #2122, .T. ) ;
#4336=CARTESIAN_POINT ( 'NONE',  ( 30.25524682244395436, -4.391689130744175884, -3.283357778048664688 ) ) ;
#4340=ADVANCED_FACE ( 'NONE', ( #3368, #11970 ), #3550, .T. ) ;
#4343=FACE_OUTER_BOUND ( 'NONE', #9828, .T. ) ;
#4345=CARTESIAN_POINT ( 'NONE',  ( 25.95642634701329499, -4.403549397486640871, -3.686412874245495797 ) ) ;
#4348=DIRECTION ( 'NONE',  ( -0.7681011886108269904, 0.5760758914581205481, 0.2795659695588259552 ) ) ;
#4353=CARTESIAN_POINT ( 'NONE',  ( 28.64916707261694384, -6.765910400363817523, -4.533357778048668685 ) ) ;
#4355=CARTESIAN_POINT ( 'NONE',  ( 30.25080928106424594, -3.138282701210941994, -3.627061608673662896 ) ) ;
#4358=CARTESIAN_POINT ( 'NONE',  ( 5.499998817156068753, -20.49639288455253450, -13.00000000000000178 ) ) ;
#4359=VERTEX_POINT ( 'NONE', #7543 ) ;
#4365=EDGE_CURVE ( 'NONE', #17122, #3121, #9743, .T. ) ;
#4370=CYLINDRICAL_SURFACE ( 'NONE', #15365, 5.000000000000000000 ) ;
#4377=CARTESIAN_POINT ( 'NONE',  ( 32.14665875496697822, -6.044722943765660439, -6.861505862736166250 ) ) ;
#4382=ORIENTED_EDGE ( 'NONE', *, *, #6273, .F. ) ;
#4384=VECTOR ( 'NONE', #2229, 1000.000000000000000 ) ;
#4389=AXIS2_PLACEMENT_3D ( 'NONE', #13172, #4908, #931 ) ;
#4395=CARTESIAN_POINT ( 'NONE',  ( 25.88156304229571703, -4.918631652813365562, -7.939653947423662039 ) ) ;
#4397=CARTESIAN_POINT ( 'NONE',  ( 31.20090818012769773, -4.277755612481361602, -8.283357778048662468 ) ) ;
#4402=CARTESIAN_POINT ( 'NONE',  ( 27.87986455999572399, -6.131689368163070419, -3.283357778048667797 ) ) ;
#4411=DIRECTION ( 'NONE',  ( 0.9928203230275512992, 0.1196152422706614898, -0.000000000000000000 ) ) ;
#4412=DIRECTION ( 'NONE',  ( 0.000000000000000000, 1.000000000000000000, 3.469446951953614189E-16 ) ) ;
#4417=CARTESIAN_POINT ( 'NONE',  ( 33.26181313012506280, -6.547536259434060923, -6.453230759126471483 ) ) ;
#4419=AXIS2_PLACEMENT_3D ( 'NONE', #6309, #3410, #5033 ) ;
#4437=CARTESIAN_POINT ( 'NONE',  ( 26.47269060886452507, -6.728324053342490174, -6.861505862736166250 ) ) ;
#4438=PLANE ( 'NONE',  #15878 ) ;
#4439=CARTESIAN_POINT ( 'NONE',  ( -35.77680296528374271, -19.03270077640483038, -0.5379818257722512875 ) ) ;
#4440=DIRECTION ( 'NONE',  ( 0.6000000000000000888, 0.7999999999999999334, -0.000000000000000000 ) ) ;
#4443=DIRECTION ( 'NONE',  ( 0.000000000000000000, 0.000000000000000000, 1.000000000000000000 ) ) ;
#4444=CARTESIAN_POINT ( 'NONE',  ( -2.016448651773435938E-27, -20.49999999999999645, -13.00000000000000178 ) ) ;
#4447=ORIENTED_EDGE ( 'NONE', *, *, #3072, .F. ) ;
#4449=CARTESIAN_POINT ( 'NONE',  ( 29.50659824675005893, -4.481886499472614638, -7.939653947423662039 ) ) ;
#4457=CARTESIAN_POINT ( 'NONE',  ( 25.71748644841968456, -2.420320648352051851, -5.783357778048663356 ) ) ;
#4461=CARTESIAN_POINT ( 'NONE',  ( 26.39823381822652593, -6.110324093391315436, -3.627061608673668225 ) ) ;
#4463=CARTESIAN_POINT ( 'NONE',  ( 31.39792096211754924, -4.254019462947003838, -7.939653947423662039 ) ) ;
#4464=ADVANCED_FACE ( 'NONE', ( #3346 ), #3523, .F. ) ;
#4465=CARTESIAN_POINT ( 'NONE',  ( 27.82847066025702887, -2.165988739474055791, -5.783357778048658027 ) ) ;
#4470=DIRECTION ( 'NONE',  ( -0.000000000000000000, -0.000000000000000000, -1.000000000000000000 ) ) ;
#4471=ORIENTED_EDGE ( 'NONE', *, *, #12646, .F. ) ;
#4476=DIRECTION ( 'NONE',  ( 0.000000000000000000, 0.000000000000000000, -1.000000000000000000 ) ) ;
#4477=EDGE_LOOP ( 'NONE', ( #17425, #13350 ) ) ;
#4483=CARTESIAN_POINT ( 'NONE',  ( 26.82722439997946395, -4.804698134550569044, -3.627061608673664672 ) ) ;
#4485=CARTESIAN_POINT ( 'NONE',  ( 33.18226487515251222, -2.585227674546096033, -3.283357778048662023 ) ) ;
#4489=CARTESIAN_POINT ( 'NONE',  ( 28.91547068018125799, -2.672194098943493135, -6.861505862736158257 ) ) ;
#4494=ORIENTED_EDGE ( 'NONE', *, *, #9496, .F. ) ;
#4498=DIRECTION ( 'NONE',  ( -0.000000000000000000, -0.000000000000000000, -1.000000000000000000 ) ) ;
#4505=CARTESIAN_POINT ( 'NONE',  ( -45.50000000000000000, -16.03270077640482683, -5.537981825772250843 ) ) ;
#4517=VERTEX_POINT ( 'NONE', #17432 ) ;
#4520=CARTESIAN_POINT ( 'NONE',  ( 26.66961417369883591, -4.823687054261037055, -3.627061608673664672 ) ) ;
#4525=CARTESIAN_POINT ( 'NONE',  ( 2.749999999999992895, -20.49999999999999645, -13.00000000000000178 ) ) ;
#4527=DIRECTION ( 'NONE',  ( 0.000000000000000000, 0.000000000000000000, 1.000000000000000000 ) ) ;
#4528=CARTESIAN_POINT ( 'NONE',  ( 26.30185955129047315, -7.986322017489088765, -6.648778972250404706 ) ) ;
#4530=CARTESIAN_POINT ( 'NONE',  ( 31.39792096211754924, -4.254019462947003838, -7.939653947423662039 ) ) ;
#4532=CARTESIAN_POINT ( 'NONE',  ( 26.24651417059167358, -6.811311830135031720, -4.396611942026659392 ) ) ;
#4533=EDGE_LOOP ( 'NONE', ( #798, #2361, #8415, #13671 ) ) ;
#4538=CARTESIAN_POINT ( 'NONE',  ( 33.40301380667672504, -2.758504307001591993, -3.627061608673662896 ) ) ;
#4539=ORIENTED_EDGE ( 'NONE', *, *, #3039, .F. ) ;
#4541=CARTESIAN_POINT ( 'NONE',  ( -25.20502126318114833, -10.36657009486825842, -14.42817146764052083 ) ) ;
#4542=EDGE_LOOP ( 'NONE', ( #7276, #115, #15794, #10722 ) ) ;
#4545=CARTESIAN_POINT ( 'NONE',  ( 26.52522735095806894, -6.721994413439005278, -4.705209693361169343 ) ) ;
#4547=ORIENTED_EDGE ( 'NONE', *, *, #3938, .T. ) ;
#4548=CARTESIAN_POINT ( 'NONE',  ( 30.12381574833269937, -2.526612381163247267, -4.705209693361161349 ) ) ;
#4550=DIRECTION ( 'NONE',  ( 0.9928203230275510771, 0.1196152422706614621, -0.000000000000000000 ) ) ;
#4553=DIRECTION ( 'NONE',  ( -0.7999999999999999334, 0.6000000000000000888, 0.000000000000000000 ) ) ;
#4559=DIRECTION ( 'NONE',  ( 0.000000000000000000, 0.000000000000000000, -1.000000000000000000 ) ) ;
#4561=CARTESIAN_POINT ( 'NONE',  ( 26.18940839444933033, -6.337336286969802224, -7.823481096485427777 ) ) ;
#4564=CARTESIAN_POINT ( 'NONE',  ( -23.02601376483258022, 3.965314980223224151, 0.000000000000000000 ) ) ;
#4565=ORIENTED_EDGE ( 'NONE', *, *, #1194, .T. ) ;
#4567=CARTESIAN_POINT ( 'NONE',  ( 26.64639396487419987, -2.308405637095112706, -5.783357778048658027 ) ) ;
#4568=CARTESIAN_POINT ( 'NONE',  ( 27.65458886993626564, -2.824105456627233224, -6.861505862736158257 ) ) ;
#4569=CARTESIAN_POINT ( 'NONE',  ( 32.77701044293393551, -4.087866415376695706, -3.283357778048664688 ) ) ;
#4573=FACE_OUTER_BOUND ( 'NONE', #3714, .T. ) ;
#4574=CARTESIAN_POINT ( 'NONE',  ( 28.40332666278570173, -4.614808937445885384, -7.939653947423662039 ) ) ;
#4577=CARTESIAN_POINT ( 'NONE',  ( -9.099998387031003944, -19.29508120620799616, -16.81964500401478091 ) ) ;
#4591=CARTESIAN_POINT ( 'NONE',  ( 13.00000000000000178, 0.000000000000000000, -10.50000000000000000 ) ) ;
#4603=ORIENTED_EDGE ( 'NONE', *, *, #9645, .F. ) ;
#4604=ORIENTED_EDGE ( 'NONE', *, *, #8554, .F. ) ;
#4606=VECTOR ( 'NONE', #4664, 1000.000000000000000 ) ;
#4613=DIRECTION ( 'NONE',  ( 1.000000000000000000, 0.000000000000000000, 0.000000000000000000 ) ) ;
#4619=VERTEX_POINT ( 'NONE', #11073 ) ;
#4620=CARTESIAN_POINT ( 'NONE',  ( 28.38593337277646711, -7.124786616671554107, -5.783357778048668685 ) ) ;
#4622=CARTESIAN_POINT ( 'NONE',  ( 26.86291784143654127, -6.981118157082444320, -7.033357778048666908 ) ) ;
#4635=AXIS2_PLACEMENT_3D ( 'NONE', #140, #8761, #14291 ) ;
#4636=CARTESIAN_POINT ( 'NONE',  ( 27.12922144900085186, -2.887401855662130146, -4.705209693361160461 ) ) ;
#4640=CARTESIAN_POINT ( 'NONE',  ( 26.34117031759772942, -2.982346454214467535, -4.705209693361161349 ) ) ;
#4643=CARTESIAN_POINT ( 'NONE',  ( 33.76397967447234549, -5.422769698972272678, -8.283357778048664244 ) ) ;
#4647=LINE ( 'NONE', #13084, #7743 ) ;
#4660=CARTESIAN_POINT ( 'NONE',  ( 26.73899421642883567, -2.634607751922174224, -4.533357778048659803 ) ) ;
#4661=CARTESIAN_POINT ( 'NONE',  ( 33.27992013083530054, -6.934902899450660740, -5.783357778048669573 ) ) ;
#4664=DIRECTION ( 'NONE',  ( -0.000000000000000000, -0.000000000000000000, -1.000000000000000000 ) ) ;
#4678=AXIS2_PLACEMENT_3D ( 'NONE', #2662, #1218, #9362 ) ;
#4679=AXIS2_PLACEMENT_3D ( 'NONE', #99, #2549, #8172 ) ;
#4682=CARTESIAN_POINT ( 'NONE',  ( 32.55256711014040150, -6.632986398338614364, -6.453230759126470595 ) ) ;
#4683=( BOUNDED_CURVE ( )  B_SPLINE_CURVE ( 3, ( #15233, #5522, #17733, #11124 ),
 .UNSPECIFIED., .F., .T. ) 
 B_SPLINE_CURVE_WITH_KNOTS ( ( 4, 4 ),
 ( 1.825438360997748255, 1.919862177193756514 ),
 .UNSPECIFIED. ) 
 CURVE ( )  GEOMETRIC_REPRESENTATION_ITEM ( )  RATIONAL_B_SPLINE_CURVE ( ( 1.000000000000000000, 0.9992571499088201969, 0.9992571499088201969, 1.000000000000000000 ) ) 
 REPRESENTATION_ITEM ( '' )  );
#4693=VERTEX_POINT ( 'NONE', #6100 ) ;
#4695=EDGE_LOOP ( 'NONE', ( #4214, #9797, #8476, #3359 ) ) ;
#4699=CARTESIAN_POINT ( 'NONE',  ( -15.38839387855823126, 12.77214111725050216, -16.22946975555079163 ) ) ;
#4707=CARTESIAN_POINT ( 'NONE',  ( 36.07773319708005744, -23.32620662758124297, -11.14818368178938357 ) ) ;
#4708=( BOUNDED_CURVE ( )  B_SPLINE_CURVE ( 2, ( #5386, #13398, #10902, #4139, #16470, #14763, #2348, #7867, #980 ),
 .UNSPECIFIED., .F., .T. ) 
 B_SPLINE_CURVE_WITH_KNOTS ( ( 3, 2, 2, 2, 3 ),
 ( 0.4038461538461538547, 0.4102564102564102422, 0.4230769230769230727, 0.4358974358974359031, 0.4423076923076923461 ),
 .UNSPECIFIED. ) 
 CURVE ( )  GEOMETRIC_REPRESENTATION_ITEM ( )  RATIONAL_B_SPLINE_CURVE ( ( 0.9330127018922194093, 0.9330127018922196314, 1.000000000000000000, 0.8660254037844387076, 1.000000000000000000, 0.8660254037844387076, 1.000000000000000000, 0.9330127018922190762, 0.9330127018922194093 ) ) 
 REPRESENTATION_ITEM ( '' )  );
#4711=CARTESIAN_POINT ( 'NONE',  ( 26.84461768998868436, -2.294720455324902542, -5.783357778048658027 ) ) ;
#4712=CARTESIAN_POINT ( 'NONE',  ( 25.74999999999999645, -16.21813761408365195, 0.000000000000000000 ) ) ;
#4715=CIRCLE ( 'NONE', #7046, 2.749999999999988454 ) ;
#4718=ORIENTED_EDGE ( 'NONE', *, *, #17640, .T. ) ;
#4721=CARTESIAN_POINT ( 'NONE',  ( 32.77709966008947617, -5.968767264923789284, -6.861505862736166250 ) ) ;
#4725=CARTESIAN_POINT ( 'NONE',  ( 26.18940839444933033, -6.337336286969802224, -7.823481096485427777 ) ) ;
#4727=CARTESIAN_POINT ( 'NONE',  ( 28.41655006632555569, -6.494127376913395366, -4.705209693361169343 ) ) ;
#4729=CARTESIAN_POINT ( 'NONE',  ( 28.35948656569675919, -3.366149737736551906, -3.627061608673662896 ) ) ;
#4730=CARTESIAN_POINT ( 'NONE',  ( 27.81599742762458050, -2.504850134108091098, -7.033357778048658027 ) ) ;
#4737=EDGE_CURVE ( 'NONE', #7494, #9058, #13179, .T. ) ;
#4742=FACE_OUTER_BOUND ( 'NONE', #14919, .T. ) ;
#4744=CARTESIAN_POINT ( 'NONE',  ( 33.66004903264008874, -1.463398710186760487, -5.783357778048663356 ) ) ;
#4748=CARTESIAN_POINT ( 'NONE',  ( 29.49727470010032704, -7.390636972501882340, -5.783357778048669573 ) ) ;
#4755=LINE ( 'NONE', #1789, #13843 ) ;
#4763=ORIENTED_EDGE ( 'NONE', *, *, #10602, .T. ) ;
#4769=CARTESIAN_POINT ( 'NONE',  ( 33.33308377457396432, -5.274811626130743392, -3.627061608673668225 ) ) ;
#4770=ORIENTED_EDGE ( 'NONE', *, *, #12443, .T. ) ;
#4784=CARTESIAN_POINT ( 'NONE',  ( -8.968477750016525363, -19.11972035685536042, -16.82776078363834671 ) ) ;
#4785=( BOUNDED_CURVE ( )  B_SPLINE_CURVE ( 2, ( #637, #7706, #10412 ),
 .UNSPECIFIED., .F., .T. ) 
 B_SPLINE_CURVE_WITH_KNOTS ( ( 3, 3 ),
 ( 0.000000000000000000, 1.000000000000000000 ),
 .UNSPECIFIED. ) 
 CURVE ( )  GEOMETRIC_REPRESENTATION_ITEM ( )  RATIONAL_B_SPLINE_CURVE ( ( 0.9436786787937823107, 0.9410169847269389543, 0.9390195162974519505 ) ) 
 REPRESENTATION_ITEM ( '' )  );
#4786=DIRECTION ( 'NONE',  ( -1.000000000000000000, 0.000000000000000000, 0.000000000000000000 ) ) ;
#4789=CARTESIAN_POINT ( 'NONE',  ( -16.91320375285265953, -17.65223671300078223, -16.01217750721622579 ) ) ;
#4791=FACE_OUTER_BOUND ( 'NONE', #12767, .T. ) ;
#4794=CARTESIAN_POINT ( 'NONE',  ( 25.89088658894545603, -2.009881179784104965, -5.783357778048658027 ) ) ;
#4796=CARTESIAN_POINT ( 'NONE',  ( 33.30663696749426350, -1.516174747195733863, -5.783357778048658027 ) ) ;
#4797=FACE_BOUND ( 'NONE', #8132, .T. ) ;
#4798=VERTEX_POINT ( 'NONE', #2136 ) ;
#4803=CARTESIAN_POINT ( 'NONE',  ( 32.75517961154501023, -5.344437665069116328, -7.939653947423662927 ) ) ;
#4805=( BOUNDED_CURVE ( )  B_SPLINE_CURVE ( 3, ( #94, #11118, #4262, #9761 ),
 .UNSPECIFIED., .F., .T. ) 
 B_SPLINE_CURVE_WITH_KNOTS ( ( 4, 4 ),
 ( 1.230954889131919305, 1.393542617697868691 ),
 .UNSPECIFIED. ) 
 CURVE ( )  GEOMETRIC_REPRESENTATION_ITEM ( )  RATIONAL_B_SPLINE_CURVE ( ( 1.000000000000000000, 0.9977983154653933262, 0.9977983154653933262, 1.000000000000000000 ) ) 
 REPRESENTATION_ITEM ( '' )  );
#4812=CARTESIAN_POINT ( 'NONE',  ( 26.66961417369883591, -4.823687054261037055, -3.627061608673664672 ) ) ;
#4824=ORIENTED_EDGE ( 'NONE', *, *, #194, .T. ) ;
#4828=EDGE_CURVE ( 'NONE', #1377, #16314, #10443, .T. ) ;
#4830=CARTESIAN_POINT ( 'NONE',  ( 32.17274868998081416, -2.279756424927169345, -4.705209693361160461 ) ) ;
#4833=CARTESIAN_POINT ( 'NONE',  ( 30.69058026372202974, -5.793053633118939061, -8.283357778048662468 ) ) ;
#4866=EDGE_CURVE ( 'NONE', #7917, #4619, #1992, .T. ) ;
#4870=ORIENTED_EDGE ( 'NONE', *, *, #10691, .F. ) ;
#4872=AXIS2_PLACEMENT_3D ( 'NONE', #17302, #2059, #14475 ) ;
#4875=CARTESIAN_POINT ( 'NONE',  ( 33.48062616923409252, 0.02583177435456097265, -5.783357778048662468 ) ) ;
#4877=CARTESIAN_POINT ( 'NONE',  ( -26.11936545685874833, -21.64910423302892895, -14.20663795870742696 ) ) ;
#4879=CARTESIAN_POINT ( 'NONE',  ( 31.08079519141086067, -2.838413270685653078, -8.283357778048660691 ) ) ;
#4884=ORIENTED_EDGE ( 'NONE', *, *, #1194, .F. ) ;
#4886=CARTESIAN_POINT ( 'NONE',  ( 26.21417678486618641, -2.370676134166772808, -5.783357778048658027 ) ) ;
#4888=ORIENTED_EDGE ( 'NONE', *, *, #14108, .T. ) ;
#4890=ADVANCED_FACE ( 'NONE', ( #1030 ), #5599, .F. ) ;
#4891=CARTESIAN_POINT ( 'NONE',  ( -35.41536221060850664, -16.03270077640482683, -0.5379818257722508434 ) ) ;
#4894=( BOUNDED_CURVE ( )  B_SPLINE_CURVE ( 2, ( #7813, #4993, #7904, #828, #10427, #923, #4902, #17271, #7549 ),
 .UNSPECIFIED., .F., .T. ) 
 B_SPLINE_CURVE_WITH_KNOTS ( ( 3, 2, 2, 2, 3 ),
 ( 0.3269230769230769273, 0.3333333333333333148, 0.3461538461538461453, 0.3589743589743589758, 0.3653846153846154188 ),
 .UNSPECIFIED. ) 
 CURVE ( )  GEOMETRIC_REPRESENTATION_ITEM ( )  RATIONAL_B_SPLINE_CURVE ( ( 0.9330127018922194093, 0.9330127018922194093, 1.000000000000000000, 0.8660254037844387076, 1.000000000000000000, 0.8660254037844387076, 1.000000000000000000, 0.9330127018922190762, 0.9330127018922194093 ) ) 
 REPRESENTATION_ITEM ( '' )  );
#4897=CARTESIAN_POINT ( 'NONE',  ( 33.27602027394517847, -2.146833986953896822, -4.705209693361161349 ) ) ;
#4899=CIRCLE ( 'NONE', #9521, 13.00000000000000178 ) ;
#4902=CARTESIAN_POINT ( 'NONE',  ( 31.27600417729400917, -6.449428405189353342, -7.033357778048666908 ) ) ;
#4905=CARTESIAN_POINT ( 'NONE',  ( 31.12210306526553083, -4.287250072544045665, -8.283357778048662468 ) ) ;
#4907=CARTESIAN_POINT ( 'NONE',  ( 27.61527553138257574, -4.709753535998224550, -7.939653947423662039 ) ) ;
#4908=DIRECTION ( 'NONE',  ( 0.000000000000000000, 0.000000000000000000, 1.000000000000000000 ) ) ;
#4909=CARTESIAN_POINT ( 'NONE',  ( 33.47428445112562656, -1.485779673698264913, -6.453230759126466154 ) ) ;
#4910=CARTESIAN_POINT ( 'NONE',  ( 14.05146698326616672, 13.69412420653798357, -16.38624388364804219 ) ) ;
#4917=CARTESIAN_POINT ( 'NONE',  ( -20.00000000000000355, 7.999999999999996447, -6.000000000000000000 ) ) ;
#4923=CARTESIAN_POINT ( 'NONE',  ( 31.87075164095941915, -4.197052703815608687, -3.627061608673664672 ) ) ;
#4925=CARTESIAN_POINT ( 'NONE',  ( 27.99987602667382802, -2.482696394238434578, -4.533357778048659803 ) ) ;
#4927=DIRECTION ( 'NONE',  ( 0.000000000000000000, 0.000000000000000000, 1.000000000000000000 ) ) ;
#4935=ORIENTED_EDGE ( 'NONE', *, *, #16072, .F. ) ;
#4937=ORIENTED_EDGE ( 'NONE', *, *, #8634, .F. ) ;
#4939=( LENGTH_UNIT ( ) NAMED_UNIT ( * ) SI_UNIT ( .MILLI., .METRE. ) );
#4940=FACE_OUTER_BOUND ( 'NONE', #11295, .T. ) ;
#4941=EDGE_CURVE ( 'NONE', #5360, #16822, #9268, .T. ) ;
#4943=VECTOR ( 'NONE', #11781, 1000.000000000000227 ) ;
#4948=AXIS2_PLACEMENT_3D ( 'NONE', #14139, #5881, #11404 ) ;
#4951=DIRECTION ( 'NONE',  ( -1.000000000000000000, 0.000000000000000000, 0.000000000000000000 ) ) ;
#4953=CARTESIAN_POINT ( 'NONE',  ( 33.12669930479518854, -6.563814807098823145, -5.113484796970860558 ) ) ;
#4968=DIRECTION ( 'NONE',  ( 0.000000000000000000, 0.000000000000000000, 1.000000000000000000 ) ) ;
#4969=CARTESIAN_POINT ( 'NONE',  ( -25.20430036322041545, -22.07000804769847591, -14.42834449896450799 ) ) ;
#4981=CARTESIAN_POINT ( 'NONE',  ( 28.13194630731337753, -5.901445976576171759, -3.627061608673667781 ) ) ;
#4986=ORIENTED_EDGE ( 'NONE', *, *, #6195, .F. ) ;
#4988=CARTESIAN_POINT ( 'NONE',  ( 33.40754056521197413, -5.892811586081919906, -6.861505862736166250 ) ) ;
#4989=ORIENTED_EDGE ( 'NONE', *, *, #17909, .F. ) ;
#4993=CARTESIAN_POINT ( 'NONE',  ( 30.95252083063564896, -1.789602389065743981, -6.453230759126464378 ) ) ;
#4994=ORIENTED_EDGE ( 'NONE', *, *, #11950, .F. ) ;
#4997=CARTESIAN_POINT ( 'NONE',  ( 31.17093069310692499, -6.462087684996337345, -4.533357778048668685 ) ) ;
#4998=CARTESIAN_POINT ( 'NONE',  ( 28.88938074516742205, -6.437160617781993999, -4.705209693361168455 ) ) ;
#5005=VERTEX_POINT ( 'NONE', #4177 ) ;
#5007=COLOUR_RGB ( '', 0.40784314, 0.44705882, 0.49803922) ;
#5015=CARTESIAN_POINT ( 'NONE',  ( 33.33308377457396432, -5.274811626130743392, -3.627061608673668225 ) ) ;
#5016=EDGE_CURVE ( 'NONE', #1330, #16314, #13361, .T. ) ;
#5017=ORIENTED_EDGE ( 'NONE', *, *, #2636, .T. ) ;
#5018=CARTESIAN_POINT ( 'NONE',  ( 25.95642634701329499, -4.403549397486640871, -3.686412874245495797 ) ) ;
#5019=CARTESIAN_POINT ( 'NONE',  ( 29.84999239022537409, -5.894327871574777333, -3.283357778048667797 ) ) ;
#5025=CARTESIAN_POINT ( 'NONE',  ( 34.91377932259078420, -11.86950488720510322, -11.57182824616228878 ) ) ;
#5030=ORIENTED_EDGE ( 'NONE', *, *, #15138, .T. ) ;
#5033=DIRECTION ( 'NONE',  ( -0.1196152422706611984, 0.9928203230275510771, 0.000000000000000000 ) ) ;
#5037=EDGE_CURVE ( 'NONE', #7494, #6265, #9676, .T. ) ;
#5039=LINE ( 'NONE', #7684, #14869 ) ;
#5049=ORIENTED_EDGE ( 'NONE', *, *, #2082, .T. ) ;
#5063=CARTESIAN_POINT ( 'NONE',  ( 26.65222088368961195, -7.333664733486695120, -5.783357778048669573 ) ) ;
#5065=ORIENTED_EDGE ( 'NONE', *, *, #3938, .F. ) ;
#5066=CARTESIAN_POINT ( 'NONE',  ( 31.56875459193803124, -6.114348982704044921, -4.705209693361169343 ) ) ;
#5070=DIRECTION ( 'NONE',  ( 1.000000000000000000, 0.000000000000000000, 0.000000000000000000 ) ) ;
#5074=CARTESIAN_POINT ( 'NONE',  ( 32.01513846370018967, -2.298745344637636912, -4.705209693361161349 ) ) ;
#5077=CARTESIAN_POINT ( 'NONE',  ( 25.94629020164262556, -4.319418220471658465, -8.066408332899133171 ) ) ;
#5079=ADVANCED_FACE ( 'NONE', ( #1547 ), #14050, .T. ) ;
#5080=LINE ( 'NONE', #14714, #14554 ) ;
#5081=CARTESIAN_POINT ( 'NONE',  ( 32.43181250335191379, -6.310176327312596811, -4.533357778048668685 ) ) ;
#5084=EDGE_CURVE ( 'NONE', #4359, #7377, #12679, .T. ) ;
#5085=CARTESIAN_POINT ( 'NONE',  ( 25.90934487712387480, 0.1208734971681841297, -15.78335777804866424 ) ) ;
#5093=CARTESIAN_POINT ( 'NONE',  ( 33.40745134805642635, -4.011910736534825439, -3.283357778048664688 ) ) ;
#5094=ORIENTED_EDGE ( 'NONE', *, *, #14365, .F. ) ;
#5095=CARTESIAN_POINT ( 'NONE',  ( 0.000000000000000000, 0.000000000000000000, 0.000000000000000000 ) ) ;
#5097=LINE ( 'NONE', #8004, #15403 ) ;
#5100=CARTESIAN_POINT ( 'NONE',  ( 29.18947247604337392, -3.066280307211263878, -8.283357778048658915 ) ) ;
#5107=CARTESIAN_POINT ( 'NONE',  ( 26.79666222766753592, -21.19920099154242976, -14.03599807436713398 ) ) ;
#5109=ADVANCED_FACE ( 'NONE', ( #3163 ), #8602, .F. ) ;
#5110=VERTEX_POINT ( 'NONE', #11580 ) ;
#5117=ADVANCED_FACE ( 'NONE', ( #1822 ), #4438, .F. ) ;
#5119=DIRECTION ( 'NONE',  ( -0.9928203230275514102, -0.1196152422706598939, 0.000000000000000000 ) ) ;
#5120=AXIS2_PLACEMENT_3D ( 'NONE', #5718, #11235, #2755 ) ;
#5131=EDGE_CURVE ( 'NONE', #17048, #15612, #13262, .T. ) ;
#5132=ORIENTED_EDGE ( 'NONE', *, *, #12047, .F. ) ;
#5137=EDGE_LOOP ( 'NONE', ( #3371, #16922 ) ) ;
#5143=FACE_OUTER_BOUND ( 'NONE', #16053, .T. ) ;
#5146=CARTESIAN_POINT ( 'NONE',  ( 27.45766530510195835, -4.728742455708699666, -3.627061608673664672 ) ) ;
#5149=CARTESIAN_POINT ( 'NONE',  ( 30.92509028327567933, -4.310986222078405206, -7.939653947423662039 ) ) ;
#5153=CARTESIAN_POINT ( 'NONE',  ( 33.95908713831676096, -3.945449517755638791, -3.283357778048664688 ) ) ;
#5154=AXIS2_PLACEMENT_3D ( 'NONE', #7355, #6053, #15681 ) ;
#5159=CARTESIAN_POINT ( 'NONE',  ( 28.88938074516742205, -6.437160617781993999, -4.705209693361168455 ) ) ;
#5166=CARTESIAN_POINT ( 'NONE',  ( 31.63243098167119172, -2.771952051906466874, -8.283357778048658915 ) ) ;
#5170=DIRECTION ( 'NONE',  ( 0.000000000000000000, -1.000000000000000000, -0.000000000000000000 ) ) ;
#5172=VERTEX_POINT ( 'NONE', #14135 ) ;
#5173=VECTOR ( 'NONE', #12021, 1000.000000000000000 ) ;
#5176=AXIS2_PLACEMENT_3D ( 'NONE', #13609, #14460, #6194 ) ;
#5179=CARTESIAN_POINT ( 'NONE',  ( -27.68235608956435811, -12.07326681422359194, -13.80428259828453896 ) ) ;
#5183=EDGE_CURVE ( 'NONE', #4257, #2866, #12363, .T. ) ;
#5188=CARTESIAN_POINT ( 'NONE',  ( 25.40682704530840397, -3.522014380262483702, -8.283357778048658915 ) ) ;
#5201=EDGE_LOOP ( 'NONE', ( #14346, #2164, #3184, #8400 ) ) ;
#5203=CARTESIAN_POINT ( 'NONE',  ( 33.23365877489121090, -6.550928303235100891, -5.783357778048663356 ) ) ;
#5204=ORIENTED_EDGE ( 'NONE', *, *, #11515, .T. ) ;
#5206=( GEOMETRIC_REPRESENTATION_CONTEXT ( 3 ) GLOBAL_UNCERTAINTY_ASSIGNED_CONTEXT ( ( #3004 ) ) GLOBAL_UNIT_ASSIGNED_CONTEXT ( ( #4939, #2245, #3502 ) ) REPRESENTATION_CONTEXT ( 'NONE', 'WORKASPACE' ) );
#5207=CARTESIAN_POINT ( 'NONE',  ( 31.24031073583692475, -4.273008382657478954, -3.627061608673664672 ) ) ;
#5209=EDGE_CURVE ( 'NONE', #6049, #11429, #13958, .T. ) ;
#5210=CARTESIAN_POINT ( 'NONE',  ( 30.71189515440122975, -6.854751018602581958, -5.783357778048663356 ) ) ;
#5211=CARTESIAN_POINT ( 'NONE',  ( -19.43845002722867221, 2.988003976273734263, 0.000000000000000000 ) ) ;
#5214=AXIS2_PLACEMENT_3D ( 'NONE', #16429, #8170, #13701 ) ;
#5220=CIRCLE ( 'NONE', #1181, 13.00000000000000178 ) ;
#5228=CARTESIAN_POINT ( 'NONE',  ( 30.05329989404488700, -6.934098741245490416, -5.113484796970860558 ) ) ;
#5233=ADVANCED_FACE ( 'NONE', ( #177 ), #17055, .F. ) ;
#5234=CARTESIAN_POINT ( 'NONE',  ( 27.15566825608056689, -6.646038734597135011, -4.705209693361169343 ) ) ;
#5236=DIRECTION ( 'NONE',  ( 0.9928203230275512992, 0.1196152422706587698, 0.000000000000000000 ) ) ;
#5237=ADVANCED_FACE ( 'NONE', ( #8796, #4343 ), #3626, .F. ) ;
#5238=VECTOR ( 'NONE', #17183, 1000.000000000000000 ) ;
#5239=CARTESIAN_POINT ( 'NONE',  ( 30.29464937815318493, -4.386941900920275472, -7.939653947423662039 ) ) ;
#5241=CARTESIAN_POINT ( 'NONE',  ( 26.01652455409633902, -4.902371455920928156, -5.783357778048663356 ) ) ;
#5242=VECTOR ( 'NONE', #1265, 1000.000000000000000 ) ;
#5248=CARTESIAN_POINT ( 'NONE',  ( 27.62849893492243325, -6.589071975465733644, -4.705209693361168455 ) ) ;
#5251=CARTESIAN_POINT ( 'NONE',  ( 26.31556265977298992, -7.384422263489805793, -5.783357778048663356 ) ) ;
#5253=DIRECTION ( 'NONE',  ( 1.000000000000000000, 0.000000000000000000, 0.000000000000000000 ) ) ;
#5254=CARTESIAN_POINT ( 'NONE',  ( 30.37154917142620292, -2.923863409590206519, -8.283357778048658915 ) ) ;
#5256=EDGE_CURVE ( 'NONE', #1670, #761, #1101, .T. ) ;
#5257=VERTEX_POINT ( 'NONE', #13044 ) ;
#5258=CARTESIAN_POINT ( 'NONE',  ( 33.19286683830256379, -2.783822866615540903, -7.939653947423660263 ) ) ;
#5268=VERTEX_POINT ( 'NONE', #9228 ) ;
#5270=ORIENTED_EDGE ( 'NONE', *, *, #13658, .F. ) ;
#5271=CARTESIAN_POINT ( 'NONE',  ( -29.03633718710667466, -14.58471626061076520, -13.43311195353574305 ) ) ;
#5273=SURFACE_SIDE_STYLE ('',( #12169 ) ) ;
#5275=CARTESIAN_POINT ( 'NONE',  ( 30.91186687973582536, -2.431667782610909434, -4.705209693361160461 ) ) ;
#5279=CARTESIAN_POINT ( 'NONE',  ( 26.78782184427022983, -4.809445364374452581, -8.283357778048662468 ) ) ;
#5286=EDGE_CURVE ( 'NONE', #16203, #2633, #15924, .T. ) ;
#5294=CARTESIAN_POINT ( 'NONE',  ( 30.18087924896149588, -5.654590020340094725, -3.627061608673668225 ) ) ;
#5295=EDGE_LOOP ( 'NONE', ( #13952, #9503, #5995, #6493, #2922 ) ) ;
#5298=CARTESIAN_POINT ( 'NONE',  ( 25.11802603177690330, -19.03270077640482683, -10.53798182577225084 ) ) ;
#5309=EDGE_LOOP ( 'NONE', ( #13206, #9388 ) ) ;
#5317=CARTESIAN_POINT ( 'NONE',  ( 27.27683486999669427, -2.232449958253242883, -5.783357778048658027 ) ) ;
#5318=FACE_BOUND ( 'NONE', #17618, .T. ) ;
#5320=CARTESIAN_POINT ( 'NONE',  ( 28.56587103547553852, -2.077146556768465047, -5.113484796970851676 ) ) ;
#5322=CARTESIAN_POINT ( 'NONE',  ( 29.20802265909081896, -15.38590642643731066, -13.38453386482100171 ) ) ;
#5324=CARTESIAN_POINT ( 'NONE',  ( 32.70264286945147347, -5.350767304972614546, -3.627061608673668225 ) ) ;
#5326=DIRECTION ( 'NONE',  ( 0.9928203230275510771, 0.1196152422706614621, -0.000000000000000000 ) ) ;
#5332=CARTESIAN_POINT ( 'NONE',  ( 28.86293393808771057, -2.678523738846987357, -4.705209693361161349 ) ) ;
#5337=DIRECTION ( 'NONE',  ( 0.000000000000000000, 1.000000000000000000, -0.000000000000000000 ) ) ;
#5340=CARTESIAN_POINT ( 'NONE',  ( 28.91555989733679866, -4.553094948490599592, -3.283357778048664688 ) ) ;
#5342=VERTEX_POINT ( 'NONE', #4875 ) ;
#5343=CARTESIAN_POINT ( 'NONE',  ( 32.16857880351144416, -6.669052543620333395, -5.783357778048668685 ) ) ;
#5345=CARTESIAN_POINT ( 'NONE',  ( 30.33776104811456165, -2.201027418740610919, -7.033357778048658027 ) ) ;
#5356=ORIENTED_EDGE ( 'NONE', *, *, #7800, .F. ) ;
#5357=CARTESIAN_POINT ( 'NONE',  ( 28.51709679197738723, -3.347160818026084339, -3.627061608673662008 ) ) ;
#5358=EDGE_LOOP ( 'NONE', ( #15703, #3326 ) ) ;
#5360=VERTEX_POINT ( 'NONE', #10747 ) ;
#5362=CARTESIAN_POINT ( 'NONE',  ( 32.77257290155422709, -2.834459985843461816, -3.627061608673662896 ) ) ;
#5372=DIRECTION ( 'NONE',  ( -0.000000000000000000, -0.000000000000000000, -1.000000000000000000 ) ) ;
#5374=LINE ( 'NONE', #10809, #16027 ) ;
#5381=CARTESIAN_POINT ( 'NONE',  ( 29.54591158530375239, -2.596238420101622868, -6.861505862736158257 ) ) ;
#5383=CARTESIAN_POINT ( 'NONE',  ( 30.69058026372202974, -5.793053633118939061, -8.283357778048664244 ) ) ;
#5386=CARTESIAN_POINT ( 'NONE',  ( 29.79859849048667897, -1.928627242885762705, -5.783357778048664244 ) ) ;
#5391=ORIENTED_EDGE ( 'NONE', *, *, #13189, .T. ) ;
#5403=FACE_OUTER_BOUND ( 'NONE', #17841, .T. ) ;
#5409=CARTESIAN_POINT ( 'NONE',  ( 29.25000000000000000, -16.21813761408365195, -13.37255996287876236 ) ) ;
#5414=CARTESIAN_POINT ( 'NONE',  ( 32.30426898124760982, -6.025734024055190652, -6.861505862736167138 ) ) ;
#5417=CARTESIAN_POINT ( 'NONE',  ( -23.00000000000000000, -16.21813761408365195, -13.00000000000000178 ) ) ;
#5418=CARTESIAN_POINT ( 'NONE',  ( 31.87265695910486230, -5.650636735497883478, -8.283357778048664244 ) ) ;
#5420=AXIS2_PLACEMENT_3D ( 'NONE', #14449, #17089, #1759 ) ;
#5422=VERTEX_POINT ( 'NONE', #16229 ) ;
#5424=CARTESIAN_POINT ( 'NONE',  ( 27.12505156253147831, -7.276697974355292864, -5.783357778048668685 ) ) ;
#5431=CARTESIAN_POINT ( 'NONE',  ( 27.84978555093622177, -3.227686124957687586, -8.283357778048658915 ) ) ;
#5439=CARTESIAN_POINT ( 'NONE',  ( 25.95642634701329499, -4.403549397486640871, -3.686412874245495797 ) ) ;
#5442=VECTOR ( 'NONE', #12694, 1000.000000000000000 ) ;
#5448=CARTESIAN_POINT ( 'NONE',  ( 30.28142597461332741, -2.507623461452779701, -4.705209693361160461 ) ) ;
#5450=ORIENTED_EDGE ( 'NONE', *, *, #11344, .F. ) ;
#5452=CARTESIAN_POINT ( 'NONE',  ( 32.54050588463559990, -2.235448945602741766, -6.861505862736159145 ) ) ;
#5458=CARTESIAN_POINT ( 'NONE',  ( 29.08935247050201767, -2.014077381790315702, -5.783357778048658027 ) ) ;
#5464=ORIENTED_EDGE ( 'NONE', *, *, #12835, .T. ) ;
#5470=CARTESIAN_POINT ( 'NONE',  ( 30.82871344409320713, -3.068656662272551738, -7.939653947423660263 ) ) ;
#5479=CARTESIAN_POINT ( 'NONE',  ( -21.42601376483257880, 2.765314980223223529, 0.000000000000000000 ) ) ;
#5484=VERTEX_POINT ( 'NONE', #12482 ) ;
#5486=CARTESIAN_POINT ( 'NONE',  ( 23.00000000000000000, -16.21813761408365195, -13.00000000000000178 ) ) ;
#5496=FACE_OUTER_BOUND ( 'NONE', #36, .T. ) ;
#5498=PLANE ( 'NONE',  #9074 ) ;
#5501=CARTESIAN_POINT ( 'NONE',  ( 28.08810621022444920, -4.652786776866828511, -3.627061608673664672 ) ) ;
#5502=AXIS2_PLACEMENT_3D ( 'NONE', #9526, #6908, #1115 ) ;
#5510=ORIENTED_EDGE ( 'NONE', *, *, #5707, .T. ) ;
#5513=CARTESIAN_POINT ( 'NONE',  ( 29.82181869931131146, -4.443908660051686610, -3.627061608673664672 ) ) ;
#5516=LINE ( 'NONE', #6886, #8149 ) ;
#5518=VECTOR ( 'NONE', #8991, 1000.000000000000000 ) ;
#5519=DIRECTION ( 'NONE',  ( 0.9928203230275511881, 0.1196152422706614760, 0.000000000000000000 ) ) ;
#5522=CARTESIAN_POINT ( 'NONE',  ( 30.07408527595748282, -27.82894256842317660, -13.18310524188698452 ) ) ;
#5523=CARTESIAN_POINT ( 'NONE',  ( 26.52132749406794687, -1.933925500942234921, -5.783357778048658027 ) ) ;
#5524=AXIS2_PLACEMENT_3D ( 'NONE', #13048, #10230, #1917 ) ;
#5525=CARTESIAN_POINT ( 'NONE',  ( 28.98992747081925359, -3.290194058894681639, -3.627061608673662896 ) ) ;
#5526=CARTESIAN_POINT ( 'NONE',  ( 28.16881664323204859, -6.096876348486420127, -8.283357778048664244 ) ) ;
#5527=FACE_OUTER_BOUND ( 'NONE', #14208, .T. ) ;
#5534=EDGE_CURVE ( 'NONE', #11901, #9058, #1618, .T. ) ;
#5535=CARTESIAN_POINT ( 'NONE',  ( -18.31874363337315970, -12.05639433133630511, -15.79760360980902689 ) ) ;
#5537=CARTESIAN_POINT ( 'NONE',  ( 29.67743187657054449, -6.342216019229654833, -4.705209693361169343 ) ) ;
#5540=CARTESIAN_POINT ( 'NONE',  ( 26.10855331130634127, -2.710563430764044490, -4.533357778048659803 ) ) ;
#5545=AXIS2_PLACEMENT_3D ( 'NONE', #9408, #9660, #2792 ) ;
#5546=CARTESIAN_POINT ( 'NONE',  ( 17.71310509092289465, -19.55788671310905613, -15.89250038334901305 ) ) ;
#5553=ORIENTED_EDGE ( 'NONE', *, *, #11040, .T. ) ;
#5558=ORIENTED_EDGE ( 'NONE', *, *, #10949, .F. ) ;
#5559=ORIENTED_EDGE ( 'NONE', *, *, #2253, .F. ) ;
#5560=CARTESIAN_POINT ( 'NONE',  ( 33.10345976029034887, -2.594722134608779207, -3.283357778048662023 ) ) ;
#5561=CARTESIAN_POINT ( 'NONE',  ( 29.76058531221316628, -5.705227139567997874, -7.939653947423664704 ) ) ;
#5562=ORIENTED_EDGE ( 'NONE', *, *, #12061, .F. ) ;
#5568=CARTESIAN_POINT ( 'NONE',  ( -23.00000000000000000, -16.21813761408365195, -13.00000000000000178 ) ) ;
#5572=ORIENTED_EDGE ( 'NONE', *, *, #11835, .F. ) ;
#5576=AXIS2_PLACEMENT_3D ( 'NONE', #3712, #14614, #5236 ) ;
#5582=DIRECTION ( 'NONE',  ( 0.9928203230275512992, 0.1196152422706614898, -0.000000000000000000 ) ) ;
#5583=CARTESIAN_POINT ( 'NONE',  ( 31.68992120585416217, -1.700760206360153015, -5.783357778048664244 ) ) ;
#5593=CARTESIAN_POINT ( 'NONE',  ( 30.03006034954003667, -2.965006068755446478, -3.283357778048662023 ) ) ;
#5598=CARTESIAN_POINT ( 'NONE',  ( 25.95642634701329499, -4.403549397486640871, -3.686412874245495352 ) ) ;
#5599=PLANE ( 'NONE',  #10349 ) ;
#5600=EDGE_CURVE ( 'NONE', #14870, #13858, #7057, .T. ) ;
#5604=CARTESIAN_POINT ( 'NONE',  ( 31.88017671309158274, -6.376637546091784792, -4.533357778048668685 ) ) ;
#5608=CARTESIAN_POINT ( 'NONE',  ( 29.23078034989804763, -4.515117109069654688, -8.283357778048662468 ) ) ;
#5611=CARTESIAN_POINT ( 'NONE',  ( 30.02326902268086428, -5.673578940050561847, -3.627061608673667781 ) ) ;
#5616=ORIENTED_EDGE ( 'NONE', *, *, #5183, .F. ) ;
#5621=FACE_OUTER_BOUND ( 'NONE', #8937, .T. ) ;
#5623=CARTESIAN_POINT ( 'NONE',  ( 28.28502977505876359, -2.748149777785362957, -6.861505862736158257 ) ) ;
#5626=VERTEX_POINT ( 'NONE', #8495 ) ;
#5627=ORIENTED_EDGE ( 'NONE', *, *, #11024, .T. ) ;
#5628=CARTESIAN_POINT ( 'NONE',  ( 30.64918316926811315, -2.463315982128351678, -6.861505862736159145 ) ) ;
#5634=EDGE_LOOP ( 'NONE', ( #4471, #213, #9562, #9242 ) ) ;
#5635=CARTESIAN_POINT ( 'NONE',  ( 30.00264913441657555, -6.940201157507134511, -5.783357778048657138 ) ) ;
#5639=SHAPE_REPRESENTATION ( 'Caliper Body Half', ( #3575 ), #2991 ) ;
#5648=ORIENTED_EDGE ( 'NONE', *, *, #8958, .F. ) ;
#5650=CARTESIAN_POINT ( 'NONE',  ( 26.39370705969127684, -2.976016814310973313, -6.861505862736158257 ) ) ;
#5653=PRODUCT_CONTEXT ( 'NONE', #14562, 'mechanical' ) ;
#5665=ADVANCED_FACE ( 'NONE', ( #9304 ), #17519, .F. ) ;
#5668=ORIENTED_EDGE ( 'NONE', *, *, #4173, .F. ) ;
#5671=CARTESIAN_POINT ( 'NONE',  ( 32.95080301609915097, -1.548848848676412260, -5.783357778048663356 ) ) ;
#5673=CARTESIAN_POINT ( 'NONE',  ( 26.18940839444933033, -6.337336286969802224, -7.823481096485427777 ) ) ;
#5675=CARTESIAN_POINT ( 'NONE',  ( 29.24999999999999645, -15.80522841342829921, -13.37255996287877480 ) ) ;
#5680=DIRECTION ( 'NONE',  ( -0.1196152422706621143, 0.9928203230275509661, 0.000000000000000000 ) ) ;
#5684=ORIENTED_EDGE ( 'NONE', *, *, #10282, .F. ) ;
#5686=CARTESIAN_POINT ( 'NONE',  ( 29.14074637024071990, -5.979778010479330774, -3.283357778048667797 ) ) ;
#5687=CARTESIAN_POINT ( 'NONE',  ( -25.11802603177690330, -19.03270077640483038, -0.5379818257722508434 ) ) ;
#5689=CARTESIAN_POINT ( 'NONE',  ( 25.78902048130849067, -3.014061381488925218, -4.757751673912568258 ) ) ;
#5692=CARTESIAN_POINT ( 'NONE',  ( 45.50000000000000000, -19.03270077640483038, -8.287981825772241962 ) ) ;
#5695=CARTESIAN_POINT ( 'NONE',  ( 27.78220930431293922, -1.782014143258494832, -5.783357778048658027 ) ) ;
#5697=CARTESIAN_POINT ( 'NONE',  ( 30.86385689617752348, -5.572304701594726239, -7.939653947423664704 ) ) ;
#5707=EDGE_CURVE ( 'NONE', #14370, #17637, #10127, .T. ) ;
#5708=ORIENTED_EDGE ( 'NONE', *, *, #15440, .T. ) ;
#5712=ORIENTED_EDGE ( 'NONE', *, *, #2168, .T. ) ;
#5713=CARTESIAN_POINT ( 'NONE',  ( -20.46503100693326260, -10.50166121531458430, -15.42720773483998009 ) ) ;
#5715=CARTESIAN_POINT ( 'NONE',  ( 35.77680296528374271, -19.03270077640483038, -0.5379818257722508434 ) ) ;
#5716=ORIENTED_EDGE ( 'NONE', *, *, #9764, .T. ) ;
#5717=CARTESIAN_POINT ( 'NONE',  ( 31.08270050955629671, -4.291997302367946077, -3.627061608673664672 ) ) ;
#5718=CARTESIAN_POINT ( 'NONE',  ( 0.000000000000000000, 0.000000000000000000, -8.700000000000001066 ) ) ;
#5728=APPLICATION_CONTEXT ( 'automotive_design' ) ;
#5732=DIRECTION ( 'NONE',  ( 1.000000000000000000, 0.000000000000000000, 0.000000000000000000 ) ) ;
#5735=ORIENTED_EDGE ( 'NONE', *, *, #13760, .T. ) ;
#5736=LINE ( 'NONE', #16825, #10690 ) ;
#5739=CARTESIAN_POINT ( 'NONE',  ( 27.67650891848073158, -3.448435056481901295, -7.939653947423660263 ) ) ;
#5740=VECTOR ( 'NONE', #5822, 1000.000000000000227 ) ;
#5741=CARTESIAN_POINT ( 'NONE',  ( 31.01321894478757812, -1.392741288986461212, -5.783357778048658027 ) ) ;
#5746=CARTESIAN_POINT ( 'NONE',  ( 28.08317206381523334, -7.171460237833785278, -5.113484796970862334 ) ) ;
#5749=AXIS2_PLACEMENT_3D ( 'NONE', #17582, #13468, #9450 ) ;
#5755=CARTESIAN_POINT ( 'NONE',  ( 26.03726795043090547, -3.446058701420613879, -8.283357778048660691 ) ) ;
#5762=CARTESIAN_POINT ( 'NONE',  ( 33.95908713831676096, -3.945449517755638791, -3.283357778048664688 ) ) ;
#5765=CARTESIAN_POINT ( 'NONE',  ( 32.50309786422735669, -5.574681056656013212, -8.283357778048664244 ) ) ;
#5767=CYLINDRICAL_SURFACE ( 'NONE', #3461, 5.500000000000000888 ) ;
#5774=PLANE ( 'NONE',  #11884 ) ;
#5776=VECTOR ( 'NONE', #12916, 1000.000000000000114 ) ;
#5777=ORIENTED_EDGE ( 'NONE', *, *, #4365, .F. ) ;
#5781=DIRECTION ( 'NONE',  ( 0.9396926207859104263, 0.000000000000000000, 0.3420201433256631618 ) ) ;
#5784=ADVANCED_FACE ( 'NONE', ( #52 ), #11082, .T. ) ;
#5790=EDGE_LOOP ( 'NONE', ( #12749, #12183, #14356, #11226 ) ) ;
#5792=VECTOR ( 'NONE', #2419, 1000.000000000000000 ) ;
#5795=CARTESIAN_POINT ( 'NONE',  ( 30.27725608814395031, -6.896919580145944195, -5.783357778048668685 ) ) ;
#5798=CARTESIAN_POINT ( 'NONE',  ( 26.31308423962587995, -7.363851090081254824, -5.799730202602000340 ) ) ;
#5801=ORIENTED_EDGE ( 'NONE', *, *, #3088, .F. ) ;
#5806=CARTESIAN_POINT ( 'NONE',  ( -18.90926271784950075, -11.47470670281267857, -15.70082023719634989 ) ) ;
#5809=CARTESIAN_POINT ( 'NONE',  ( 28.49970350196817392, -5.857138497251737519, -7.939653947423662927 ) ) ;
#5810=CARTESIAN_POINT ( 'NONE',  ( 30.67110321781257909, -3.087645581983020637, -7.939653947423660263 ) ) ;
#5822=DIRECTION ( 'NONE',  ( 0.9928203230275510771, 0.1196152422706614621, -0.000000000000000000 ) ) ;
#5825=CARTESIAN_POINT ( 'NONE',  ( 28.11132641904908169, -7.168068194032743534, -5.783357778048668685 ) ) ;
#5826=ORIENTED_EDGE ( 'NONE', *, *, #5828, .F. ) ;
#5827=DIRECTION ( 'NONE',  ( -0.000000000000000000, -1.000000000000000000, 0.000000000000000000 ) ) ;
#5828=EDGE_CURVE ( 'NONE', #8562, #2496, #13261, .T. ) ;
#5829=ORIENTED_EDGE ( 'NONE', *, *, #756, .T. ) ;
#5831=CARTESIAN_POINT ( 'NONE',  ( 26.52522735095806894, -6.721994413439005278, -4.705209693361169343 ) ) ;
#5833=CARTESIAN_POINT ( 'NONE',  ( 32.01903832059031174, -7.086814257134402162, -5.783357778048669573 ) ) ;
#5836=CARTESIAN_POINT ( 'NONE',  ( 30.80688261270428541, -4.325227911964988792, -3.283357778048664688 ) ) ;
#5839=CARTESIAN_POINT ( 'NONE',  ( 29.34898802046944155, -4.500875419183088866, -3.627061608673664672 ) ) ;
#5840=CARTESIAN_POINT ( 'NONE',  ( -2.016448651773435938E-27, -20.49999999999999645, -13.00000000000000178 ) ) ;
#5849=SURFACE_SIDE_STYLE ('',( #16747 ) ) ;
#5854=EDGE_CURVE ( 'NONE', #10333, #13069, #2503, .T. ) ;
#5855=ORIENTED_EDGE ( 'NONE', *, *, #2253, .T. ) ;
#5859=CYLINDRICAL_SURFACE ( 'NONE', #16025, 13.00000000000000178 ) ;
#5870=ORIENTED_EDGE ( 'NONE', *, *, #13770, .T. ) ;
#5874=DIRECTION ( 'NONE',  ( -0.9928203230275510771, -0.1196152422706610735, 0.000000000000000000 ) ) ;
#5875=DIRECTION ( 'NONE',  ( -0.000000000000000000, -0.000000000000000000, -1.000000000000000000 ) ) ;
#5880=ADVANCED_FACE ( 'NONE', ( #17778 ), #10817, .F. ) ;
#5881=DIRECTION ( 'NONE',  ( 0.9928203230275512992, 0.1196152422706614898, -0.000000000000000000 ) ) ;
#5882=CARTESIAN_POINT ( 'NONE',  ( 45.50000000000000000, -19.03270077640483038, -5.537981825772250843 ) ) ;
#5886=CARTESIAN_POINT ( 'NONE',  ( 29.82181869931131146, -4.443908660051686610, -3.627061608673664672 ) ) ;
#5888=CARTESIAN_POINT ( 'NONE',  ( 33.14105852333657509, -6.224726188408045147, -4.533357778048668685 ) ) ;
#5889=CARTESIAN_POINT ( 'NONE',  ( 36.27615609941022257, -23.17738945083361557, 0.000000000000000000 ) ) ;
#5890=ORIENTED_EDGE ( 'NONE', *, *, #12326, .F. ) ;
#5895=ORIENTED_EDGE ( 'NONE', *, *, #13074, .F. ) ;
#5898=LINE ( 'NONE', #15338, #1778 ) ;
#5902=CARTESIAN_POINT ( 'NONE',  ( 26.60838078660069428, -6.085005533777348319, -7.939653947423662927 ) ) ;
#5904=CARTESIAN_POINT ( 'NONE',  ( 32.02836186724004364, -4.178063784105134459, -7.939653947423662039 ) ) ;
#5906=CYLINDRICAL_SURFACE ( 'NONE', #17445, 2.749999999999992006 ) ;
#5907=CARTESIAN_POINT ( 'NONE',  ( 27.19802975513453092, -2.241944418315925613, -5.783357778048658027 ) ) ;
#5915=DIRECTION ( 'NONE',  ( 0.9928203230275510771, 0.1196152422706614621, -0.000000000000000000 ) ) ;
#5916=ADVANCED_FACE ( 'NONE', ( #4307 ), #3456, .F. ) ;
#5924=CARTESIAN_POINT ( 'NONE',  ( 33.95908713831676096, -3.945449517755638791, -3.283357778048664688 ) ) ;
#5929=CARTESIAN_POINT ( 'NONE',  ( 28.52162355051263987, -6.481468097106410475, -6.861505862736167138 ) ) ;
#5931=CARTESIAN_POINT ( 'NONE',  ( 26.01652455409633902, -4.902371455920928156, -5.783357778048663356 ) ) ;
#5935=ORIENTED_EDGE ( 'NONE', *, *, #1268, .F. ) ;
#5940=FACE_OUTER_BOUND ( 'NONE', #12125, .T. ) ;
#5943=CARTESIAN_POINT ( 'NONE',  ( 28.05993251931039012, -3.202367565343740452, -3.283357778048662023 ) ) ;
#5946=CARTESIAN_POINT ( 'NONE',  ( 27.45273115869273539, -7.247415916675651992, -5.113484796970856117 ) ) ;
#5959=CARTESIAN_POINT ( 'NONE',  ( 29.08935247050201767, -2.014077381790315702, -5.783357778048658027 ) ) ;
#5961=DIRECTION ( 'NONE',  ( -0.6000000000000000888, 0.7999999999999999334, 0.000000000000000000 ) ) ;
#5962=CARTESIAN_POINT ( 'NONE',  ( -23.83685604381143364, -22.42490655540755284, -14.74319968589249719 ) ) ;
#5968=( BOUNDED_CURVE ( )  B_SPLINE_CURVE ( 2, ( #3379, #4909, #3296, #572, #11797, #4643, #1943, #17184, #7554 ),
 .UNSPECIFIED., .F., .F. ) 
 B_SPLINE_CURVE_WITH_KNOTS ( ( 3, 2, 2, 2, 3 ),
 ( 0.01923076923076924918, 0.02564102564102564014, 0.03846153846153846367, 0.05128205128205128027, 0.05769230769230770939 ),
 .UNSPECIFIED. ) 
 CURVE ( )  GEOMETRIC_REPRESENTATION_ITEM ( )  RATIONAL_B_SPLINE_CURVE ( ( 0.9330127018922194093, 0.9330127018922195203, 1.000000000000000000, 0.8660254037844387076, 1.000000000000000000, 0.8660254037844387076, 1.000000000000000000, 0.9330127018922190762, 0.9330127018922194093 ) ) 
 REPRESENTATION_ITEM ( '' )  );
#5972=CARTESIAN_POINT ( 'NONE',  ( 27.09860475545177039, -3.518061095420291995, -3.627061608673662896 ) ) ;
#5974=LINE ( 'NONE', #8810, #17329 ) ;
#5982=ORIENTED_EDGE ( 'NONE', *, *, #6828, .F. ) ;
#5983=CARTESIAN_POINT ( 'NONE',  ( 29.42969845347704450, -5.944964990802679594, -8.283357778048664244 ) ) ;
#5984=EDGE_LOOP ( 'NONE', ( #13664, #5464 ) ) ;
#5986=CARTESIAN_POINT ( 'NONE',  ( 27.65911562847151117, -5.958412735707574015, -3.627061608673668225 ) ) ;
#5988=CARTESIAN_POINT ( 'NONE',  ( 27.26074174026764751, -6.633379454790151009, -6.861505862736167138 ) ) ;
#5990=CARTESIAN_POINT ( 'NONE',  ( 30.86385689617752348, -5.572304701594726239, -7.939653947423664704 ) ) ;
#5992=DIRECTION ( 'NONE',  ( -0.000000000000000000, -0.000000000000000000, -1.000000000000000000 ) ) ;
#5995=ORIENTED_EDGE ( 'NONE', *, *, #3739, .T. ) ;
#6003=ORIENTED_EDGE ( 'NONE', *, *, #2262, .T. ) ;
#6009=ORIENTED_EDGE ( 'NONE', *, *, #307, .F. ) ;
#6010=CARTESIAN_POINT ( 'NONE',  ( 23.02601376483258022, 3.965314980223224151, -6.000000000000000000 ) ) ;
#6013=CARTESIAN_POINT ( 'NONE',  ( 32.41296236253129592, -1.951006642345344044, -4.533357778048659803 ) ) ;
#6018=AXIS2_PLACEMENT_3D ( 'NONE', #9357, #9182, #92 ) ;
#6019=DIRECTION ( 'NONE',  ( 0.1195020427801297691, -0.9918807541847894926, 0.04349518650597276187 ) ) ;
#6020=AXIS2_PLACEMENT_3D ( 'NONE', #3495, #14195, #11546 ) ;
#6021=PLANE ( 'NONE',  #3722 ) ;
#6028=DIRECTION ( 'NONE',  ( -1.000000000000000000, 0.000000000000000000, 0.000000000000000000 ) ) ;
#6032=AXIS2_PLACEMENT_3D ( 'NONE', #9213, #977, #7600 ) ;
#6038=ADVANCED_FACE ( 'NONE', ( #9598 ), #1573, .F. ) ;
#6049=VERTEX_POINT ( 'NONE', #7796 ) ;
#6053=DIRECTION ( 'NONE',  ( -0.7999999999999999334, -0.6000000000000001998, 0.000000000000000000 ) ) ;
#6057=CARTESIAN_POINT ( 'NONE',  ( 31.32102116884452414, -5.717097954277069682, -8.283357778048664244 ) ) ;
#6061=CARTESIAN_POINT ( 'NONE',  ( 45.00000000000000711, -16.03270077640482683, -5.537981825772250843 ) ) ;
#6064=CARTESIAN_POINT ( 'NONE',  ( 26.75784435724945709, -6.993777436889428323, -4.533357778048668685 ) ) ;
#6067=CARTESIAN_POINT ( 'NONE',  ( 25.77727992838053339, -5.625024813964539128, -7.939653947423662927 ) ) ;
#6070=CARTESIAN_POINT ( 'NONE',  ( 26.04653150877178902, -5.151432644682725659, -3.575219446611406227 ) ) ;
#6075=VECTOR ( 'NONE', #319, 1000.000000000000000 ) ;
#6078=CARTESIAN_POINT ( 'NONE',  ( 32.54503264317084188, -5.369756224683081669, -3.627061608673667781 ) ) ;
#6081=DIRECTION ( 'NONE',  ( 0.000000000000000000, -1.000000000000000000, -3.469446951953614189E-16 ) ) ;
#6085=CARTESIAN_POINT ( 'NONE',  ( 25.86833963875586306, -3.039313213345869791, -4.705209693361160461 ) ) ;
#6087=CARTESIAN_POINT ( 'NONE',  ( 25.96861057204955259, -6.167300557297518360, -7.540293452860097112 ) ) ;
#6089=CARTESIAN_POINT ( 'NONE',  ( 26.87106449706838873, -6.053357334259913181, -3.627061608673667781 ) ) ;
#6092=EDGE_LOOP ( 'NONE', ( #7675, #6009 ) ) ;
#6100=CARTESIAN_POINT ( 'NONE',  ( -13.00000000000000178, 1.592040838891559293E-15, -10.50000000000000000 ) ) ;
#6102=CARTESIAN_POINT ( 'NONE',  ( 23.00000000000000000, -16.21813761408365195, -13.00000000000000178 ) ) ;
#6107=DIRECTION ( 'NONE',  ( 0.7999999999999999334, -0.6000000000000001998, 0.000000000000000000 ) ) ;
#6108=ORIENTED_EDGE ( 'NONE', *, *, #14588, .T. ) ;
#6109=CARTESIAN_POINT ( 'NONE',  ( 26.95740407890011170, -7.307093047852763590, -6.453230759126468818 ) ) ;
#6111=EDGE_CURVE ( 'NONE', #8674, #11419, #7584, .T. ) ;
#6113=CARTESIAN_POINT ( 'NONE',  ( 30.45035428628836627, -2.914368949527523789, -8.283357778048658915 ) ) ;
#6116=ORIENTED_EDGE ( 'NONE', *, *, #14797, .T. ) ;
#6117=AXIS2_PLACEMENT_3D ( 'NONE', #4101, #2746, #8267 ) ;
#6118=CARTESIAN_POINT ( 'NONE',  ( -25.74999999999999645, -16.21813761408365195, 0.000000000000000000 ) ) ;
#6119=CARTESIAN_POINT ( 'NONE',  ( 31.80137159822941939, -6.386132006154467078, -4.533357778048668685 ) ) ;
#6129=B_SPLINE_CURVE_WITH_KNOTS ( 'NONE', 3,
 ( #93, #9760, #1548, #13697, #11117, #7081, #5689, #1280, #2894, #3990, #1451, #9589, #17967, #4178, #15050, #4345 ),
 .UNSPECIFIED., .F., .F.,
 ( 4, 2, 2, 2, 2, 2, 2, 4 ),
 ( 0.000000000000000000, 0.0008414457502979328513, 0.001262168625446899277, 0.001682891500595865703, 0.002103614375744832128, 0.002524337250893798554, 0.002945060126042764979, 0.003365783001191731405 ),
 .UNSPECIFIED. ) ;
#6130=CARTESIAN_POINT ( 'NONE',  ( 28.74176732417158320, -7.092112515190875044, -5.783357778048657138 ) ) ;
#6147=VECTOR ( 'NONE', #4005, 1000.000000000000000 ) ;
#6155=CARTESIAN_POINT ( 'NONE',  ( -11.16099250167134826, 15.37423824781781079, -16.67067991271537863 ) ) ;
#6156=CARTESIAN_POINT ( 'NONE',  ( -28.92121476417970882, -18.25996810291579209, -13.46562832783231478 ) ) ;
#6158=CARTESIAN_POINT ( 'NONE',  ( 33.40745134805642635, -4.011910736534825439, -3.283357778048664688 ) ) ;
#6160=CARTESIAN_POINT ( 'NONE',  ( -27.17934203385504333, -30.00000000000000355, -12.00000000000000000 ) ) ;
#6167=CARTESIAN_POINT ( 'NONE',  ( 25.58373587974369201, -2.446631813008643075, -5.783357778048658027 ) ) ;
#6173=EDGE_LOOP ( 'NONE', ( #2459, #5017, #9780, #6965, #6822, #11090 ) ) ;
#6174=CARTESIAN_POINT ( 'NONE',  ( 29.35089333861488115, -5.954459450865362768, -8.283357778048664244 ) ) ;
#6175=CARTESIAN_POINT ( 'NONE',  ( 30.78070346053490880, -6.209293581256383199, -4.705209693361168455 ) ) ;
#6178=CARTESIAN_POINT ( 'NONE',  ( 30.71189515440122975, -6.854751018602581958, -5.783357778048663356 ) ) ;
#6183=CARTESIAN_POINT ( 'NONE',  ( 28.76238721243587193, -5.825490297734302381, -3.627061608673667781 ) ) ;
#6184=FACE_OUTER_BOUND ( 'NONE', #3876, .T. ) ;
#6185=CARTESIAN_POINT ( 'NONE',  ( 27.50903986916043920, -7.240631829073577386, -6.453230759126468818 ) ) ;
#6194=DIRECTION ( 'NONE',  ( 1.000000000000000000, 0.000000000000000000, 0.000000000000000000 ) ) ;
#6195=EDGE_CURVE ( 'NONE', #1319, #7967, #12665, .T. ) ;
#6203=DIRECTION ( 'NONE',  ( 0.000000000000000000, 0.000000000000000000, 1.000000000000000000 ) ) ;
#6206=CARTESIAN_POINT ( 'NONE',  ( 29.30958546476020743, -4.505622649006972402, -8.283357778048662468 ) ) ;
#6209=LINE ( 'NONE', #11818, #14162 ) ;
#6215=EDGE_CURVE ( 'NONE', #2334, #4359, #17949, .T. ) ;
#6228=EDGE_CURVE ( 'NONE', #11475, #3307, #11385, .T. ) ;
#6231=DIRECTION ( 'NONE',  ( 0.6000000000000001998, -0.7999999999999999334, 0.000000000000000000 ) ) ;
#6233=CARTESIAN_POINT ( 'NONE',  ( -5.500000000000000888, -20.49999999999999645, -12.00000000000000000 ) ) ;
#6236=ADVANCED_FACE ( 'NONE', ( #16759 ), #5767, .T. ) ;
#6244=CARTESIAN_POINT ( 'NONE',  ( 21.42601376483257880, 2.765314980223224417, -6.000000000000000000 ) ) ;
#6245=CARTESIAN_POINT ( 'NONE',  ( -25.01192583800304448, -22.13892749297381002, -14.47384481777684151 ) ) ;
#6256=ORIENTED_EDGE ( 'NONE', *, *, #3942, .T. ) ;
#6257=CARTESIAN_POINT ( 'NONE',  ( 27.61527553138257574, -4.709753535998224550, -7.939653947423662039 ) ) ;
#6261=CARTESIAN_POINT ( 'NONE',  ( 26.31556265977298992, -7.384422263489805793, -5.783357778048663356 ) ) ;
#6263=CARTESIAN_POINT ( 'NONE',  ( -34.91600907648203389, -11.88801210197604341, -12.00000000000000000 ) ) ;
#6264=CARTESIAN_POINT ( 'NONE',  ( 30.76748005699505129, -4.329975141788874993, -7.939653947423662039 ) ) ;
#6265=VERTEX_POINT ( 'NONE', #1625 ) ;
#6270=CARTESIAN_POINT ( 'NONE',  ( 30.96820195323705605, -2.125071739898741097, -7.033357778048658027 ) ) ;
#6273=EDGE_CURVE ( 'NONE', #761, #1670, #11225, .T. ) ;
#6274=CARTESIAN_POINT ( 'NONE',  ( 27.30005507882132676, -4.747731375419166788, -3.627061608673664672 ) ) ;
#6276=CARTESIAN_POINT ( 'NONE',  ( 27.49335874655903567, -6.905162478240574053, -7.033357778048666908 ) ) ;
#6283=FACE_OUTER_BOUND ( 'NONE', #4542, .T. ) ;
#6288=CARTESIAN_POINT ( 'NONE',  ( 15.92260893619738837, -28.39189527176317540, 0.000000000000000000 ) ) ;
#6291=ORIENTED_EDGE ( 'NONE', *, *, #10457, .F. ) ;
#6293=EDGE_CURVE ( 'NONE', #2108, #11560, #10947, .T. ) ;
#6294=CARTESIAN_POINT ( 'NONE',  ( 30.75815651034531584, -7.238725614818142695, -5.783357778048669573 ) ) ;
#6297=DIRECTION ( 'NONE',  ( 0.000000000000000000, 1.000000000000000000, 0.000000000000000000 ) ) ;
#6305=ORIENTED_EDGE ( 'NONE', *, *, #5084, .F. ) ;
#6307=ORIENTED_EDGE ( 'NONE', *, *, #17118, .F. ) ;
#6309=CARTESIAN_POINT ( 'NONE',  ( 26.01652455409633902, -4.902371455920928156, -5.783357778048663356 ) ) ;
#6328=VERTEX_POINT ( 'NONE', #15091 ) ;
#6333=ORIENTED_EDGE ( 'NONE', *, *, #1569, .T. ) ;
#6335=CARTESIAN_POINT ( 'NONE',  ( -27.11285657029384666, -20.94160726625447211, -13.95434672273383114 ) ) ;
#6338=CARTESIAN_POINT ( 'NONE',  ( 32.83754810739939956, -9.116730809865838836, -5.783357778048662468 ) ) ;
#6342=CARTESIAN_POINT ( 'NONE',  ( 29.69163902039066372, -1.941513746749485847, -6.453230759126468818 ) ) ;
#6345=CARTESIAN_POINT ( 'NONE',  ( 28.14933959732260149, -3.391468297350501260, -7.939653947423660263 ) ) ;
#6347=EDGE_LOOP ( 'NONE', ( #1795, #7350, #16181, #3014, #9027, #402 ) ) ;
#6353=( BOUNDED_CURVE ( )  B_SPLINE_CURVE ( 3, ( #10109, #10208, #15755, #10290 ),
 .UNSPECIFIED., .F., .T. ) 
 B_SPLINE_CURVE_WITH_KNOTS ( ( 4, 4 ),
 ( 0.000000000000000000, 3.141592653589793116 ),
 .UNSPECIFIED. ) 
 CURVE ( )  GEOMETRIC_REPRESENTATION_ITEM ( )  RATIONAL_B_SPLINE_CURVE ( ( 1.000000000000000000, 0.3333333333333333703, 0.3333333333333333703, 1.000000000000000000 ) ) 
 REPRESENTATION_ITEM ( '' )  );
#6356=CARTESIAN_POINT ( 'NONE',  ( 31.51621784984448738, -6.120678622607529817, -6.861505862736166250 ) ) ;
#6360=CARTESIAN_POINT ( 'NONE',  ( -35.46635924378174565, -16.45598204045937152, -11.37070560279562059 ) ) ;
#6362=CARTESIAN_POINT ( 'NONE',  ( 32.29295089585319545, -5.599999616269980329, -3.283357778048667797 ) ) ;
#6365=CARTESIAN_POINT ( 'NONE',  ( 26.36761712467744090, -6.740983333149474177, -4.705209693361168455 ) ) ;
#6366=CARTESIAN_POINT ( 'NONE',  ( 25.90934487712385348, 0.1208734971681838660, -5.783357778048663356 ) ) ;
#6367=CARTESIAN_POINT ( 'NONE',  ( 30.37154917142620292, -2.923863409590206519, -8.283357778048660691 ) ) ;
#6386=CARTESIAN_POINT ( 'NONE',  ( 28.04870365451522218, -4.657534006690712935, -8.283357778048662468 ) ) ;
#6406=AXIS2_PLACEMENT_3D ( 'NONE', #3295, #11518, #16910 ) ;
#6410=CARTESIAN_POINT ( 'NONE',  ( 32.08959525433819238, -2.916745304588811649, -7.939653947423660263 ) ) ;
#6411=EDGE_CURVE ( 'NONE', #11056, #3273, #7030, .T. ) ;
#6414=CARTESIAN_POINT ( 'NONE',  ( 28.60033944477555323, -4.591072787911525843, -8.283357778048662468 ) ) ;
#6415=CARTESIAN_POINT ( 'NONE',  ( -2.016448651773435938E-27, -20.49999999999999645, -13.00000000000000178 ) ) ;
#6417=CARTESIAN_POINT ( 'NONE',  ( 36.27615609941022257, -23.17738945083361557, 0.000000000000000000 ) ) ;
#6418=CARTESIAN_POINT ( 'NONE',  ( 27.73348320195396965, -4.695511846111656062, -3.283357778048664688 ) ) ;
#6426=EDGE_LOOP ( 'NONE', ( #15768, #866, #6943, #14731 ) ) ;
#6434=CARTESIAN_POINT ( 'NONE',  ( 31.35480929215617252, -6.439933945126671055, -7.033357778048666908 ) ) ;
#6439=CARTESIAN_POINT ( 'NONE',  ( 25.78518620311324838, -3.676302093007511651, -7.939653947423660263 ) ) ;
#6444=CARTESIAN_POINT ( 'NONE',  ( 32.67619606237177265, -1.592130426037603907, -5.783357778048658027 ) ) ;
#6450=EDGE_CURVE ( 'NONE', #512, #8562, #8749, .T. ) ;
#6451=ORIENTED_EDGE ( 'NONE', *, *, #3385, .T. ) ;
#6454=CARTESIAN_POINT ( 'NONE',  ( 33.30246708102489350, -5.905470865888903020, -4.705209693361168455 ) ) ;
#6458=LINE ( 'NONE', #742, #1816 ) ;
#6460=DIRECTION ( 'NONE',  ( 0.000000000000000000, 0.000000000000000000, 1.000000000000000000 ) ) ;
#6461=CARTESIAN_POINT ( 'NONE',  ( 30.58169613980036772, -2.898544849976259385, -3.283357778048662023 ) ) ;
#6466=AXIS2_PLACEMENT_3D ( 'NONE', #16364, #8090, #4009 ) ;
#6469=CARTESIAN_POINT ( 'NONE',  ( 17.88061427385022739, 10.54987872837076601, -15.87467694953868502 ) ) ;
#6475=ADVANCED_FACE ( 'NONE', ( #16726, #16920 ), #11439, .T. ) ;
#6484=CARTESIAN_POINT ( 'NONE',  ( 29.21955148510287614, -5.970283550416647600, -3.283357778048667797 ) ) ;
#6485=CARTESIAN_POINT ( 'NONE',  ( -3.347071143357316814, -15.22052928361022950, -17.00000000000000000 ) ) ;
#6488=CARTESIAN_POINT ( 'NONE',  ( -3.538288549924106796, -15.34800872113743431, -13.00000000000000178 ) ) ;
#6493=ORIENTED_EDGE ( 'NONE', *, *, #4285, .F. ) ;
#6497=VERTEX_POINT ( 'NONE', #1770 ) ;
#6500=CARTESIAN_POINT ( 'NONE',  ( 7.499998387031003411, -20.49508120620799900, -6.000000000000000000 ) ) ;
#6501=CARTESIAN_POINT ( 'NONE',  ( 32.67619606237177265, -1.592130426037603907, -5.783357778048658027 ) ) ;
#6503=CARTESIAN_POINT ( 'NONE',  ( 28.76992167940542799, -7.088720471389836852, -6.453230759126468818 ) ) ;
#6504=PLANE ( 'NONE',  #9804 ) ;
#6510=CARTESIAN_POINT ( 'NONE',  ( -2.016448651773435938E-27, -20.49999999999999645, -12.00000000000000000 ) ) ;
#6511=CARTESIAN_POINT ( 'NONE',  ( -8.632250723006720250, -18.84644399697197770, -13.00000000000000178 ) ) ;
#6512=CARTESIAN_POINT ( 'NONE',  ( 26.16860980394290337, -3.430234601869349920, -3.283357778048662023 ) ) ;
#6514=EDGE_LOOP ( 'NONE', ( #15404, #9325, #16717, #7233 ) ) ;
#6515=ADVANCED_FACE ( 'NONE', ( #7299 ), #14005, .T. ) ;
#6526=CARTESIAN_POINT ( 'NONE',  ( 26.31556265977298992, -7.384422263489805793, -5.783357778048663356 ) ) ;
#6527=CARTESIAN_POINT ( 'NONE',  ( 26.51200394741821498, -4.842675973971495296, -7.939653947423662039 ) ) ;
#6530=CARTESIAN_POINT ( 'NONE',  ( 31.65190802758064592, -5.477360103042387074, -7.939653947423664704 ) ) ;
#6533=DIRECTION ( 'NONE',  ( 0.9928203230275512992, 0.1196152422706614898, -0.000000000000000000 ) ) ;
#6537=VERTEX_POINT ( 'NONE', #13093 ) ;
#6539=CARTESIAN_POINT ( 'NONE',  ( 27.71165237056504793, -5.952083095804076684, -7.939653947423662927 ) ) ;
#6543=CARTESIAN_POINT ( 'NONE',  ( 30.61177514885987350, -5.802548093181622235, -8.283357778048662468 ) ) ;
#6547=CYLINDRICAL_SURFACE ( 'NONE', #3676, 2.749999999999992006 ) ;
#6551=EDGE_CURVE ( 'NONE', #14662, #17553, #9511, .T. ) ;
#6552=CARTESIAN_POINT ( 'NONE',  ( 5.500000000000000888, -20.49999999999999645, -12.00000000000000000 ) ) ;
#6557=CARTESIAN_POINT ( 'NONE',  ( 32.93470988637010066, -5.949778345213319497, -6.861505862736167138 ) ) ;
#6560=CARTESIAN_POINT ( 'NONE',  ( 26.27749392786457250, -6.324743385012029151, -8.283357778048662468 ) ) ;
#6563=FACE_OUTER_BOUND ( 'NONE', #1446, .T. ) ;
#6576=CARTESIAN_POINT ( 'NONE',  ( -7.499998387031003411, -20.49508120620799900, -12.00000000000000000 ) ) ;
#6579=CARTESIAN_POINT ( 'NONE',  ( 29.65098506949083301, -2.583579140294649523, -4.705209693361160461 ) ) ;
#6580=CARTESIAN_POINT ( 'NONE',  ( 30.40088504037531791, -1.856063607844930852, -6.453230759126464378 ) ) ;
#6581=PLANE ( 'NONE',  #13316 ) ;
#6588=ORIENTED_EDGE ( 'NONE', *, *, #9344, .F. ) ;
#6589=VERTEX_POINT ( 'NONE', #672 ) ;
#6591=ADVANCED_FACE ( 'NONE', ( #4742 ), #14560, .F. ) ;
#6598=CARTESIAN_POINT ( 'NONE',  ( 26.31556265977298992, -7.384422263489805793, -5.783357778048663356 ) ) ;
#6607=AXIS2_PLACEMENT_3D ( 'NONE', #3364, #13154, #7538 ) ;
#6608=CARTESIAN_POINT ( 'NONE',  ( 33.58707084003705745, -6.498152266226123963, -5.783357778048669573 ) ) ;
#6613=DIRECTION ( 'NONE',  ( 0.000000000000000000, 0.000000000000000000, -1.000000000000000000 ) ) ;
#6614=AXIS2_PLACEMENT_3D ( 'NONE', #2351, #13660, #9308 ) ;
#6617=CARTESIAN_POINT ( 'NONE',  ( 29.51982165028991645, -6.361204938940122844, -4.705209693361168455 ) ) ;
#6621=DIRECTION ( 'NONE',  ( 0.9928203230275512992, 0.1196152422706614898, -0.000000000000000000 ) ) ;
#6624=CARTESIAN_POINT ( 'NONE',  ( 30.54048978798443059, -6.538043363838207611, -4.533357778048668685 ) ) ;
#6629=DIRECTION ( 'NONE',  ( -0.000000000000000000, -0.000000000000000000, -1.000000000000000000 ) ) ;
#6630=CARTESIAN_POINT ( 'NONE',  ( 7.345582307948228973, 16.91090888051954977, -16.91488491921997195 ) ) ;
#6638=CYLINDRICAL_SURFACE ( 'NONE', #19, 2.499999999999999112 ) ;
#6640=CARTESIAN_POINT ( 'NONE',  ( 45.50000000000000000, -16.03270077640482683, -5.537981825772250843 ) ) ;
#6644=CARTESIAN_POINT ( 'NONE',  ( 32.91278983782564183, -5.325448745358647429, -7.939653947423662927 ) ) ;
#6645=CARTESIAN_POINT ( 'NONE',  ( -3.538288549924106796, -15.34800872113743431, -16.99955934415556769 ) ) ;
#6646=VERTEX_POINT ( 'NONE', #3479 ) ;
#6647=CARTESIAN_POINT ( 'NONE',  ( 33.42946061375642586, -6.517141185936593750, -5.783357778048668685 ) ) ;
#6655=EDGE_CURVE ( 'NONE', #8205, #17076, #4316, .T. ) ;
#6660=DIRECTION ( 'NONE',  ( 0.000000000000000000, 0.000000000000000000, 1.000000000000000000 ) ) ;
#6663=( BOUNDED_CURVE ( )  B_SPLINE_CURVE ( 2, ( #11086, #5746, #16839, #4402, #10463, #687, #1964, #10194, #3401 ),
 .UNSPECIFIED., .F., .T. ) 
 B_SPLINE_CURVE_WITH_KNOTS ( ( 3, 2, 2, 2, 3 ),
 ( 0.7500000000000000000, 0.7564102564102563875, 0.7692307692307692735, 0.7820512820512820484, 0.7884615384615384359 ),
 .UNSPECIFIED. ) 
 CURVE ( )  GEOMETRIC_REPRESENTATION_ITEM ( )  RATIONAL_B_SPLINE_CURVE ( ( 0.9330127018922194093, 0.9330127018922194093, 1.000000000000000000, 0.8660254037844387076, 1.000000000000000000, 0.8660254037844387076, 1.000000000000000000, 0.9330127018922194093, 0.9330127018922194093 ) ) 
 REPRESENTATION_ITEM ( '' )  );
#6665=CARTESIAN_POINT ( 'NONE',  ( -35.62429925076629189, -17.76690233603958902, -0.5379818257722508434 ) ) ;
#6668=CARTESIAN_POINT ( 'NONE',  ( 28.91547068018125799, -2.672194098943493135, -6.861505862736158257 ) ) ;
#6669=DIRECTION ( 'NONE',  ( 0.000000000000000000, 0.000000000000000000, -1.000000000000000000 ) ) ;
#6673=EDGE_CURVE ( 'NONE', #7694, #5110, #9101, .T. ) ;
#6686=VECTOR ( 'NONE', #14611, 1000.000000000000000 ) ;
#6688=CARTESIAN_POINT ( 'NONE',  ( 27.58784498402260610, -7.231137369010889770, -6.453230759126474148 ) ) ;
#6697=CARTESIAN_POINT ( 'NONE',  ( 32.29974222271236073, -2.891426744974864071, -3.627061608673662008 ) ) ;
#6700=AXIS2_PLACEMENT_3D ( 'NONE', #2045, #7571, #2878 ) ;
#6706=CARTESIAN_POINT ( 'NONE',  ( 27.09860475545177039, -3.518061095420291995, -3.627061608673662896 ) ) ;
#6710=DIRECTION ( 'NONE',  ( 0.9928203230275510771, 0.1196152422706614621, -0.000000000000000000 ) ) ;
#6713=CARTESIAN_POINT ( 'NONE',  ( 27.24942365487322959, -6.207645047004941574, -3.283357778048667797 ) ) ;
#6723=VECTOR ( 'NONE', #1327, 1000.000000000000227 ) ;
#6727=CARTESIAN_POINT ( 'NONE',  ( -26.11885528537984413, -10.78654967147420329, -14.20677827292374040 ) ) ;
#6732=CARTESIAN_POINT ( 'NONE',  ( 31.03886041246737548, -3.043338102658604161, -3.627061608673662008 ) ) ;
#6738=CARTESIAN_POINT ( 'NONE',  ( 26.03726795043090547, -3.446058701420613879, -8.283357778048658915 ) ) ;
#6749=EDGE_CURVE ( 'NONE', #3447, #16316, #6129, .T. ) ;
#6750=( BOUNDED_CURVE ( )  B_SPLINE_CURVE ( 2, ( #6938, #8570, #13919, #11364, #15468, #1328, #4143, #6852, #2778 ),
 .UNSPECIFIED., .F., .T. ) 
 B_SPLINE_CURVE_WITH_KNOTS ( ( 3, 2, 2, 2, 3 ),
 ( 0.8269230769230769829, 0.8333333333333333703, 0.8461538461538461453, 0.8589743589743589203, 0.8653846153846154188 ),
 .UNSPECIFIED. ) 
 CURVE ( )  GEOMETRIC_REPRESENTATION_ITEM ( )  RATIONAL_B_SPLINE_CURVE ( ( 0.9330127018922192983, 0.9330127018922198534, 1.000000000000000000, 0.8660254037844387076, 1.000000000000000000, 0.8660254037844387076, 1.000000000000000000, 0.9330127018922187432, 0.9330127018922192983 ) ) 
 REPRESENTATION_ITEM ( '' )  );
#6758=EDGE_CURVE ( 'NONE', #1259, #13758, #12508, .T. ) ;
#6761=CARTESIAN_POINT ( 'NONE',  ( 28.89355063163679915, -2.047864499088824175, -5.783357778048658027 ) ) ;
#6769=CARTESIAN_POINT ( 'NONE',  ( 27.27683486999669427, -2.232449958253242883, -5.783357778048658027 ) ) ;
#6772=ORIENTED_EDGE ( 'NONE', *, *, #3245, .F. ) ;
#6774=FACE_OUTER_BOUND ( 'NONE', #13628, .T. ) ;
#6775=ORIENTED_EDGE ( 'NONE', *, *, #16237, .T. ) ;
#6782=CARTESIAN_POINT ( 'NONE',  ( 29.98885399772409954, -6.604504582617394703, -4.533357778048668685 ) ) ;
#6787=CARTESIAN_POINT ( 'NONE',  ( 28.92482766011098150, -14.18604173879621477, -13.46461621778217577 ) ) ;
#6788=FACE_OUTER_BOUND ( 'NONE', #11326, .T. ) ;
#6789=VERTEX_POINT ( 'NONE', #12599 ) ;
#6792=CARTESIAN_POINT ( 'NONE',  ( 32.50119254608192421, -4.121097024973739309, -3.627061608673664672 ) ) ;
#6795=LINE ( 'NONE', #17888, #9767 ) ;
#6800=CARTESIAN_POINT ( 'NONE',  ( 27.08121146544255353, -6.028038774645947839, -7.939653947423662927 ) ) ;
#6801=DIRECTION ( 'NONE',  ( 0.000000000000000000, 0.000000000000000000, 1.000000000000000000 ) ) ;
#6806=EDGE_CURVE ( 'NONE', #15344, #10032, #9856, .T. ) ;
#6807=CARTESIAN_POINT ( 'NONE',  ( 28.79241808379989465, -7.086010098929231837, -5.113484796970862334 ) ) ;
#6808=CARTESIAN_POINT ( 'NONE',  ( 32.60321786976872005, -6.626883982076972046, -5.783357778048663356 ) ) ;
#6810=CARTESIAN_POINT ( 'NONE',  ( 28.72045243349238675, -6.030415129707233035, -8.283357778048662468 ) ) ;
#6813=CARTESIAN_POINT ( 'NONE',  ( 31.93198502805756789, -2.935734224299280548, -7.939653947423660263 ) ) ;
#6815=CARTESIAN_POINT ( 'NONE',  ( 26.70901672940806648, -4.818939824437135755, -8.283357778048662468 ) ) ;
#6816=DIRECTION ( 'NONE',  ( -0.1196152422706611984, 0.9928203230275510771, 0.000000000000000000 ) ) ;
#6821=CARTESIAN_POINT ( 'NONE',  ( -29.20850947011023280, -15.38975055298431549, -13.38439523458337099 ) ) ;
#6822=ORIENTED_EDGE ( 'NONE', *, *, #15074, .T. ) ;
#6824=CARTESIAN_POINT ( 'NONE',  ( 29.66420847303068697, -4.462897579762144851, -7.939653947423662039 ) ) ;
#6826=ORIENTED_EDGE ( 'NONE', *, *, #608, .F. ) ;
#6827=CARTESIAN_POINT ( 'NONE',  ( 27.60595198473284384, -7.618504009027492252, -5.783357778048669573 ) ) ;
#6828=EDGE_CURVE ( 'NONE', #5257, #9208, #11742, .T. ) ;
#6832=CARTESIAN_POINT ( 'NONE',  ( 24.62797819841904001, -22.25577170577939157, -14.56336204217505426 ) ) ;
#6834=CARTESIAN_POINT ( 'NONE',  ( -45.00000000000000711, -19.03270077640483038, -0.5379818257722508434 ) ) ;
#6843=CARTESIAN_POINT ( 'NONE',  ( 28.93739072872572393, -3.296523698798161650, -7.939653947423660263 ) ) ;
#6852=CARTESIAN_POINT ( 'NONE',  ( 26.04410741498555382, -2.380969272135942560, -5.113484796970857893 ) ) ;
#6855=ORIENTED_EDGE ( 'NONE', *, *, #2531, .F. ) ;
#6871=CARTESIAN_POINT ( 'NONE',  ( 29.66420847303068697, -4.462897579762144851, -7.939653947423662039 ) ) ;
#6873=ORIENTED_EDGE ( 'NONE', *, *, #1767, .T. ) ;
#6876=DIRECTION ( 'NONE',  ( 1.000000000000000000, -1.734723475976805517E-15, 0.000000000000000000 ) ) ;
#6881=CARTESIAN_POINT ( 'NONE',  ( 28.38593337277646711, -7.124786616671554107, -5.783357778048668685 ) ) ;
#6886=CARTESIAN_POINT ( 'NONE',  ( -20.00000000000000355, 7.999999999999996447, 0.000000000000000000 ) ) ;
#6891=CARTESIAN_POINT ( 'NONE',  ( 29.11066736118121057, -3.075774767273946608, -8.283357778048658915 ) ) ;
#6894=CARTESIAN_POINT ( 'NONE',  ( 29.41022140756759029, -3.239556939666760726, -7.939653947423660263 ) ) ;
#6895=CIRCLE ( 'NONE', #17053, 2.749999999999988454 ) ;
#6908=DIRECTION ( 'NONE',  ( 0.9928203230275512992, 0.1196152422706614898, -0.000000000000000000 ) ) ;
#6910=CARTESIAN_POINT ( 'NONE',  ( 30.78487334700428235, -1.819997462563214263, -5.783357778048658915 ) ) ;
#6912=CARTESIAN_POINT ( 'NONE',  ( 25.52694003402523748, -4.961356722058193114, -8.283357778048662468 ) ) ;
#6913=CARTESIAN_POINT ( 'NONE',  ( -20.25000000000000355, -16.21813761408365195, 0.000000000000000000 ) ) ;
#6917=EDGE_CURVE ( 'NONE', #17090, #6049, #14416, .T. ) ;
#6918=CARTESIAN_POINT ( 'NONE',  ( 21.03881409870396624, -22.15596512169676302, -15.31966522629967464 ) ) ;
#6923=ORIENTED_EDGE ( 'NONE', *, *, #17453, .F. ) ;
#6929=FACE_OUTER_BOUND ( 'NONE', #7004, .T. ) ;
#6930=CARTESIAN_POINT ( 'NONE',  ( 31.06530721954707985, -6.801974981593605030, -5.783357778048669573 ) ) ;
#6938=CARTESIAN_POINT ( 'NONE',  ( 26.92924972366625980, -7.310485091653801781, -5.783357778048657138 ) ) ;
#6941=ADVANCED_FACE ( 'NONE', ( #458, #630 ), #8967, .T. ) ;
#6942=VERTEX_POINT ( 'NONE', #14235 ) ;
#6943=ORIENTED_EDGE ( 'NONE', *, *, #14606, .T. ) ;
#6945=DIRECTION ( 'NONE',  ( -0.000000000000000000, -0.000000000000000000, -1.000000000000000000 ) ) ;
#6952=FACE_OUTER_BOUND ( 'NONE', #7166, .T. ) ;
#6953=CARTESIAN_POINT ( 'NONE',  ( 26.01652455409633902, -4.902371455920928156, -5.783357778048663356 ) ) ;
#6958=CYLINDRICAL_SURFACE ( 'NONE', #5545, 14.00000000000000178 ) ;
#6960=CARTESIAN_POINT ( 'NONE',  ( 26.12124691615246874, -10.79952268558355755, -14.20570119594951208 ) ) ;
#6965=ORIENTED_EDGE ( 'NONE', *, *, #6828, .T. ) ;
#6966=CARTESIAN_POINT ( 'NONE',  ( 27.88665588685489993, -3.423116496867954162, -3.627061608673662008 ) ) ;
#6970=FACE_OUTER_BOUND ( 'NONE', #2864, .T. ) ;
#6972=DIRECTION ( 'NONE',  ( -0.000000000000000000, -0.000000000000000000, -1.000000000000000000 ) ) ;
#6977=CARTESIAN_POINT ( 'NONE',  ( 28.55151181693415907, -2.416235175459247486, -4.533357778048659803 ) ) ;
#6979=CARTESIAN_POINT ( 'NONE',  ( -13.00000000000000178, 1.592040838891559293E-15, -12.00000000000000000 ) ) ;
#6983=DIRECTION ( 'NONE',  ( 0.000000000000000000, -1.000000000000000000, -3.469446951953614189E-16 ) ) ;
#6984=CIRCLE ( 'NONE', #15674, 2.000000000000001776 ) ;
#6987=CARTESIAN_POINT ( 'NONE',  ( 29.54600080245929306, -4.477139269648729325, -3.283357778048664688 ) ) ;
#6988=VECTOR ( 'NONE', #8403, 1000.000000000000227 ) ;
#6989=CARTESIAN_POINT ( 'NONE',  ( 30.45225960443380231, -4.367952981209816343, -3.627061608673664672 ) ) ;
#6990=CARTESIAN_POINT ( 'NONE',  ( 28.20260476654369697, -6.819712339336020612, -7.033357778048666908 ) ) ;
#6992=DIRECTION ( 'NONE',  ( -0.000000000000000000, -0.000000000000000000, -1.000000000000000000 ) ) ;
#6996=VECTOR ( 'NONE', #1, 1000.000000000000000 ) ;
#7003=VECTOR ( 'NONE', #1195, 1000.000000000000000 ) ;
#7004=EDGE_LOOP ( 'NONE', ( #16078, #3646, #2320, #3138 ) ) ;
#7005=CARTESIAN_POINT ( 'NONE',  ( -16.75000000000000000, -16.21813761408365195, -16.03574476417183448 ) ) ;
#7007=CARTESIAN_POINT ( 'NONE',  ( 28.91547068018125799, -2.672194098943493135, -6.861505862736158257 ) ) ;
#7010=ORIENTED_EDGE ( 'NONE', *, *, #8873, .T. ) ;
#7012=CARTESIAN_POINT ( 'NONE',  ( 30.62726312072365431, -1.838986382273682718, -5.783357778048658027 ) ) ;
#7025=( BOUNDED_CURVE ( )  B_SPLINE_CURVE ( 2, ( #7417, #436, #244, #5755, #15656, #11269, #3236, #8774, #14307 ),
 .UNSPECIFIED., .F., .T. ) 
 B_SPLINE_CURVE_WITH_KNOTS ( ( 3, 2, 2, 2, 3 ),
 ( 0.8653846153846154188, 0.8717948717948718063, 0.8846153846153845812, 0.8974358974358974672, 0.9012882778258578531 ),
 .UNSPECIFIED. ) 
 CURVE ( )  GEOMETRIC_REPRESENTATION_ITEM ( )  RATIONAL_B_SPLINE_CURVE ( ( 0.9330127018922192983, 0.9330127018922198534, 1.000000000000000000, 0.8660254037844387076, 1.000000000000000000, 0.8660254037844387076, 1.000000000000000000, 0.9597425536373320742, 0.9436786787937823107 ) ) 
 REPRESENTATION_ITEM ( '' )  );
#7027=CIRCLE ( 'NONE', #15426, 14.00000000000000178 ) ;
#7030=LINE ( 'NONE', #12548, #5740 ) ;
#7031=VERTEX_POINT ( 'NONE', #2185 ) ;
#7032=VECTOR ( 'NONE', #17776, 1000.000000000000227 ) ;
#7036=ORIENTED_EDGE ( 'NONE', *, *, #16651, .T. ) ;
#7039=CARTESIAN_POINT ( 'NONE',  ( 27.89118264539014547, -6.557423775948280742, -6.861505862736167138 ) ) ;
#7040=CARTESIAN_POINT ( 'NONE',  ( 32.14656953781143756, -4.163822094218565972, -3.283357778048664688 ) ) ;
#7046=AXIS2_PLACEMENT_3D ( 'NONE', #6640, #847, #9443 ) ;
#7053=AXIS2_PLACEMENT_3D ( 'NONE', #1980, #5119, #13211 ) ;
#7057=LINE ( 'NONE', #16851, #12120 ) ;
#7062=EDGE_CURVE ( 'NONE', #3307, #16117, #17393, .T. ) ;
#7064=ORIENTED_EDGE ( 'NONE', *, *, #14845, .T. ) ;
#7066=EDGE_CURVE ( 'NONE', #4693, #15606, #4899, .T. ) ;
#7068=CARTESIAN_POINT ( 'NONE',  ( 17.15697743806116549, -13.99005979112454767, -15.97644891051836957 ) ) ;
#7069=DIRECTION ( 'NONE',  ( 0.000000000000000000, 0.000000000000000000, 1.000000000000000000 ) ) ;
#7073=DIRECTION ( 'NONE',  ( -0.1196152422706621143, -0.9928203230275509661, 0.000000000000000000 ) ) ;
#7077=ORIENTED_EDGE ( 'NONE', *, *, #14445, .T. ) ;
#7080=CARTESIAN_POINT ( 'NONE',  ( 33.76207435632690590, -3.969185667289998332, -3.627061608673664672 ) ) ;
#7081=CARTESIAN_POINT ( 'NONE',  ( 25.78162057792670225, -2.952641328940847743, -4.882123357130833341 ) ) ;
#7084=CARTESIAN_POINT ( 'NONE',  ( 26.85044460880409645, -7.319979551716484067, -5.783357778048668685 ) ) ;
#7088=CARTESIAN_POINT ( 'NONE',  ( 27.02423718196931546, -4.780961985016209503, -3.283357778048664688 ) ) ;
#7089=ORIENTED_EDGE ( 'NONE', *, *, #13801, .F. ) ;
#7090=CARTESIAN_POINT ( 'NONE',  ( 29.19137779418881351, -4.519864338893556877, -3.627061608673664672 ) ) ;
#7091=CARTESIAN_POINT ( 'NONE',  ( -14.00000000000000178, 0.000000000000000000, -8.700000000000001066 ) ) ;
#7094=LINE ( 'NONE', #15425, #2561 ) ;
#7099=ORIENTED_EDGE ( 'NONE', *, *, #11091, .F. ) ;
#7101=DIRECTION ( 'NONE',  ( 0.000000000000000000, 0.000000000000000000, -1.000000000000000000 ) ) ;
#7102=CARTESIAN_POINT ( 'NONE',  ( 30.17644170758179101, -4.401183590806859947, -3.283357778048664688 ) ) ;
#7104=DIRECTION ( 'NONE',  ( 0.1113444980252557837, -0.9937818688019538493, 0.000000000000000000 ) ) ;
#7107=CARTESIAN_POINT ( 'NONE',  ( 30.60986983071443390, -4.348964061499348333, -3.627061608673664672 ) ) ;
#7108=CARTESIAN_POINT ( 'NONE',  ( 27.55969062878875064, -7.234529412811931515, -5.783357778048668685 ) ) ;
#7111=CARTESIAN_POINT ( 'NONE',  ( 29.82181869931131146, -4.443908660051686610, -3.627061608673664672 ) ) ;
#7112=DIRECTION ( 'NONE',  ( -0.1196152422706611984, 0.9928203230275510771, 0.000000000000000000 ) ) ;
#7116=CARTESIAN_POINT ( 'NONE',  ( 17.07932405232147488, -18.26192153598439205, -15.98801167710370663 ) ) ;
#7123=CARTESIAN_POINT ( 'NONE',  ( 26.28639176851562453, -7.142300497639897827, -6.903997060601237301 ) ) ;
#7129=CARTESIAN_POINT ( 'NONE',  ( 28.28955653359400557, -5.882457056865704637, -3.627061608673668225 ) ) ;
#7130=CARTESIAN_POINT ( 'NONE',  ( 31.92138306490751987, -2.737139032229836122, -3.283357778048662023 ) ) ;
#7136=CARTESIAN_POINT ( 'NONE',  ( -15.92260893619738837, -28.39189527176317540, -16.15082599432113142 ) ) ;
#7139=ORIENTED_EDGE ( 'NONE', *, *, #11950, .T. ) ;
#7140=ADVANCED_FACE ( 'NONE', ( #10839 ), #9487, .F. ) ;
#7141=ORIENTED_EDGE ( 'NONE', *, *, #15038, .F. ) ;
#7151=CARTESIAN_POINT ( 'NONE',  ( 26.56758885001203652, -2.317900097157796324, -5.783357778048670461 ) ) ;
#7159=( BOUNDED_CURVE ( )  B_SPLINE_CURVE ( 2, ( #11498, #9138, #5888, #14341, #7447, #3176, #11411, #1737, #12022 ),
 .UNSPECIFIED., .F., .T. ) 
 B_SPLINE_CURVE_WITH_KNOTS ( ( 3, 2, 2, 2, 3 ),
 ( 0.05769230769230770939, 0.06410256410256409687, 0.07692307692307692735, 0.08974358974358974395, 0.09615384615384617306 ),
 .UNSPECIFIED. ) 
 CURVE ( )  GEOMETRIC_REPRESENTATION_ITEM ( )  RATIONAL_B_SPLINE_CURVE ( ( 0.9330127018922194093, 0.9330127018922196314, 1.000000000000000000, 0.8660254037844387076, 1.000000000000000000, 0.8660254037844387076, 1.000000000000000000, 0.9330127018922191873, 0.9330127018922194093 ) ) 
 REPRESENTATION_ITEM ( '' )  );
#7165=ADVANCED_FACE ( 'NONE', ( #6952 ), #1427, .F. ) ;
#7166=EDGE_LOOP ( 'NONE', ( #16377, #2177, #9802, #5450 ) ) ;
#7169=CARTESIAN_POINT ( 'NONE',  ( 26.36761712467744090, -6.740983333149474177, -4.705209693361168455 ) ) ;
#7178=UNCERTAINTY_MEASURE_WITH_UNIT (LENGTH_MEASURE( 1.000000000000000082E-05 ), #10875, 'distance_accuracy_value', 'NONE');
#7180=CARTESIAN_POINT ( 'NONE',  ( 28.99445422935450267, -6.424501337975009996, -6.861505862736166250 ) ) ;
#7183=CARTESIAN_POINT ( 'NONE',  ( 26.06962060539356330, -5.343074812781621219, -3.590724507760069795 ) ) ;
#7192=DIRECTION ( 'NONE',  ( 1.000000000000000000, 0.000000000000000000, 0.000000000000000000 ) ) ;
#7195=AXIS2_PLACEMENT_3D ( 'NONE', #995, #3436, #3703 ) ;
#7196=CARTESIAN_POINT ( 'NONE',  ( 26.49878054387835746, -2.963357534503999968, -4.705209693361160461 ) ) ;
#7198=CARTESIAN_POINT ( 'NONE',  ( 30.27725608814395031, -6.896919580145944195, -5.783357778048668685 ) ) ;
#7202=AXIS2_PLACEMENT_3D ( 'NONE', #5417, #17808, #5070 ) ;
#7211=ORIENTED_EDGE ( 'NONE', *, *, #2485, .T. ) ;
#7217=CARTESIAN_POINT ( 'NONE',  ( 33.69269431359690969, -6.158264969628857166, -4.533357778048668685 ) ) ;
#7220=CARTESIAN_POINT ( 'NONE',  ( 31.51612863268893960, -4.239777773060436239, -3.283357778048664688 ) ) ;
#7222=DIRECTION ( 'NONE',  ( 1.000000000000000000, 0.000000000000000000, 0.000000000000000000 ) ) ;
#7225=CARTESIAN_POINT ( 'NONE',  ( 30.45719375084302527, -1.849279520242854469, -5.113484796970851676 ) ) ;
#7229=VERTEX_POINT ( 'NONE', #16485 ) ;
#7233=ORIENTED_EDGE ( 'NONE', *, *, #3217, .F. ) ;
#7237=FACE_OUTER_BOUND ( 'NONE', #2221, .T. ) ;
#7239=CARTESIAN_POINT ( 'NONE',  ( 27.24942365487322959, -6.207645047004940686, -3.283357778048667797 ) ) ;
#7251=ORIENTED_EDGE ( 'NONE', *, *, #11689, .T. ) ;
#7254=CARTESIAN_POINT ( 'NONE',  ( 33.68326924318660076, -3.978680127145231893, -3.283357778048664688 ) ) ;
#7257=CARTESIAN_POINT ( 'NONE',  ( -2.016448651773435938E-27, -20.49999999999999645, -6.000000000000000000 ) ) ;
#7259=CARTESIAN_POINT ( 'NONE',  ( 31.08763465596552322, -1.773323841400983758, -5.113484796970854340 ) ) ;
#7262=( BOUNDED_CURVE ( )  B_SPLINE_CURVE ( 2, ( #5671, #2707, #8583, #4326, #11012, #14118, #9569, #4417, #8498 ),
 .UNSPECIFIED., .F., .T. ) 
 B_SPLINE_CURVE_WITH_KNOTS ( ( 3, 2, 2, 2, 3 ),
 ( 0.01923076923076924918, 0.02564102564102564014, 0.03846153846153846367, 0.05128205128205128027, 0.05769230769230770939 ),
 .UNSPECIFIED. ) 
 CURVE ( )  GEOMETRIC_REPRESENTATION_ITEM ( )  RATIONAL_B_SPLINE_CURVE ( ( 0.9330127018922194093, 0.9330127018922195203, 1.000000000000000000, 0.8660254037844387076, 1.000000000000000000, 0.8660254037844387076, 1.000000000000000000, 0.9330127018922191873, 0.9330127018922194093 ) ) 
 REPRESENTATION_ITEM ( '' )  );
#7267=CARTESIAN_POINT ( 'NONE',  ( 28.86293393808771057, -2.678523738846987357, -4.705209693361161349 ) ) ;
#7269=CARTESIAN_POINT ( 'NONE',  ( 32.24155699611449677, -1.634298987580965923, -5.783357778048664244 ) ) ;
#7272=AXIS2_PLACEMENT_3D ( 'NONE', #6160, #15779, #14239 ) ;
#7276=ORIENTED_EDGE ( 'NONE', *, *, #11915, .F. ) ;
#7277=CIRCLE ( 'NONE', #11606, 5.000000000000000000 ) ;
#7281=CARTESIAN_POINT ( 'NONE',  ( -18.05564684537134568, -12.37312016356480449, -15.83930707548887895 ) ) ;
#7282=ORIENTED_EDGE ( 'NONE', *, *, #13895, .T. ) ;
#7286=CARTESIAN_POINT ( 'NONE',  ( 30.90769699326644826, -6.820963901304073929, -5.783357778048668685 ) ) ;
#7288=DIRECTION ( 'NONE',  ( 1.000000000000000000, 0.000000000000000000, 0.000000000000000000 ) ) ;
#7296=AXIS2_PLACEMENT_3D ( 'NONE', #4444, #15593, #3171 ) ;
#7299=FACE_OUTER_BOUND ( 'NONE', #2646, .T. ) ;
#7303=VERTEX_POINT ( 'NONE', #1705 ) ;
#7307=CARTESIAN_POINT ( 'NONE',  ( 26.92924972366625980, -7.310485091653801781, -5.783357778048657138 ) ) ;
#7308=CARTESIAN_POINT ( 'NONE',  ( 26.37178701114681800, -2.351687214456304353, -5.783357778048658027 ) ) ;
#7310=VECTOR ( 'NONE', #15321, 1000.000000000000227 ) ;
#7312=CARTESIAN_POINT ( 'NONE',  ( 31.24973580796908834, -6.452593224933654170, -4.533357778048668685 ) ) ;
#7316=CARTESIAN_POINT ( 'NONE',  ( 27.75966235412334981, -2.811446176820259879, -4.705209693361160461 ) ) ;
#7318=DIRECTION ( 'NONE',  ( -0.000000000000000000, -0.000000000000000000, -1.000000000000000000 ) ) ;
#7329=CARTESIAN_POINT ( 'NONE',  ( -2.016448651773435938E-27, -20.49999999999999645, -13.00000000000000178 ) ) ;
#7335=CARTESIAN_POINT ( 'NONE',  ( -20.25000000000000711, -16.21813761408365195, -13.00000000000000178 ) ) ;
#7341=VECTOR ( 'NONE', #17578, 1000.000000000000000 ) ;
#7346=CARTESIAN_POINT ( 'NONE',  ( 35.62429925076629189, -17.76690233603958902, -0.5379818257722508434 ) ) ;
#7347=ORIENTED_EDGE ( 'NONE', *, *, #2168, .F. ) ;
#7349=MECHANICAL_DESIGN_GEOMETRIC_PRESENTATION_REPRESENTATION('',(#13706),#14216);
#7350=ORIENTED_EDGE ( 'NONE', *, *, #15855, .T. ) ;
#7355=CARTESIAN_POINT ( 'NONE',  ( 15.92260893619738837, -28.39189527176317540, -12.00000000000000000 ) ) ;
#7357=DIRECTION ( 'NONE',  ( 0.9937818688019538493, -0.1113444980252557837, 0.000000000000000000 ) ) ;
#7359=CYLINDRICAL_SURFACE ( 'NONE', #4948, 2.499999999999999112 ) ;
#7362=CARTESIAN_POINT ( 'NONE',  ( 25.95846283556873502, -3.455553161483296609, -8.283357778048658915 ) ) ;
#7365=CARTESIAN_POINT ( 'NONE',  ( 33.44685390376565692, -4.007163506710925027, -7.939653947423662039 ) ) ;
#7367=DIRECTION ( 'NONE',  ( 0.000000000000000000, 0.000000000000000000, 1.000000000000000000 ) ) ;
#7368=DIRECTION ( 'NONE',  ( 0.000000000000000000, 0.000000000000000000, -1.000000000000000000 ) ) ;
#7372=VERTEX_POINT ( 'NONE', #3241 ) ;
#7377=VERTEX_POINT ( 'NONE', #8496 ) ;
#7378=CARTESIAN_POINT ( 'NONE',  ( -45.00000000000000711, 0.000000000000000000, -5.537981825772250843 ) ) ;
#7380=CARTESIAN_POINT ( 'NONE',  ( 27.14244485254070938, -4.766720295129625029, -7.939653947423662039 ) ) ;
#7381=CARTESIAN_POINT ( 'NONE',  ( 25.93489015466116854, -5.606035894254070229, -7.939653947423662927 ) ) ;
#7383=CARTESIAN_POINT ( 'NONE',  ( 30.65370992780335868, -5.597623261208691581, -3.627061608673667781 ) ) ;
#7384=ORIENTED_EDGE ( 'NONE', *, *, #562, .F. ) ;
#7405=CARTESIAN_POINT ( 'NONE',  ( 31.67744797322171735, -2.039621600994187656, -7.033357778048658027 ) ) ;
#7417=CARTESIAN_POINT ( 'NONE',  ( 26.01595305975170547, -2.384361315936983416, -5.783357778048670461 ) ) ;
#7418=ORIENTED_EDGE ( 'NONE', *, *, #510, .T. ) ;
#7431=ORIENTED_EDGE ( 'NONE', *, *, #8634, .T. ) ;
#7435=CARTESIAN_POINT ( 'NONE',  ( 20.00000000000000000, 7.999999999999996447, -12.00000000000000000 ) ) ;
#7438=CARTESIAN_POINT ( 'NONE',  ( -37.55714628004649569, -12.56174331051002113, -5.783357778048663356 ) ) ;
#7445=CARTESIAN_POINT ( 'NONE',  ( 26.36761712467744090, -6.740983333149474177, -4.705209693361168455 ) ) ;
#7447=CARTESIAN_POINT ( 'NONE',  ( 32.77701044293393551, -4.087866415376695706, -3.283357778048664688 ) ) ;
#7449=FACE_OUTER_BOUND ( 'NONE', #14319, .T. ) ;
#7452=CARTESIAN_POINT ( 'NONE',  ( 30.88577694472199298, -6.196634301449400084, -6.861505862736166250 ) ) ;
#7453=ORIENTED_EDGE ( 'NONE', *, *, #8915, .F. ) ;
#7455=CARTESIAN_POINT ( 'NONE',  ( 35.77680296528374271, -19.03270077640483038, -0.5379818257722512875 ) ) ;
#7457=CARTESIAN_POINT ( 'NONE',  ( 26.41562710823574278, -3.600346414165641828, -7.939653947423660263 ) ) ;
#7461=CARTESIAN_POINT ( 'NONE',  ( 28.23249303296521617, -2.754479417688857179, -4.705209693361161349 ) ) ;
#7477=CARTESIAN_POINT ( 'NONE',  ( 3.443595183066687326, -15.28297513750540837, -16.99984776326510172 ) ) ;
#7480=CARTESIAN_POINT ( 'NONE',  ( 28.16881664323205570, -6.096876348486420127, -8.283357778048662468 ) ) ;
#7481=CYLINDRICAL_SURFACE ( 'NONE', #15366, 5.000000000000001776 ) ;
#7486=VECTOR ( 'NONE', #2804, 999.9999999999998863 ) ;
#7488=CIRCLE ( 'NONE', #4872, 3.999999999999994671 ) ;
#7494=VERTEX_POINT ( 'NONE', #11834 ) ;
#7502=VERTEX_POINT ( 'NONE', #17412 ) ;
#7510=VECTOR ( 'NONE', #16679, 1000.000000000000227 ) ;
#7514=AXIS2_PLACEMENT_3D ( 'NONE', #353, #618, #11188 ) ;
#7524=CARTESIAN_POINT ( 'NONE',  ( -14.05523583925745257, 13.74128089903392613, -16.39434919531312218 ) ) ;
#7525=CARTESIAN_POINT ( 'NONE',  ( -29.25000000000000000, -16.63595338719256844, -13.37255996287877124 ) ) ;
#7533=ORIENTED_EDGE ( 'NONE', *, *, #15138, .F. ) ;
#7536=CARTESIAN_POINT ( 'NONE',  ( 27.08121146544255353, -6.028038774645947839, -7.939653947423664704 ) ) ;
#7538=DIRECTION ( 'NONE',  ( 0.9899494936611662466, -0.1414213562373111965, 0.000000000000000000 ) ) ;
#7543=CARTESIAN_POINT ( 'NONE',  ( -16.75000000000000000, -16.21813761408365195, -13.00000000000000178 ) ) ;
#7544=CARTESIAN_POINT ( 'NONE',  ( 30.90769699326645181, -6.820963901304073929, -5.783357778048668685 ) ) ;
#7549=CARTESIAN_POINT ( 'NONE',  ( 31.26353094466156080, -6.788289799823394866, -5.783357778048663356 ) ) ;
#7552=CARTESIAN_POINT ( 'NONE',  ( 27.10313151398701947, -6.652368374500619908, -6.861505862736166250 ) ) ;
#7554=CARTESIAN_POINT ( 'NONE',  ( 33.78529456515154550, -6.484467084455914687, -5.783357778048663356 ) ) ;
#7559=AXIS2_PLACEMENT_3D ( 'NONE', #3019, #8541, #7192 ) ;
#7563=EDGE_CURVE ( 'NONE', #548, #15612, #16210, .T. ) ;
#7564=ORIENTED_EDGE ( 'NONE', *, *, #14893, .F. ) ;
#7571=DIRECTION ( 'NONE',  ( 0.9928203230275512992, 0.1196152422706614898, -0.000000000000000000 ) ) ;
#7573=AXIS2_PLACEMENT_3D ( 'NONE', #399, #661, #10167 ) ;
#7575=CARTESIAN_POINT ( 'NONE',  ( 28.52524344760924180, -2.419399995203538101, -7.033357778048658027 ) ) ;
#7576=FACE_BOUND ( 'NONE', #6092, .T. ) ;
#7580=VECTOR ( 'NONE', #6107, 1000.000000000000000 ) ;
#7581=CARTESIAN_POINT ( 'NONE',  ( -13.00000000000000178, 1.592040838891559293E-15, -8.700000000000001066 ) ) ;
#7584=B_SPLINE_CURVE_WITH_KNOTS ( 'NONE', 3,
 ( #2027, #16412, #78, #11105, #1436, #13593, #7068, #13680, #4165, #12584, #12228, #9409, #8408, #17883, #2621, #9493, #15126, #15034, #10845, #3893, #12491, #13940, #3979, #1175, #9747, #13848, #17965, #8318, #8148, #6960, #2881, #12317, #1533, #4247, #1269, #163, #15300, #10925, #14950, #6787, #17802, #5322, #5675, #5409 ),
 .UNSPECIFIED., .F., .F.,
 ( 4, 2, 2, 2, 2, 2, 2, 2, 2, 2, 2, 2, 2, 2, 2, 2, 2, 2, 2, 2, 2, 4 ),
 ( 0.000000000000000000, 0.001235617314710323825, 0.001853425972065488340, 0.002471234629420653289, 0.003706851944130986655, 0.004324660601486156157, 0.004942469258841326527, 0.006178086573551669868, 0.007413703888262013209, 0.008031512545617180976, 0.008649321202972348743, 0.009884938517682682543, 0.01112055583239301808, 0.01235617314710335361, 0.01297398180445852138, 0.01359179046181369088, 0.01482740777652402121, 0.01606302509123435501, 0.01668083374858951584, 0.01729864240594468014, 0.01853425972065500180, 0.01976987703536532692 ),
 .UNSPECIFIED. ) ;
#7586=ORIENTED_EDGE ( 'NONE', *, *, #756, .F. ) ;
#7592=LINE ( 'NONE', #16207, #3562 ) ;
#7600=DIRECTION ( 'NONE',  ( 0.000000000000000000, 0.000000000000000000, 1.000000000000000000 ) ) ;
#7602=CARTESIAN_POINT ( 'NONE',  ( 26.01652455409633902, -4.902371455920928156, -5.783357778048663356 ) ) ;
#7605=CIRCLE ( 'NONE', #10488, 5.500000000000000888 ) ;
#7618=CARTESIAN_POINT ( 'NONE',  ( -19.90989778724008019, -21.66613080872904717, -15.52824432210780259 ) ) ;
#7621=CARTESIAN_POINT ( 'NONE',  ( 25.11802603177690330, -19.03270077640483038, -0.5379818257722508434 ) ) ;
#7622=AXIS2_PLACEMENT_3D ( 'NONE', #16387, #4218, #12369 ) ;
#7625=ADVANCED_FACE ( 'NONE', ( #8287 ), #13817, .F. ) ;
#7629=CARTESIAN_POINT ( 'NONE',  ( 27.72904566057427189, -3.442105416578422172, -3.627061608673662896 ) ) ;
#7638=CARTESIAN_POINT ( 'NONE',  ( 33.14902674121363901, -1.535163666906202318, -5.783357778048658915 ) ) ;
#7642=CARTESIAN_POINT ( 'NONE',  ( 25.83183225892938140, -3.369404079293177645, -7.443282702368841264 ) ) ;
#7646=CARTESIAN_POINT ( 'NONE',  ( 27.15566825608056689, -6.646038734597135011, -4.705209693361169343 ) ) ;
#7650=CARTESIAN_POINT ( 'NONE',  ( 27.45957062324739084, -6.182326487390971792, -8.283357778048664244 ) ) ;
#7662=CARTESIAN_POINT ( 'NONE',  ( 33.58707084003705745, -6.498152266226124851, -5.783357778048669573 ) ) ;
#7665=CARTESIAN_POINT ( 'NONE',  ( 29.94002636988270538, -4.429666970165102136, -8.283357778048662468 ) ) ;
#7666=DIRECTION ( 'NONE',  ( -1.000000000000000000, 0.000000000000000000, 0.000000000000000000 ) ) ;
#7669=CARTESIAN_POINT ( 'NONE',  ( 26.01652455409633902, -4.902371455920928156, -5.783357778048663356 ) ) ;
#7673=DIRECTION ( 'NONE',  ( -0.6000000000000001998, -0.7999999999999999334, 0.000000000000000000 ) ) ;
#7675=ORIENTED_EDGE ( 'NONE', *, *, #640, .F. ) ;
#7684=CARTESIAN_POINT ( 'NONE',  ( 8.632250723006720250, -18.84644399697197770, -13.00000000000000178 ) ) ;
#7687=FACE_OUTER_BOUND ( 'NONE', #8303, .T. ) ;
#7692=CARTESIAN_POINT ( 'NONE',  ( 25.96530230012339757, -2.390463732198628399, -5.113484796970851676 ) ) ;
#7694=VERTEX_POINT ( 'NONE', #8376 ) ;
#7696=VERTEX_POINT ( 'NONE', #5203 ) ;
#7701=CARTESIAN_POINT ( 'NONE',  ( -29.25000000000000000, -16.21813761408365195, -13.37255996287876947 ) ) ;
#7703=DIRECTION ( 'NONE',  ( -0.000000000000000000, -0.000000000000000000, -1.000000000000000000 ) ) ;
#7706=CARTESIAN_POINT ( 'NONE',  ( 26.31321956127059636, -7.341867041618697520, -6.247270588150510839 ) ) ;
#7710=CARTESIAN_POINT ( 'NONE',  ( 33.43363050022580296, -2.127845067243429256, -4.705209693361160461 ) ) ;
#7714=CARTESIAN_POINT ( 'NONE',  ( -13.00000000000000178, 1.592040838891559293E-15, -12.00000000000000000 ) ) ;
#7719=CARTESIAN_POINT ( 'NONE',  ( 32.79901970863393501, -6.593096864778464017, -5.783357778048668685 ) ) ;
#7725=CARTESIAN_POINT ( 'NONE',  ( -2.749999999999988454, -20.49999999999999645, -13.00000000000000355 ) ) ;
#7726=CARTESIAN_POINT ( 'NONE',  ( 31.80137159822941939, -6.386132006154467078, -4.533357778048668685 ) ) ;
#7727=CARTESIAN_POINT ( 'NONE',  ( 26.47269060886452507, -6.728324053342490174, -6.861505862736166250 ) ) ;
#7729=CARTESIAN_POINT ( 'NONE',  ( 31.68992120585416217, -1.700760206360153015, -5.783357778048664244 ) ) ;
#7730=CARTESIAN_POINT ( 'NONE',  ( 11.20128062458870843, 15.41171339406673546, -16.67750984750043486 ) ) ;
#7736=VERTEX_POINT ( 'NONE', #1137 ) ;
#7742=CARTESIAN_POINT ( 'NONE',  ( 3.248936832696172505, -15.16081378324841289, -17.00000000000000000 ) ) ;
#7743=VECTOR ( 'NONE', #665, 1000.000000000000000 ) ;
#7745=CARTESIAN_POINT ( 'NONE',  ( 30.09392748191118017, -6.591845302810410701, -7.033357778048666908 ) ) ;
#7758=CARTESIAN_POINT ( 'NONE',  ( -45.00000000000000711, -19.03270077640482683, -10.53798182577225084 ) ) ;
#7759=CARTESIAN_POINT ( 'NONE',  ( 32.24155699611449677, -1.634298987580965923, -5.783357778048664244 ) ) ;
#7762=ORIENTED_EDGE ( 'NONE', *, *, #5016, .F. ) ;
#7766=ORIENTED_EDGE ( 'NONE', *, *, #10585, .F. ) ;
#7769=CARTESIAN_POINT ( 'NONE',  ( 32.29974222271236073, -2.891426744974864071, -3.627061608673662008 ) ) ;
#7776=CARTESIAN_POINT ( 'NONE',  ( 33.50243880635947846, -1.482387629897225390, -5.783357778048663356 ) ) ;
#7778=CIRCLE ( 'NONE', #17934, 2.000000000000001776 ) ;
#7783=ORIENTED_EDGE ( 'NONE', *, *, #14522, .F. ) ;
#7790=CARTESIAN_POINT ( 'NONE',  ( 29.16815758536418102, -2.004582921727632971, -5.783357778048664244 ) ) ;
#7792=CYLINDRICAL_SURFACE ( 'NONE', #1492, 5.000000000000001776 ) ;
#7796=CARTESIAN_POINT ( 'NONE',  ( -35.77680296528374271, -19.03270077640483038, -0.5379818257722508434 ) ) ;
#7797=CARTESIAN_POINT ( 'NONE',  ( 30.01512236704901682, -6.601339762873093875, -7.033357778048666908 ) ) ;
#7799=CARTESIAN_POINT ( 'NONE',  ( 31.24031073583692475, -4.273008382657478954, -3.627061608673664672 ) ) ;
#7800=EDGE_CURVE ( 'NONE', #6646, #16041, #17478, .T. ) ;
#7805=LINE ( 'NONE', #17354, #13635 ) ;
#7808=CARTESIAN_POINT ( 'NONE',  ( 32.64557936882268052, -2.222789665795767089, -4.705209693361161349 ) ) ;
#7810=AXIS2_PLACEMENT_3D ( 'NONE', #6102, #760, #11631 ) ;
#7813=CARTESIAN_POINT ( 'NONE',  ( 30.98067518586950442, -1.786210345264705790, -5.783357778048658027 ) ) ;
#7817=CARTESIAN_POINT ( 'NONE',  ( 31.27600417729400917, -6.449428405189353342, -7.033357778048666908 ) ) ;
#7820=CARTESIAN_POINT ( 'NONE',  ( 27.49697864365563760, -2.843094376337701679, -6.861505862736159145 ) ) ;
#7826=ORIENTED_EDGE ( 'NONE', *, *, #8540, .T. ) ;
#7836=ORIENTED_EDGE ( 'NONE', *, *, #10260, .T. ) ;
#7838=( BOUNDED_CURVE ( )  B_SPLINE_CURVE ( 2, ( #2886, #2797, #8695, #16765, #4336, #5593, #1540, #9941, #1815 ),
 .UNSPECIFIED., .F., .T. ) 
 B_SPLINE_CURVE_WITH_KNOTS ( ( 3, 2, 2, 2, 3 ),
 ( 0.3653846153846154188, 0.3717948717948718063, 0.3846153846153846367, 0.3974358974358974117, 0.4038461538461538547 ),
 .UNSPECIFIED. ) 
 CURVE ( )  GEOMETRIC_REPRESENTATION_ITEM ( )  RATIONAL_B_SPLINE_CURVE ( ( 0.9330127018922194093, 0.9330127018922196314, 1.000000000000000000, 0.8660254037844387076, 1.000000000000000000, 0.8660254037844387076, 1.000000000000000000, 0.9330127018922190762, 0.9330127018922194093 ) ) 
 REPRESENTATION_ITEM ( '' )  );
#7839=CARTESIAN_POINT ( 'NONE',  ( 28.86683379497783264, -7.466592651343750831, -5.783357778048669573 ) ) ;
#7844=DIRECTION ( 'NONE',  ( -0.000000000000000000, 1.000000000000000000, -0.000000000000000000 ) ) ;
#7846=CIRCLE ( 'NONE', #8711, 2.000000000000001776 ) ;
#7849=CARTESIAN_POINT ( 'NONE',  ( 28.77507474356526984, -18.63405514100518801, -13.50648245236009792 ) ) ;
#7851=AXIS2_PLACEMENT_3D ( 'NONE', #1750, #1383, #9880 ) ;
#7856=ORIENTED_EDGE ( 'NONE', *, *, #15285, .F. ) ;
#7858=DIRECTION ( 'NONE',  ( -0.000000000000000000, -0.000000000000000000, -1.000000000000000000 ) ) ;
#7860=ADVANCED_FACE ( 'NONE', ( #12552 ), #15734, .F. ) ;
#7862=CARTESIAN_POINT ( 'NONE',  ( 32.95662993491455950, -6.574107945067995118, -5.783357778048669573 ) ) ;
#7865=CARTESIAN_POINT ( 'NONE',  ( 28.44643833274707845, -2.428894455266221275, -7.033357778048658027 ) ) ;
#7866=DIRECTION ( 'NONE',  ( 0.7999999999999999334, 0.6000000000000001998, 0.000000000000000000 ) ) ;
#7867=CARTESIAN_POINT ( 'NONE',  ( 30.10960860451258370, -6.927314653643411368, -6.453230759126470595 ) ) ;
#7870=CARTESIAN_POINT ( 'NONE',  ( 27.50829672905005907, -3.268828784122926212, -3.283357778048662023 ) ) ;
#7871=CARTESIAN_POINT ( 'NONE',  ( 26.75784435724945709, -6.993777436889428323, -4.533357778048668685 ) ) ;
#7875=AXIS2_PLACEMENT_3D ( 'NONE', #9446, #12350, #2484 ) ;
#7885=VECTOR ( 'NONE', #16755, 1000.000000000000227 ) ;
#7886=CARTESIAN_POINT ( 'NONE',  ( 28.55903157092087952, -3.142235986053133256, -8.283357778048660691 ) ) ;
#7888=DIRECTION ( 'NONE',  ( 0.000000000000000000, 0.000000000000000000, -1.000000000000000000 ) ) ;
#7892=CARTESIAN_POINT ( 'NONE',  ( 30.78487334700428590, -1.819997462563214263, -5.783357778048658027 ) ) ;
#7896=ADVANCED_FACE ( 'NONE', ( #11158 ), #1592, .T. ) ;
#7901=CARTESIAN_POINT ( 'NONE',  ( 29.38830135902312080, -2.615227339812091767, -6.861505862736159145 ) ) ;
#7902=EDGE_CURVE ( 'NONE', #17331, #5257, #3308, .T. ) ;
#7904=CARTESIAN_POINT ( 'NONE',  ( 30.96820195323705605, -2.125071739898741097, -7.033357778048658027 ) ) ;
#7905=CARTESIAN_POINT ( 'NONE',  ( 27.90727577511918867, -2.156494279411373061, -5.783357778048670461 ) ) ;
#7907=CARTESIAN_POINT ( 'NONE',  ( 33.20111501597313719, -6.944397359513344803, -5.783357778048669573 ) ) ;
#7908=CARTESIAN_POINT ( 'NONE',  ( 32.54503264317084188, -5.369756224683081669, -3.627061608673667781 ) ) ;
#7910=CARTESIAN_POINT ( 'NONE',  ( 31.92138306490751987, -2.737139032229836566, -3.283357778048662023 ) ) ;
#7911=CARTESIAN_POINT ( 'NONE',  ( 15.39462056267347734, 12.71537873815137232, -16.22282132715419678 ) ) ;
#7915=EDGE_CURVE ( 'NONE', #15856, #12531, #5736, .T. ) ;
#7917=VERTEX_POINT ( 'NONE', #3483 ) ;
#7918=CIRCLE ( 'NONE', #14872, 13.00000000000000178 ) ;
#7919=ORIENTED_EDGE ( 'NONE', *, *, #4365, .T. ) ;
#7921=CARTESIAN_POINT ( 'NONE',  ( -29.25000000000000000, -15.80023397548365871, -13.37255996287876592 ) ) ;
#7923=ORIENTED_EDGE ( 'NONE', *, *, #13451, .T. ) ;
#7928=CARTESIAN_POINT ( 'NONE',  ( 32.67619606237177265, -1.592130426037604352, -5.783357778048658915 ) ) ;
#7930=ORIENTED_EDGE ( 'NONE', *, *, #1916, .T. ) ;
#7931=CARTESIAN_POINT ( 'NONE',  ( 33.40754056521197413, -5.892811586081919906, -6.861505862736166250 ) ) ;
#7932=CARTESIAN_POINT ( 'NONE',  ( 0.000000000000000000, 0.000000000000000000, -8.700000000000001066 ) ) ;
#7933=CYLINDRICAL_SURFACE ( 'NONE', #1663, 2.499999999999999112 ) ;
#7939=ORIENTED_EDGE ( 'NONE', *, *, #2831, .T. ) ;
#7941=LINE ( 'NONE', #9459, #5792 ) ;
#7942=DIRECTION ( 'NONE',  ( -1.000000000000000000, 0.000000000000000000, 0.000000000000000000 ) ) ;
#7948=( BOUNDED_CURVE ( )  B_SPLINE_CURVE ( 2, ( #12595, #2995, #15499, #5686, #11201, #13861, #6977, #3080, #1448 ),
 .UNSPECIFIED., .F., .T. ) 
 B_SPLINE_CURVE_WITH_KNOTS ( ( 3, 2, 2, 2, 3 ),
 ( 0.5961538461538461453, 0.6025641025641025328, 0.6153846153846154188, 0.6282051282051281937, 0.6346153846153846922 ),
 .UNSPECIFIED. ) 
 CURVE ( )  GEOMETRIC_REPRESENTATION_ITEM ( )  RATIONAL_B_SPLINE_CURVE ( ( 0.9330127018922194093, 0.9330127018922194093, 1.000000000000000000, 0.8660254037844387076, 1.000000000000000000, 0.8660254037844387076, 1.000000000000000000, 0.9330127018922187432, 0.9330127018922192983 ) ) 
 REPRESENTATION_ITEM ( '' )  );
#7950=CARTESIAN_POINT ( 'NONE',  ( 28.71854711534694715, -4.576831098024959132, -3.627061608673664672 ) ) ;
#7954=ORIENTED_EDGE ( 'NONE', *, *, #17702, .F. ) ;
#7955=CARTESIAN_POINT ( 'NONE',  ( -45.50000000000000000, -16.03270077640482683, -8.287981825772241962 ) ) ;
#7957=CARTESIAN_POINT ( 'NONE',  ( 32.43181250335191379, -6.310176327312596811, -4.533357778048668685 ) ) ;
#7967=VERTEX_POINT ( 'NONE', #6288 ) ;
#7972=CARTESIAN_POINT ( 'NONE',  ( 28.19013153391124860, -7.158573733970061248, -5.783357778048657138 ) ) ;
#7976=CARTESIAN_POINT ( 'NONE',  ( 29.98133424373737199, -5.878503772023492502, -8.283357778048664244 ) ) ;
#7977=CARTESIAN_POINT ( 'NONE',  ( 32.81641299864316608, -4.083119185552795294, -7.939653947423662039 ) ) ;
#7986=CARTESIAN_POINT ( 'NONE',  ( 29.39282811755836988, -5.749534618892433002, -3.627061608673667781 ) ) ;
#7989=CARTESIAN_POINT ( 'NONE',  ( 33.48062616923409962, 0.02583177435455490112, -5.783357778048662468 ) ) ;
#7990=DIRECTION ( 'NONE',  ( -0.000000000000000000, -0.000000000000000000, -1.000000000000000000 ) ) ;
#7991=EDGE_CURVE ( 'NONE', #13453, #10591, #613, .T. ) ;
#7992=CARTESIAN_POINT ( 'NONE',  ( 31.90644508241650357, -6.373472726347483963, -7.033357778048666908 ) ) ;
#7995=CARTESIAN_POINT ( 'NONE',  ( 31.78252145740879797, -2.026962321187214311, -4.533357778048659803 ) ) ;
#7998=ORIENTED_EDGE ( 'NONE', *, *, #1585, .F. ) ;
#8004=CARTESIAN_POINT ( 'NONE',  ( 25.71748644841968456, -2.420320648352051851, -5.783357778048663356 ) ) ;
#8008=CARTESIAN_POINT ( 'NONE',  ( 26.90793483298706690, -6.248787706170159773, -8.283357778048662468 ) ) ;
#8019=ORIENTED_EDGE ( 'NONE', *, *, #16397, .T. ) ;
#8021=VERTEX_POINT ( 'NONE', #2518 ) ;
#8024=EDGE_LOOP ( 'NONE', ( #2455, #3053 ) ) ;
#8025=DIRECTION ( 'NONE',  ( 0.9928203230275511881, 0.1196152422706614482, 0.000000000000000000 ) ) ;
#8026=CARTESIAN_POINT ( 'NONE',  ( 29.02054416436834217, -2.659534819136519790, -4.705209693361160461 ) ) ;
#8034=AXIS2_PLACEMENT_3D ( 'NONE', #15528, #17186, #573 ) ;
#8056=CYLINDRICAL_SURFACE ( 'NONE', #2699, 25.00000000000000000 ) ;
#8058=AXIS2_PLACEMENT_3D ( 'NONE', #8812, #646, #17450 ) ;
#8059=CARTESIAN_POINT ( 'NONE',  ( 32.93470988637010066, -5.949778345213319497, -6.861505862736167138 ) ) ;
#8064=CARTESIAN_POINT ( 'NONE',  ( 3.538288549924106796, -15.34800872113743431, -16.99955934415557479 ) ) ;
#8066=VERTEX_POINT ( 'NONE', #1423 ) ;
#8069=CARTESIAN_POINT ( 'NONE',  ( 28.12741954877813555, -2.767138697495831856, -6.861505862736159145 ) ) ;
#8074=VECTOR ( 'NONE', #5915, 1000.000000000000227 ) ;
#8076=DIRECTION ( 'NONE',  ( 0.6000000000000000888, -0.7999999999999999334, 0.000000000000000000 ) ) ;
#8077=CARTESIAN_POINT ( 'NONE',  ( 31.43732351782677625, -4.249272233123119413, -3.283357778048664688 ) ) ;
#8088=AXIS2_PLACEMENT_3D ( 'NONE', #70, #5582, #9738 ) ;
#8090=DIRECTION ( 'NONE',  ( -0.000000000000000000, -0.000000000000000000, -1.000000000000000000 ) ) ;
#8091=CARTESIAN_POINT ( 'NONE',  ( -28.60529878918911706, -13.42304697295875648, -13.55371198823188017 ) ) ;
#8092=ORIENTED_EDGE ( 'NONE', *, *, #15855, .F. ) ;
#8096=CARTESIAN_POINT ( 'NONE',  ( 29.14753769709988518, -3.271205139184214072, -3.627061608673662008 ) ) ;
#8099=CARTESIAN_POINT ( 'NONE',  ( 26.06734695949040059, -6.350061944625998933, -3.283357778048667797 ) ) ;
#8103=CARTESIAN_POINT ( 'NONE',  ( 29.20951391065003122, -17.04067956308641030, -13.38411038749911697 ) ) ;
#8116=LINE ( 'NONE', #6665, #7032 ) ;
#8117=VECTOR ( 'NONE', #1131, 1000.000000000000227 ) ;
#8119=CARTESIAN_POINT ( 'NONE',  ( 30.41294626588012306, -6.253601060580800564, -6.861505862736167138 ) ) ;
#8120=DIRECTION ( 'NONE',  ( -0.5661261679878573094, 0.8243186046180107640, 0.000000000000000000 ) ) ;
#8126=CARTESIAN_POINT ( 'NONE',  ( 28.16197717867739314, -7.161965777771100328, -5.113484796970856117 ) ) ;
#8130=ADVANCED_FACE ( 'NONE', ( #6774 ), #15114, .F. ) ;
#8132=EDGE_LOOP ( 'NONE', ( #12165, #8733 ) ) ;
#8135=ORIENTED_EDGE ( 'NONE', *, *, #12646, .T. ) ;
#8142=CIRCLE ( 'NONE', #7851, 2.749999999999991118 ) ;
#8144=CARTESIAN_POINT ( 'NONE',  ( -1.917618200156724081E-28, -7.000000000000001776, 0.000000000000000000 ) ) ;
#8145=DIRECTION ( 'NONE',  ( 0.000000000000000000, 0.000000000000000000, -1.000000000000000000 ) ) ;
#8148=CARTESIAN_POINT ( 'NONE',  ( 25.76366024945007638, -10.60870341083598056, -14.29366788170017699 ) ) ;
#8149=VECTOR ( 'NONE', #16966, 1000.000000000000114 ) ;
#8152=AXIS2_PLACEMENT_3D ( 'NONE', #8177, #10953, #13709 ) ;
#8153=CARTESIAN_POINT ( 'NONE',  ( 30.93831368681553684, -6.190304661545915188, -4.705209693361169343 ) ) ;
#8156=FACE_OUTER_BOUND ( 'NONE', #1773, .T. ) ;
#8158=CARTESIAN_POINT ( 'NONE',  ( 31.75254397038802878, -4.211294393702175398, -8.283357778048662468 ) ) ;
#8163=CIRCLE ( 'NONE', #354, 5.500000000000000888 ) ;
#8164=CARTESIAN_POINT ( 'NONE',  ( 27.61527553138257574, -4.709753535998224550, -7.939653947423662039 ) ) ;
#8170=DIRECTION ( 'NONE',  ( 0.9928203230275511881, 0.1196152422706614760, 0.000000000000000000 ) ) ;
#8172=DIRECTION ( 'NONE',  ( 0.000000000000000000, -0.000000000000000000, 1.000000000000000000 ) ) ;
#8173=CARTESIAN_POINT ( 'NONE',  ( 29.74110826630370497, -2.999819088432076786, -8.283357778048658915 ) ) ;
#8177=CARTESIAN_POINT ( 'NONE',  ( 0.000000000000000000, 0.000000000000000000, -12.00000000000000000 ) ) ;
#8178=CYLINDRICAL_SURFACE ( 'NONE', #16156, 2.499999999999999112 ) ;
#8193=CARTESIAN_POINT ( 'NONE',  ( 29.02054416436834217, -2.659534819136519790, -4.705209693361160461 ) ) ;
#8195=CARTESIAN_POINT ( 'NONE',  ( 33.27602027394517847, -2.146833986953896822, -4.705209693361161349 ) ) ;
#8196=CARTESIAN_POINT ( 'NONE',  ( 45.50000000000000000, -16.03270077640482683, -2.787981825772258837 ) ) ;
#8197=FACE_OUTER_BOUND ( 'NONE', #6426, .T. ) ;
#8200=CARTESIAN_POINT ( 'NONE',  ( 18.06124445020232727, -20.07065898529088344, -15.83842874644866505 ) ) ;
#8201=AXIS2_PLACEMENT_3D ( 'NONE', #2714, #17803, #13681 ) ;
#8205=VERTEX_POINT ( 'NONE', #2967 ) ;
#8206=CARTESIAN_POINT ( 'NONE',  ( 32.63137222500256485, -6.623491938275930302, -6.453230759126470595 ) ) ;
#8210=CARTESIAN_POINT ( 'NONE',  ( 33.95908713831673964, -3.945449517755637014, -5.783357778048663356 ) ) ;
#8211=CARTESIAN_POINT ( 'NONE',  ( 30.40841950734487753, -3.119293781500474427, -3.627061608673662008 ) ) ;
#8213=CARTESIAN_POINT ( 'NONE',  ( 25.11802603177690330, -16.03270077640482683, -0.5379818257722508434 ) ) ;
#8218=PLANE ( 'NONE',  #2399 ) ;
#8225=EDGE_LOOP ( 'NONE', ( #8739, #4884, #17427, #11989, #15859 ) ) ;
#8230=DIRECTION ( 'NONE',  ( -1.000000000000000000, 0.000000000000000000, -0.000000000000000000 ) ) ;
#8231=CARTESIAN_POINT ( 'NONE',  ( -25.11802603177690330, -19.03270077640482683, -10.53798182577225084 ) ) ;
#8239=CARTESIAN_POINT ( 'NONE',  ( 29.15206445563513071, -6.405512418264540209, -6.861505862736167138 ) ) ;
#8243=CARTESIAN_POINT ( 'NONE',  ( -7.499998387031003411, -20.49508120620799900, -6.000000000000000000 ) ) ;
#8248=CARTESIAN_POINT ( 'NONE',  ( 27.93049598394382116, -4.671775696577297410, -3.627061608673664672 ) ) ;
#8249=CARTESIAN_POINT ( 'NONE',  ( 8.632250723006720250, -18.84644399697197770, -13.00000000000000178 ) ) ;
#8255=EDGE_CURVE ( 'NONE', #15783, #7031, #1242, .T. ) ;
#8256=CARTESIAN_POINT ( 'NONE',  ( 27.15176839919044482, -1.857969822100365098, -5.783357778048658027 ) ) ;
#8267=DIRECTION ( 'NONE',  ( 1.000000000000000000, 0.000000000000000000, 0.000000000000000000 ) ) ;
#8268=CARTESIAN_POINT ( 'NONE',  ( -29.25000000000000000, -16.21813761408365195, -13.37255996287876947 ) ) ;
#8270=CARTESIAN_POINT ( 'NONE',  ( 30.17635249042624679, -2.520282741259753045, -6.861505862736158257 ) ) ;
#8273=CARTESIAN_POINT ( 'NONE',  ( 32.54503264317084188, -5.369756224683081669, -3.627061608673667781 ) ) ;
#8280=( BOUNDED_CURVE ( )  B_SPLINE_CURVE ( 2, ( #22, #16524, #9783, #3017, #7102, #12526, #13986, #8352, #16800 ),
 .UNSPECIFIED., .F., .T. ) 
 B_SPLINE_CURVE_WITH_KNOTS ( ( 3, 2, 2, 2, 3 ),
 ( 0.4423076923076923461, 0.4487179487179487336, 0.4615384615384615641, 0.4743589743589743390, 0.4807692307692307820 ),
 .UNSPECIFIED. ) 
 CURVE ( )  GEOMETRIC_REPRESENTATION_ITEM ( )  RATIONAL_B_SPLINE_CURVE ( ( 0.9330127018922194093, 0.9330127018922196314, 1.000000000000000000, 0.8660254037844387076, 1.000000000000000000, 0.8660254037844387076, 1.000000000000000000, 0.9330127018922190762, 0.9330127018922194093 ) ) 
 REPRESENTATION_ITEM ( '' )  );
#8286=VERTEX_POINT ( 'NONE', #343 ) ;
#8287=FACE_OUTER_BOUND ( 'NONE', #10153, .T. ) ;
#8290=CARTESIAN_POINT ( 'NONE',  ( 31.03886041246737548, -3.043338102658604161, -3.627061608673662008 ) ) ;
#8293=CARTESIAN_POINT ( 'NONE',  ( 30.45035428628836627, -2.914368949527523789, -8.283357778048660691 ) ) ;
#8296=CARTESIAN_POINT ( 'NONE',  ( 30.37838863598085837, -1.858773980305536089, -5.113484796970855228 ) ) ;
#8298=LINE ( 'NONE', #13827, #6723 ) ;
#8300=ADVANCED_FACE ( 'NONE', ( #16748 ), #10014, .F. ) ;
#8303=EDGE_LOOP ( 'NONE', ( #10942, #16420, #11233, #11376 ) ) ;
#8304=ADVANCED_FACE ( 'NONE', ( #5940 ), #12569, .T. ) ;
#8310=DIRECTION ( 'NONE',  ( -1.000000000000000000, 0.000000000000000000, 0.000000000000000000 ) ) ;
#8317=EDGE_CURVE ( 'NONE', #3497, #15348, #7025, .T. ) ;
#8318=CARTESIAN_POINT ( 'NONE',  ( 25.57853536445108489, -10.52124088318384310, -14.33864855032055985 ) ) ;
#8320=CARTESIAN_POINT ( 'NONE',  ( 29.17398450417959310, -7.029842018119214941, -5.783357778048669573 ) ) ;
#8334=DIRECTION ( 'NONE',  ( 0.000000000000000000, 0.000000000000000000, 1.000000000000000000 ) ) ;
#8337=CARTESIAN_POINT ( 'NONE',  ( 26.82912971812490355, -6.258282166232842947, -8.283357778048662468 ) ) ;
#8338=VECTOR ( 'NONE', #2312, 1000.000000000000000 ) ;
#8340=CARTESIAN_POINT ( 'NONE',  ( 30.90769699326644826, -6.820963901304073929, -5.783357778048668685 ) ) ;
#8342=CARTESIAN_POINT ( 'NONE',  ( 27.87912141988533676, -2.159886323212414361, -6.453230759126469707 ) ) ;
#8343=FACE_BOUND ( 'NONE', #14179, .T. ) ;
#8351=DIRECTION ( 'NONE',  ( 0.9928203230275510771, 0.1196152422706614621, -0.000000000000000000 ) ) ;
#8352=CARTESIAN_POINT ( 'NONE',  ( 29.74794773085836397, -1.934729659147405689, -5.113484796970855228 ) ) ;
#8354=ORIENTED_EDGE ( 'NONE', *, *, #10602, .F. ) ;
#8355=CARTESIAN_POINT ( 'NONE',  ( -16.79182286896198306, -15.38653328895459893, -16.02976683711036898 ) ) ;
#8357=CARTESIAN_POINT ( 'NONE',  ( 29.54591158530375239, -2.596238420101622868, -6.861505862736158257 ) ) ;
#8359=VECTOR ( 'NONE', #7844, 1000.000000000000000 ) ;
#8360=CARTESIAN_POINT ( 'NONE',  ( 28.98992747081925359, -3.290194058894681639, -3.627061608673662896 ) ) ;
#8366=CARTESIAN_POINT ( 'NONE',  ( 20.84394630543432569, -22.08803114836474890, -15.35658910651175013 ) ) ;
#8368=AXIS2_PLACEMENT_3D ( 'NONE', #9891, #11333, #7112 ) ;
#8375=VERTEX_POINT ( 'NONE', #15838 ) ;
#8376=CARTESIAN_POINT ( 'NONE',  ( 20.00000000000000000, 7.999999999999996447, -15.51150668642334374 ) ) ;
#8378=CARTESIAN_POINT ( 'NONE',  ( 33.69269431359690969, -6.158264969628857166, -4.533357778048668685 ) ) ;
#8379=CARTESIAN_POINT ( 'NONE',  ( 26.19678349485696955, -4.880653813392439311, -3.627061608673664672 ) ) ;
#8384=AXIS2_PLACEMENT_3D ( 'NONE', #2347, #978, #16215 ) ;
#8400=ORIENTED_EDGE ( 'NONE', *, *, #16124, .F. ) ;
#8403=DIRECTION ( 'NONE',  ( 0.9928203230275510771, 0.1196152422706614621, -0.000000000000000000 ) ) ;
#8407=DIRECTION ( 'NONE',  ( -0.000000000000000000, 1.000000000000000000, -0.000000000000000000 ) ) ;
#8408=CARTESIAN_POINT ( 'NONE',  ( 18.46842688268906230, -11.90892979872008084, -15.77307170257308933 ) ) ;
#8409=FACE_OUTER_BOUND ( 'NONE', #6173, .T. ) ;
#8411=( BOUNDED_CURVE ( )  B_SPLINE_CURVE ( 2, ( #5762, #15120, #17959, #16574, #12578 ),
 .UNSPECIFIED., .F., .T. ) 
 B_SPLINE_CURVE_WITH_KNOTS ( ( 3, 2, 3 ),
 ( 0.000000000000000000, 0.01282051282051282007, 0.01923076923076924918 ),
 .UNSPECIFIED. ) 
 CURVE ( )  GEOMETRIC_REPRESENTATION_ITEM ( )  RATIONAL_B_SPLINE_CURVE ( ( 1.000000000000000000, 0.8660254037844387076, 1.000000000000000000, 0.9330127018922191873, 0.9330127018922194093 ) ) 
 REPRESENTATION_ITEM ( '' )  );
#8415=ORIENTED_EDGE ( 'NONE', *, *, #17570, .T. ) ;
#8421=CARTESIAN_POINT ( 'NONE',  ( 26.03917326857634151, -4.899642733102906433, -3.627061608673664672 ) ) ;
#8423=CARTESIAN_POINT ( 'NONE',  ( -4.914599809708808387, 17.56967244544484075, -17.00000000000000711 ) ) ;
#8426=LINE ( 'NONE', #4525, #4087 ) ;
#8428=AXIS2_PLACEMENT_3D ( 'NONE', #1089, #6613, #14956 ) ;
#8430=CARTESIAN_POINT ( 'NONE',  ( 28.01872616749444944, -6.841866079205687790, -4.533357778048668685 ) ) ;
#8431=AXIS2_PLACEMENT_3D ( 'NONE', #14881, #5519, #9592 ) ;
#8432=ADVANCED_FACE ( 'NONE', ( #4940 ), #10288, .F. ) ;
#8433=CARTESIAN_POINT ( 'NONE',  ( 30.25533603959949502, -6.272589980291270351, -6.861505862736166250 ) ) ;
#8444=ORIENTED_EDGE ( 'NONE', *, *, #3385, .F. ) ;
#8445=ORIENTED_EDGE ( 'NONE', *, *, #5534, .F. ) ;
#8449=AXIS2_PLACEMENT_3D ( 'NONE', #15991, #6460, #5253 ) ;
#8451=CARTESIAN_POINT ( 'NONE',  ( -27.17934203385504333, -30.00000000000000355, 0.000000000000000000 ) ) ;
#8452=ORIENTED_EDGE ( 'NONE', *, *, #11091, .T. ) ;
#8453=CARTESIAN_POINT ( 'NONE',  ( 29.76058531221316272, -5.705227139567997874, -7.939653947423662927 ) ) ;
#8454=CARTESIAN_POINT ( 'NONE',  ( -20.00000000000000355, 7.999999999999996447, -6.000000000000000000 ) ) ;
#8458=CARTESIAN_POINT ( 'NONE',  ( 29.64681518302145591, -6.972875258987813574, -5.783357778048668685 ) ) ;
#8462=ORIENTED_EDGE ( 'NONE', *, *, #14891, .F. ) ;
#8476=ORIENTED_EDGE ( 'NONE', *, *, #4941, .T. ) ;
#8478=CARTESIAN_POINT ( 'NONE',  ( 27.00222791626931595, -2.275731535614434531, -5.783357778048658027 ) ) ;
#8483=CARTESIAN_POINT ( 'NONE',  ( 25.71748644841968456, -2.420320648352051851, -5.783357778048663356 ) ) ;
#8489=EDGE_CURVE ( 'NONE', #17637, #16432, #7592, .T. ) ;
#8490=ORIENTED_EDGE ( 'NONE', *, *, #9289, .T. ) ;
#8493=ORIENTED_EDGE ( 'NONE', *, *, #11024, .F. ) ;
#8495=CARTESIAN_POINT ( 'NONE',  ( 31.05948030073166066, -1.776715885202022394, -5.783357778048661579 ) ) ;
#8496=CARTESIAN_POINT ( 'NONE',  ( -16.75000000000000000, -16.21813761408365195, -16.03574476417183448 ) ) ;
#8498=CARTESIAN_POINT ( 'NONE',  ( 33.23365877489121090, -6.550928303235100891, -5.783357778048663356 ) ) ;
#8500=CARTESIAN_POINT ( 'NONE',  ( -20.00000000000000000, 7.999999999999996447, -15.51150668642334374 ) ) ;
#8514=ORIENTED_EDGE ( 'NONE', *, *, #10326, .T. ) ;
#8523=LINE ( 'NONE', #16970, #13665 ) ;
#8525=CARTESIAN_POINT ( 'NONE',  ( 26.58890374069123652, -3.379597482641427231, -8.283357778048658915 ) ) ;
#8527=EDGE_CURVE ( 'NONE', #947, #15308, #14555, .T. ) ;
#8528=CARTESIAN_POINT ( 'NONE',  ( 30.67110321781257909, -3.087645581983020637, -7.939653947423660263 ) ) ;
#8529=DIRECTION ( 'NONE',  ( 1.000000000000000000, 0.000000000000000000, -0.000000000000000000 ) ) ;
#8530=CARTESIAN_POINT ( 'NONE',  ( 26.01652455409633902, -4.902371455920928156, -5.783357778048663356 ) ) ;
#8540=EDGE_CURVE ( 'NONE', #9208, #1330, #16403, .T. ) ;
#8541=DIRECTION ( 'NONE',  ( 0.000000000000000000, 0.000000000000000000, 1.000000000000000000 ) ) ;
#8543=CARTESIAN_POINT ( 'NONE',  ( 27.78610916120306129, -6.570083055755264745, -4.705209693361169343 ) ) ;
#8545=ADVANCED_FACE ( 'NONE', ( #350 ), #5859, .F. ) ;
#8546=CARTESIAN_POINT ( 'NONE',  ( 31.53813789838894621, -6.745008222462202774, -5.783357778048668685 ) ) ;
#8548=FACE_OUTER_BOUND ( 'NONE', #3742, .T. ) ;
#8549=CARTESIAN_POINT ( 'NONE',  ( 33.60446413004628141, -3.988174587000466342, -3.627061608673664672 ) ) ;
#8551=CARTESIAN_POINT ( 'NONE',  ( 16.79145860028663151, -17.04903085677362640, -16.02982020200856184 ) ) ;
#8554=EDGE_CURVE ( 'NONE', #14154, #16037, #15851, .T. ) ;
#8561=CARTESIAN_POINT ( 'NONE',  ( -45.50000000000000000, -16.03270077640482683, -5.537981825772250843 ) ) ;
#8562=VERTEX_POINT ( 'NONE', #14034 ) ;
#8564=CARTESIAN_POINT ( 'NONE',  ( 33.64386668575551198, -3.983427357176565486, -8.283357778048662468 ) ) ;
#8565=CARTESIAN_POINT ( 'NONE',  ( 33.40745134805642635, -4.011910736534825439, -3.283357778048664688 ) ) ;
#8567=CYLINDRICAL_SURFACE ( 'NONE', #11548, 5.500000000000000888 ) ;
#8570=CARTESIAN_POINT ( 'NONE',  ( 26.90109536843240789, -7.313877135454839973, -5.113484796970856117 ) ) ;
#8572=ORIENTED_EDGE ( 'NONE', *, *, #14, .T. ) ;
#8579=ORIENTED_EDGE ( 'NONE', *, *, #9764, .F. ) ;
#8580=PLANE ( 'NONE',  #16353 ) ;
#8583=CARTESIAN_POINT ( 'NONE',  ( 32.93832978346670615, -1.887710243310447567, -7.033357778048658027 ) ) ;
#8592=LINE ( 'NONE', #14224, #261 ) ;
#8594=ORIENTED_EDGE ( 'NONE', *, *, #1804, .F. ) ;
#8596=CARTESIAN_POINT ( 'NONE',  ( 31.59864285835955400, -2.049116061056871274, -7.033357778048658027 ) ) ;
#8598=ORIENTED_EDGE ( 'NONE', *, *, #12117, .T. ) ;
#8602=CYLINDRICAL_SURFACE ( 'NONE', #17655, 6.249999999999998224 ) ;
#8604=CARTESIAN_POINT ( 'NONE',  ( -17.24286622940504188, 11.12094428624988218, -15.96573730347181019 ) ) ;
#8605=CARTESIAN_POINT ( 'NONE',  ( -20.00000000000000000, 7.999999999999996447, -6.000000000000000000 ) ) ;
#8607=CARTESIAN_POINT ( 'NONE',  ( 31.74131510559286085, -5.666460835049167422, -3.283357778048667797 ) ) ;
#8611=CARTESIAN_POINT ( 'NONE',  ( 26.18945719470476163, -6.341381504099093291, -7.820351782355674963 ) ) ;
#8613=CARTESIAN_POINT ( 'NONE',  ( 28.76238721243587193, -5.825490297734302381, -3.627061608673667781 ) ) ;
#8615=LINE ( 'NONE', #7955, #12513 ) ;
#8617=EDGE_LOOP ( 'NONE', ( #728, #2242, #5049, #17411, #3201 ) ) ;
#8623=ORIENTED_EDGE ( 'NONE', *, *, #2701, .T. ) ;
#8624=AXIS2_PLACEMENT_3D ( 'NONE', #6510, #7367, #11935 ) ;
#8626=CARTESIAN_POINT ( 'NONE',  ( 35.19141017012124451, -14.17387298022714326, -11.46934516270796323 ) ) ;
#8627=EDGE_CURVE ( 'NONE', #12549, #5172, #17140, .T. ) ;
#8629=CARTESIAN_POINT ( 'NONE',  ( -22.21636613273916794, -10.00424398458219066, -15.08813622000165466 ) ) ;
#8630=ORIENTED_EDGE ( 'NONE', *, *, #1079, .T. ) ;
#8634=EDGE_CURVE ( 'NONE', #29, #6646, #5039, .T. ) ;
#8635=CARTESIAN_POINT ( 'NONE',  ( 31.38469755857769528, -2.374701023479507178, -4.705209693361161349 ) ) ;
#8641=EDGE_CURVE ( 'NONE', #15612, #17048, #14593, .T. ) ;
#8659=CARTESIAN_POINT ( 'NONE',  ( 28.54354359905709870, -7.105797696961086096, -5.783357778048669573 ) ) ;
#8660=CARTESIAN_POINT ( 'NONE',  ( 33.21234388421201089, -5.489230917751459771, -8.283357778048662468 ) ) ;
#8663=PLANE ( 'NONE',  #13303 ) ;
#8664=CARTESIAN_POINT ( 'NONE',  ( 28.71854711534694715, -4.576831098024959132, -3.627061608673664672 ) ) ;
#8668=CARTESIAN_POINT ( 'NONE',  ( 30.98067518586950442, -1.786210345264705790, -5.783357778048658027 ) ) ;
#8671=VERTEX_POINT ( 'NONE', #3509 ) ;
#8672=VECTOR ( 'NONE', #6801, 1000.000000000000000 ) ;
#8674=VERTEX_POINT ( 'NONE', #703 ) ;
#8679=ADVANCED_FACE ( 'NONE', ( #17600 ), #16300, .F. ) ;
#8683=LINE ( 'NONE', #11379, #16860 ) ;
#8689=CARTESIAN_POINT ( 'NONE',  ( -15.92260893619738837, -28.39189527176317540, 0.000000000000000000 ) ) ;
#8691=VERTEX_POINT ( 'NONE', #2007 ) ;
#8693=EDGE_CURVE ( 'NONE', #1377, #2104, #9957, .T. ) ;
#8695=CARTESIAN_POINT ( 'NONE',  ( 30.61929490284659394, -6.528548903775525325, -4.533357778048668685 ) ) ;
#8704=CARTESIAN_POINT ( 'NONE',  ( -23.43613571611706803, -22.46619466838626877, -14.83130101496670861 ) ) ;
#8706=CARTESIAN_POINT ( 'NONE',  ( 31.66176685062031027, -1.704152250161192539, -6.453230759126468818 ) ) ;
#8711=AXIS2_PLACEMENT_3D ( 'NONE', #10621, #3488, #7666 ) ;
#8713=CARTESIAN_POINT ( 'NONE',  ( 31.49429780130001433, -5.496349022752856861, -7.939653947423664704 ) ) ;
#8714=PLANE ( 'NONE',  #3203 ) ;
#8717=CARTESIAN_POINT ( 'NONE',  ( -7.499998387031003411, -20.49508120620799900, -6.000000000000000000 ) ) ;
#8729=AXIS2_PLACEMENT_3D ( 'NONE', #10752, #14947, #4060 ) ;
#8730=CARTESIAN_POINT ( 'NONE',  ( 25.71748644841968456, -2.420320648352051851, -5.783357778048663356 ) ) ;
#8731=CARTESIAN_POINT ( 'NONE',  ( 27.02414796481377124, -2.900061135469103490, -6.861505862736158257 ) ) ;
#8733=ORIENTED_EDGE ( 'NONE', *, *, #7066, .F. ) ;
#8734=CARTESIAN_POINT ( 'NONE',  ( 29.50659824675005893, -4.481886499472614638, -7.939653947423662039 ) ) ;
#8736=CARTESIAN_POINT ( 'NONE',  ( 33.18300801526289234, -6.557030719496743210, -6.453230759126470595 ) ) ;
#8739=ORIENTED_EDGE ( 'NONE', *, *, #16999, .F. ) ;
#8749=LINE ( 'NONE', #411, #8074 ) ;
#8750=AXIS2_PLACEMENT_3D ( 'NONE', #8144, #13674, #9151 ) ;
#8757=CARTESIAN_POINT ( 'NONE',  ( 27.55969062878875064, -7.234529412811931515, -5.783357778048668685 ) ) ;
#8758=AXIS2_PLACEMENT_3D ( 'NONE', #5568, #7318, #12647 ) ;
#8760=CARTESIAN_POINT ( 'NONE',  ( 32.64947922571280259, -7.010858578292532783, -5.783357778048669573 ) ) ;
#8761=DIRECTION ( 'NONE',  ( 0.000000000000000000, 0.000000000000000000, -1.000000000000000000 ) ) ;
#8765=CARTESIAN_POINT ( 'NONE',  ( 25.71748644841968456, -2.420320648352051851, -5.783357778048663356 ) ) ;
#8766=CYLINDRICAL_SURFACE ( 'NONE', #6020, 2.499999999999999112 ) ;
#8771=ORIENTED_EDGE ( 'NONE', *, *, #12351, .F. ) ;
#8773=LINE ( 'NONE', #11557, #15093 ) ;
#8774=CARTESIAN_POINT ( 'NONE',  ( 26.32044349065828115, -7.243571858916999950, -6.694428052743685242 ) ) ;
#8779=CARTESIAN_POINT ( 'NONE',  ( 25.92467471225709374, -2.732717170633701453, -7.033357778048658027 ) ) ;
#8793=ORIENTED_EDGE ( 'NONE', *, *, #2508, .F. ) ;
#8796=FACE_BOUND ( 'NONE', #8024, .T. ) ;
#8799=PLANE ( 'NONE',  #621 ) ;
#8802=CARTESIAN_POINT ( 'NONE',  ( 29.35841309260160159, -6.680460261459264970, -4.533357778048668685 ) ) ;
#8805=CARTESIAN_POINT ( 'NONE',  ( 26.02974819644417792, -2.720057890826728109, -4.533357778048659803 ) ) ;
#8808=CARTESIAN_POINT ( 'NONE',  ( 26.87106449706838873, -6.053357334259913181, -3.627061608673667781 ) ) ;
#8810=CARTESIAN_POINT ( 'NONE',  ( 14.00000000000000178, 1.714505518806294835E-15, -8.700000000000001066 ) ) ;
#8811=CARTESIAN_POINT ( 'NONE',  ( 33.76207435632690590, -3.969185667289998332, -3.627061608673664672 ) ) ;
#8812=CARTESIAN_POINT ( 'NONE',  ( 26.01652455409633902, -4.902371455920928156, -5.783357778048663356 ) ) ;
#8814=DIRECTION ( 'NONE',  ( 1.000000000000000000, 0.000000000000000000, -0.000000000000000000 ) ) ;
#8817=EDGE_LOOP ( 'NONE', ( #8493, #11914 ) ) ;
#8821=CARTESIAN_POINT ( 'NONE',  ( 27.00222791626931240, -2.275731535614434531, -5.783357778048658915 ) ) ;
#8823=ORIENTED_EDGE ( 'NONE', *, *, #13686, .F. ) ;
#8824=CARTESIAN_POINT ( 'NONE',  ( 26.98483462626008134, -4.785709214840094816, -7.939653947423662039 ) ) ;
#8826=CARTESIAN_POINT ( 'NONE',  ( 28.45891156537951971, -2.090033060632186412, -5.783357778048670461 ) ) ;
#8827=PLANE ( 'NONE',  #5420 ) ;
#8831=DIRECTION ( 'NONE',  ( -0.5999999999999999778, -0.7999999999999999334, 0.000000000000000000 ) ) ;
#8835=CARTESIAN_POINT ( 'NONE',  ( 35.74085044863416982, -18.73429073671341172, -11.27079897466147251 ) ) ;
#8836=ORIENTED_EDGE ( 'NONE', *, *, #13511, .T. ) ;
#8837=CARTESIAN_POINT ( 'NONE',  ( 9.099998387031005720, -19.29508120620799971, -16.81964500401478091 ) ) ;
#8840=CARTESIAN_POINT ( 'NONE',  ( 26.87785582392756112, -3.344784462964796035, -3.283357778048662023 ) ) ;
#8841=CARTESIAN_POINT ( 'NONE',  ( 30.03006034954003667, -2.965006068755446478, -3.283357778048662023 ) ) ;
#8850=ORIENTED_EDGE ( 'NONE', *, *, #4828, .F. ) ;
#8855=CARTESIAN_POINT ( 'NONE',  ( 26.01652455409633902, -4.902371455920928156, -5.783357778048663356 ) ) ;
#8858=CARTESIAN_POINT ( 'NONE',  ( 34.43754810739937966, -7.916730809865828888, -5.783357778048663356 ) ) ;
#8859=ORIENTED_EDGE ( 'NONE', *, *, #13855, .T. ) ;
#8862=ORIENTED_EDGE ( 'NONE', *, *, #6551, .T. ) ;
#8864=CARTESIAN_POINT ( 'NONE',  ( 32.70264286945147347, -5.350767304972614546, -3.627061608673668225 ) ) ;
#8868=ADVANCED_FACE ( 'NONE', ( #2194 ), #12136, .T. ) ;
#8873=EDGE_CURVE ( 'NONE', #12535, #8691, #8983, .T. ) ;
#8883=CARTESIAN_POINT ( 'NONE',  ( -27.94765010173961883, -20.05889348609997924, -13.73347386810006832 ) ) ;
#8886=DIRECTION ( 'NONE',  ( 0.000000000000000000, 0.000000000000000000, 1.000000000000000000 ) ) ;
#8887=CARTESIAN_POINT ( 'NONE',  ( 28.63031693179632242, -2.406740715396564756, -4.533357778048659803 ) ) ;
#8892=CARTESIAN_POINT ( 'NONE',  ( 27.51889869220010354, -3.467423976192371082, -7.939653947423660263 ) ) ;
#8901=CARTESIAN_POINT ( 'NONE',  ( 31.27962407439061110, -2.387360303286481855, -6.861505862736159145 ) ) ;
#8902=ORIENTED_EDGE ( 'NONE', *, *, #12443, .F. ) ;
#8904=CARTESIAN_POINT ( 'NONE',  ( 45.00000000000000711, -19.03270077640483038, -5.537981825772250843 ) ) ;
#8907=CARTESIAN_POINT ( 'NONE',  ( 27.45766530510195835, -4.728742455708699666, -3.627061608673664672 ) ) ;
#8908=CARTESIAN_POINT ( 'NONE',  ( 26.19678349485696955, -4.880653813392439311, -3.627061608673664672 ) ) ;
#8910=CARTESIAN_POINT ( 'NONE',  ( 28.38593337277646711, -7.124786616671554107, -5.783357778048668685 ) ) ;
#8913=FACE_OUTER_BOUND ( 'NONE', #17912, .T. ) ;
#8915=EDGE_CURVE ( 'NONE', #10032, #7736, #10220, .T. ) ;
#8918=ORIENTED_EDGE ( 'NONE', *, *, #2209, .F. ) ;
#8922=DIRECTION ( 'NONE',  ( 0.000000000000000000, 0.000000000000000000, 1.000000000000000000 ) ) ;
#8924=FACE_OUTER_BOUND ( 'NONE', #14485, .T. ) ;
#8926=CARTESIAN_POINT ( 'NONE',  ( 29.81991338116587542, -2.990324628369393611, -8.283357778048658915 ) ) ;
#8936=ADVANCED_FACE ( 'NONE', ( #6788 ), #5498, .T. ) ;
#8937=EDGE_LOOP ( 'NONE', ( #16006, #17407, #13381, #17762 ) ) ;
#8945=DIRECTION ( 'NONE',  ( -0.6174492339697512655, -0.7866107318554506067, 0.000000000000000000 ) ) ;
#8949=CARTESIAN_POINT ( 'NONE',  ( 32.93470988637010066, -5.949778345213319497, -6.861505862736167138 ) ) ;
#8953=CYLINDRICAL_SURFACE ( 'NONE', #8963, 2.749999999999992895 ) ;
#8958=EDGE_CURVE ( 'NONE', #10072, #13311, #9355, .T. ) ;
#8963=AXIS2_PLACEMENT_3D ( 'NONE', #6415, #13215, #4951 ) ;
#8967=PLANE ( 'NONE',  #10677 ) ;
#8968=CARTESIAN_POINT ( 'NONE',  ( -16.75000000000000000, -16.21813761408365195, -16.03574476417183448 ) ) ;
#8970=CARTESIAN_POINT ( 'NONE',  ( 32.95080301609915097, -1.548848848676412260, -5.783357778048663356 ) ) ;
#8979=CARTESIAN_POINT ( 'NONE',  ( 27.71165237056504438, -5.952083095804076684, -7.939653947423664704 ) ) ;
#8983=( BOUNDED_CURVE ( )  B_SPLINE_CURVE ( 2, ( #1082, #6342, #3635, #907, #9236, #7976, #7797, #17346, #810 ),
 .UNSPECIFIED., .F., .T. ) 
 B_SPLINE_CURVE_WITH_KNOTS ( ( 3, 2, 2, 2, 3 ),
 ( 0.4807692307692307820, 0.4871794871794871695, 0.5000000000000000000, 0.5128205128205127750, 0.5192307692307692735 ),
 .UNSPECIFIED. ) 
 CURVE ( )  GEOMETRIC_REPRESENTATION_ITEM ( )  RATIONAL_B_SPLINE_CURVE ( ( 0.9330127018922194093, 0.9330127018922196314, 1.000000000000000000, 0.8660254037844387076, 1.000000000000000000, 0.8660254037844387076, 1.000000000000000000, 0.9330127018922187432, 0.9330127018922192983 ) ) 
 REPRESENTATION_ITEM ( '' )  );
#8987=ORIENTED_EDGE ( 'NONE', *, *, #1850, .T. ) ;
#8989=CARTESIAN_POINT ( 'NONE',  ( 29.99682221560115991, -1.914942061115552541, -5.783357778048658915 ) ) ;
#8991=DIRECTION ( 'NONE',  ( 0.000000000000000000, -1.000000000000000000, -0.000000000000000000 ) ) ;
#8993=DIRECTION ( 'NONE',  ( -0.000000000000000000, -0.000000000000000000, -1.000000000000000000 ) ) ;
#8994=AXIS2_PLACEMENT_3D ( 'NONE', #13104, #16016, #681 ) ;
#8997=CARTESIAN_POINT ( 'NONE',  ( 27.02414796481377124, -2.900061135469103490, -6.861505862736158257 ) ) ;
#8999=CARTESIAN_POINT ( 'NONE',  ( 25.62757597683262034, -3.695291012717980994, -7.939653947423660263 ) ) ;
#9000=CARTESIAN_POINT ( 'NONE',  ( 28.13948077428293715, -7.164676150231702678, -6.453230759126474148 ) ) ;
#9003=( BOUNDED_CURVE ( )  B_SPLINE_CURVE ( 2, ( #8757, #9909, #14288, #3310, #12728, #8840, #4660, #1682, #4567 ),
 .UNSPECIFIED., .F., .T. ) 
 B_SPLINE_CURVE_WITH_KNOTS ( ( 3, 2, 2, 2, 3 ),
 ( 0.7500000000000000000, 0.7564102564102563875, 0.7692307692307692735, 0.7820512820512820484, 0.7884615384615384359 ),
 .UNSPECIFIED. ) 
 CURVE ( )  GEOMETRIC_REPRESENTATION_ITEM ( )  RATIONAL_B_SPLINE_CURVE ( ( 0.9330127018922194093, 0.9330127018922194093, 1.000000000000000000, 0.8660254037844387076, 1.000000000000000000, 0.8660254037844387076, 1.000000000000000000, 0.9330127018922194093, 0.9330127018922194093 ) ) 
 REPRESENTATION_ITEM ( '' )  );
#9007=VERTEX_POINT ( 'NONE', #16674 ) ;
#9009=DIRECTION ( 'NONE',  ( 0.000000000000000000, 0.000000000000000000, 1.000000000000000000 ) ) ;
#9011=ORIENTED_EDGE ( 'NONE', *, *, #8554, .T. ) ;
#9013=DIRECTION ( 'NONE',  ( -0.000000000000000000, -1.000000000000000000, -0.000000000000000000 ) ) ;
#9015=CARTESIAN_POINT ( 'NONE',  ( 32.08959525433819238, -2.916745304588811205, -7.939653947423660263 ) ) ;
#9018=CIRCLE ( 'NONE', #1496, 5.500000000000000000 ) ;
#9019=ADVANCED_FACE ( 'NONE', ( #8409 ), #8056, .T. ) ;
#9021=CARTESIAN_POINT ( 'NONE',  ( 28.20260476654369697, -6.819712339336020612, -7.033357778048666908 ) ) ;
#9025=DIRECTION ( 'NONE',  ( 0.1113444980252557837, 0.9937818688019538493, -0.000000000000000000 ) ) ;
#9027=ORIENTED_EDGE ( 'NONE', *, *, #17198, .F. ) ;
#9029=VERTEX_POINT ( 'NONE', #13594 ) ;
#9036=ORIENTED_EDGE ( 'NONE', *, *, #15758, .F. ) ;
#9044=FACE_OUTER_BOUND ( 'NONE', #13038, .T. ) ;
#9047=VECTOR ( 'NONE', #13798, 1000.000000000000227 ) ;
#9053=ORIENTED_EDGE ( 'NONE', *, *, #12117, .F. ) ;
#9058=VERTEX_POINT ( 'NONE', #8689 ) ;
#9060=VECTOR ( 'NONE', #14836, 1000.000000000000227 ) ;
#9061=CARTESIAN_POINT ( 'NONE',  ( -28.29220412912503946, -19.54937045720491184, -13.63977809545137454 ) ) ;
#9064=PLANE ( 'NONE',  #7272 ) ;
#9073=CARTESIAN_POINT ( 'NONE',  ( 26.25801688195511474, -3.619335333876111171, -7.939653947423660263 ) ) ;
#9074=AXIS2_PLACEMENT_3D ( 'NONE', #16413, #16492, #11189 ) ;
#9083=CARTESIAN_POINT ( 'NONE',  ( 32.02836186724004364, -4.178063784105134459, -7.939653947423662039 ) ) ;
#9085=CARTESIAN_POINT ( 'NONE',  ( 29.14000323013032556, -2.007974965528672495, -6.453230759126468818 ) ) ;
#9090=CARTESIAN_POINT ( 'NONE',  ( 32.06776442294927421, -4.173316554281249147, -3.283357778048664688 ) ) ;
#9091=CARTESIAN_POINT ( 'NONE',  ( 28.24571643650507369, -4.633797857156355171, -7.939653947423662039 ) ) ;
#9093=CARTESIAN_POINT ( 'NONE',  ( 32.85952466860454280, -1.897204703373130741, -7.033357778048658027 ) ) ;
#9094=CARTESIAN_POINT ( 'NONE',  ( 4.906836669863238853, 17.52808241874658890, -16.98904569177533119 ) ) ;
#9101=LINE ( 'NONE', #14642, #3473 ) ;
#9107=CARTESIAN_POINT ( 'NONE',  ( 32.28234893270314387, -5.401404424200516807, -7.939653947423662927 ) ) ;
#9111=CARTESIAN_POINT ( 'NONE',  ( 27.26436163736424945, -2.571311352887278190, -7.033357778048658027 ) ) ;
#9114=LINE ( 'NONE', #10459, #4606 ) ;
#9128=CARTESIAN_POINT ( 'NONE',  ( 28.71361296893772774, -7.095504558991913235, -5.113484796970856117 ) ) ;
#9131=CARTESIAN_POINT ( 'NONE',  ( 32.91278983782564183, -5.325448745358647429, -7.939653947423664704 ) ) ;
#9136=CARTESIAN_POINT ( 'NONE',  ( 26.31556265977298992, -7.384422263489805793, -5.783357778048663356 ) ) ;
#9138=CARTESIAN_POINT ( 'NONE',  ( 33.20550441965735899, -6.554320347036139971, -5.113484796970860558 ) ) ;
#9139=LINE ( 'NONE', #16890, #12983 ) ;
#9140=CARTESIAN_POINT ( 'NONE',  ( 35.41536221060850664, -16.03270077640482683, -0.5379818257722508434 ) ) ;
#9151=DIRECTION ( 'NONE',  ( -1.000000000000000000, 0.000000000000000000, 0.000000000000000000 ) ) ;
#9158=PRODUCT_DEFINITION_CONTEXT ( 'detailed design', #5728, 'design' ) ;
#9160=CARTESIAN_POINT ( 'NONE',  ( 32.93018312783485158, -2.815471066132994249, -3.627061608673662008 ) ) ;
#9167=CARTESIAN_POINT ( 'NONE',  ( 30.64918316926811315, -2.463315982128351678, -6.861505862736159145 ) ) ;
#9168=ORIENTED_EDGE ( 'NONE', *, *, #11480, .T. ) ;
#9173=CARTESIAN_POINT ( 'NONE',  ( 31.07327543742414022, -2.112412460091767308, -4.533357778048659803 ) ) ;
#9174=CARTESIAN_POINT ( 'NONE',  ( 27.75549246765397271, -7.200742295513423485, -5.783357778048668685 ) ) ;
#9175=CARTESIAN_POINT ( 'NONE',  ( 27.19802975513453092, -2.241944418315925613, -5.783357778048658027 ) ) ;
#9176=CARTESIAN_POINT ( 'NONE',  ( 30.64556327217151122, -6.525384084031224496, -7.033357778048666908 ) ) ;
#9182=DIRECTION ( 'NONE',  ( -0.000000000000000000, 1.000000000000000000, -0.000000000000000000 ) ) ;
#9187=CARTESIAN_POINT ( 'NONE',  ( -35.41536221060850664, -16.03270077640482683, -10.53798182577225084 ) ) ;
#9189=CARTESIAN_POINT ( 'NONE',  ( 33.56515079149260572, -5.873822666371450119, -6.861505862736167138 ) ) ;
#9192=CARTESIAN_POINT ( 'NONE',  ( 27.29814976067589072, -3.294147343736873346, -8.283357778048658915 ) ) ;
#9193=DIRECTION ( 'NONE',  ( -0.1196152422706611151, 0.9928203230275511881, 0.000000000000000000 ) ) ;
#9194=CARTESIAN_POINT ( 'NONE',  ( 27.48088551392658729, -7.244023872874614689, -5.783357778048657138 ) ) ;
#9201=ORIENTED_EDGE ( 'NONE', *, *, #14410, .F. ) ;
#9208=VERTEX_POINT ( 'NONE', #3152 ) ;
#9210=CARTESIAN_POINT ( 'NONE',  ( 32.07220196432897552, -5.426722983814484813, -3.627061608673668225 ) ) ;
#9213=CARTESIAN_POINT ( 'NONE',  ( -45.50000000000000000, -16.03270077640482683, -5.537981825772250843 ) ) ;
#9218=DIRECTION ( 'NONE',  ( 0.000000000000000000, 0.000000000000000000, -1.000000000000000000 ) ) ;
#9222=ORIENTED_EDGE ( 'NONE', *, *, #9964, .T. ) ;
#9227=ORIENTED_EDGE ( 'NONE', *, *, #13686, .T. ) ;
#9228=CARTESIAN_POINT ( 'NONE',  ( -19.43845002722867221, 2.988003976273734263, -6.000000000000000000 ) ) ;
#9235=CARTESIAN_POINT ( 'NONE',  ( 27.00222791626931595, -2.275731535614434531, -5.783357778048658027 ) ) ;
#9236=CARTESIAN_POINT ( 'NONE',  ( 29.86122125502053848, -4.439161430227785310, -8.283357778048662468 ) ) ;
#9239=AXIS2_PLACEMENT_3D ( 'NONE', #222, #4476, #5732 ) ;
#9240=CARTESIAN_POINT ( 'NONE',  ( 32.04575515724926760, -1.668086104879473730, -5.783357778048658027 ) ) ;
#9242=ORIENTED_EDGE ( 'NONE', *, *, #16651, .F. ) ;
#9247=PRODUCT_DEFINITION_SHAPE ( 'NONE', 'NONE',  #10978 ) ;
#9250=CARTESIAN_POINT ( 'NONE',  ( 30.88125018618674034, -3.062327022369072171, -3.627061608673662896 ) ) ;
#9255=CARTESIAN_POINT ( 'NONE',  ( 32.26287188679368967, -2.695996373064596607, -8.283357778048658915 ) ) ;
#9268=LINE ( 'NONE', #6552, #14727 ) ;
#9270=CARTESIAN_POINT ( 'NONE',  ( -29.08686357714922011, -14.78463821260646860, -13.41883458853107669 ) ) ;
#9272=DIRECTION ( 'NONE',  ( 1.000000000000000000, 0.000000000000000000, 0.000000000000000000 ) ) ;
#9273=LINE ( 'NONE', #7335, #14831 ) ;
#9274=CARTESIAN_POINT ( 'NONE',  ( 33.35047706458318828, -2.764833946905070672, -7.939653947423660263 ) ) ;
#9277=ADVANCED_FACE ( 'NONE', ( #13484 ), #6504, .T. ) ;
#9278=CARTESIAN_POINT ( 'NONE',  ( 26.47260139170898441, -4.847423203795396596, -3.283357778048664688 ) ) ;
#9280=AXIS2_PLACEMENT_3D ( 'NONE', #16366, #2748, #17748 ) ;
#9289=EDGE_CURVE ( 'NONE', #11111, #4281, #14175, .T. ) ;
#9297=AXIS2_PLACEMENT_3D ( 'NONE', #16247, #17722, #16342 ) ;
#9298=CARTESIAN_POINT ( 'NONE',  ( -38.15522249139979749, -7.597641695372263193, -5.783357778048663356 ) ) ;
#9301=CARTESIAN_POINT ( 'NONE',  ( 30.81132015408399027, -5.578634341498224458, -3.627061608673668225 ) ) ;
#9302=CIRCLE ( 'NONE', #5524, 2.000000000000001776 ) ;
#9304=FACE_OUTER_BOUND ( 'NONE', #10031, .T. ) ;
#9305=DIRECTION ( 'NONE',  ( 0.9928203230275512992, 0.1196152422706614898, -0.000000000000000000 ) ) ;
#9307=LINE ( 'NONE', #14846, #12808 ) ;
#9308=DIRECTION ( 'NONE',  ( -1.000000000000000000, 0.000000000000000000, 0.000000000000000000 ) ) ;
#9311=VERTEX_POINT ( 'NONE', #14844 ) ;
#9314=ADVANCED_FACE ( 'NONE', ( #9044 ), #706, .F. ) ;
#9320=CARTESIAN_POINT ( 'NONE',  ( 29.26075783691881682, -2.330785036554694489, -4.533357778048659803 ) ) ;
#9324=VERTEX_POINT ( 'NONE', #10389 ) ;
#9325=ORIENTED_EDGE ( 'NONE', *, *, #6806, .T. ) ;
#9329=CARTESIAN_POINT ( 'NONE',  ( 30.19827253897071273, -3.144612341114420673, -7.939653947423660263 ) ) ;
#9336=ADVANCED_FACE ( 'NONE', ( #7687 ), #8953, .F. ) ;
#9338=CARTESIAN_POINT ( 'NONE',  ( 29.49337484321020497, -2.602568060005117090, -4.705209693361161349 ) ) ;
#9341=CARTESIAN_POINT ( 'NONE',  ( 26.01652455409633902, -4.902371455920928156, -5.783357778048663356 ) ) ;
#9344=EDGE_CURVE ( 'NONE', #14154, #16640, #17521, .T. ) ;
#9345=CARTESIAN_POINT ( 'NONE',  ( 33.01342578063301403, -4.059383036018435753, -8.283357778048662468 ) ) ;
#9347=EDGE_LOOP ( 'NONE', ( #15123, #12404, #5735, #14876 ) ) ;
#9355=CIRCLE ( 'NONE', #2425, 2.749999999999995559 ) ;
#9356=ORIENTED_EDGE ( 'NONE', *, *, #2968, .T. ) ;
#9357=CARTESIAN_POINT ( 'NONE',  ( 45.50000000000000000, -16.03270077640482683, -5.537981825772250843 ) ) ;
#9362=DIRECTION ( 'NONE',  ( -0.1196152422706614760, 0.9928203230275510771, 0.000000000000000000 ) ) ;
#9363=CARTESIAN_POINT ( 'NONE',  ( 33.17547354829333273, -5.293800545841212291, -3.627061608673667781 ) ) ;
#9367=CARTESIAN_POINT ( 'NONE',  ( 26.01595305975170547, -2.384361315936983416, -5.783357778048670461 ) ) ;
#9376=CYLINDRICAL_SURFACE ( 'NONE', #16893, 2.000000000000001776 ) ;
#9379=CARTESIAN_POINT ( 'NONE',  ( 32.96459815279162342, -1.884545423566157174, -4.533357778048659803 ) ) ;
#9381=CARTESIAN_POINT ( 'NONE',  ( 29.52399153675929355, -1.971908820246954130, -5.783357778048658027 ) ) ;
#9388=ORIENTED_EDGE ( 'NONE', *, *, #2701, .F. ) ;
#9389=FACE_OUTER_BOUND ( 'NONE', #13737, .T. ) ;
#9390=DIRECTION ( 'NONE',  ( 0.000000000000000000, 0.000000000000000000, 1.000000000000000000 ) ) ;
#9406=ADVANCED_FACE ( 'NONE', ( #10565, #16129 ), #2430, .T. ) ;
#9408=CARTESIAN_POINT ( 'NONE',  ( 0.000000000000000000, 0.000000000000000000, -8.700000000000001066 ) ) ;
#9409=CARTESIAN_POINT ( 'NONE',  ( 18.32916366311290091, -12.06017896066153128, -15.79554754021495633 ) ) ;
#9413=CARTESIAN_POINT ( 'NONE',  ( 30.18087924896149588, -5.654590020340094725, -3.627061608673668225 ) ) ;
#9420=CARTESIAN_POINT ( 'NONE',  ( 26.84461768998868436, -2.294720455324902542, -5.783357778048658915 ) ) ;
#9424=DIRECTION ( 'NONE',  ( -0.1196152422706611984, 0.9928203230275510771, 0.000000000000000000 ) ) ;
#9426=CARTESIAN_POINT ( 'NONE',  ( 29.67353201968042598, -1.554147106732884920, -5.783357778048658027 ) ) ;
#9427=ORIENTED_EDGE ( 'NONE', *, *, #13074, .T. ) ;
#9430=CARTESIAN_POINT ( 'NONE',  ( 33.40754056521197413, -5.892811586081919906, -6.861505862736166250 ) ) ;
#9432=CARTESIAN_POINT ( 'NONE',  ( 31.71807556108801407, -1.697368162559112825, -5.113484796970855228 ) ) ;
#9441=DIRECTION ( 'NONE',  ( -0.1196152422706611984, 0.9928203230275510771, 0.000000000000000000 ) ) ;
#9443=DIRECTION ( 'NONE',  ( 0.000000000000000000, 0.000000000000000000, 1.000000000000000000 ) ) ;
#9444=CARTESIAN_POINT ( 'NONE',  ( 30.43486631442457835, -6.877930660435475296, -5.783357778048669573 ) ) ;
#9446=CARTESIAN_POINT ( 'NONE',  ( -1.917618200156724081E-28, -7.000000000000001776, -6.000000000000000000 ) ) ;
#9448=CARTESIAN_POINT ( 'NONE',  ( 33.40301380667672504, -2.758504307001591549, -3.627061608673662896 ) ) ;
#9450=DIRECTION ( 'NONE',  ( 0.000000000000000000, 0.000000000000000000, -1.000000000000000000 ) ) ;
#9451=CARTESIAN_POINT ( 'NONE',  ( 13.65694651542703397, -25.37101204406936361, -16.45580752066269881 ) ) ;
#9459=CARTESIAN_POINT ( 'NONE',  ( -14.00000000000000178, 0.000000000000000000, -8.700000000000001066 ) ) ;
#9465=CARTESIAN_POINT ( 'NONE',  ( 28.51709679197739078, -3.347160818026084339, -3.627061608673662008 ) ) ;
#9475=B_SPLINE_CURVE_WITH_KNOTS ( 'NONE', 3,
 ( #3674, #11912, #8103, #17760, #14908, #3939, #7849, #13638, #12279, #16024, #2490, #17587, #17501, #5107, #16200, #3765, #9539, #4118, #6832, #2671, #14083, #12358, #10887, #16632, #15352, #1489, #6918, #8366, #2760, #11149, #15087, #13809, #12714, #8200, #5546, #13896, #9626, #2931, #7116, #37, #8551, #9801, #4290 ),
 .UNSPECIFIED., .F., .F.,
 ( 4, 2, 2, 1, 2, 2, 2, 2, 2, 2, 2, 2, 2, 2, 2, 2, 2, 2, 2, 2, 2, 4 ),
 ( 0.01976987703536532692, 0.02100501831352976842, 0.02162258895261198396, 0.02224015959169420298, 0.02285773023077641852, 0.02347530086985863407, 0.02471044214802306516, 0.02594558342618749971, 0.02718072470435193080, 0.02779829534343414288, 0.02841586598251635495, 0.02965100726068079298, 0.03088614853884522754, 0.03150371917792745002, 0.03212128981700967945, 0.03335643109517413829, 0.03459157237333859714, 0.03582671365150305598, 0.03644428429058528540, 0.03706185492966751482, 0.03829699620783197367, 0.03953213748599642557 ),
 .UNSPECIFIED. ) ;
#9479=VERTEX_POINT ( 'NONE', #13913 ) ;
#9487=CYLINDRICAL_SURFACE ( 'NONE', #2033, 6.249999999999998224 ) ;
#9488=PLANE ( 'NONE',  #8750 ) ;
#9489=CIRCLE ( 'NONE', #3434, 13.00000000000000178 ) ;
#9490=CARTESIAN_POINT ( 'NONE',  ( -2.016448651773435938E-27, -20.49999999999999645, -13.00000000000000178 ) ) ;
#9493=CARTESIAN_POINT ( 'NONE',  ( 19.91392456697921531, -10.76755109436559010, -15.52754005891982736 ) ) ;
#9496=EDGE_CURVE ( 'NONE', #1259, #9479, #16499, .T. ) ;
#9497=CARTESIAN_POINT ( 'NONE',  ( 31.04338717100262102, -6.177645381738930297, -6.861505862736167138 ) ) ;
#9502=ADVANCED_FACE ( 'NONE', ( #17779 ), #6581, .T. ) ;
#9503=ORIENTED_EDGE ( 'NONE', *, *, #14916, .T. ) ;
#9505=CARTESIAN_POINT ( 'NONE',  ( 26.88845778707760914, -3.543379655034240905, -7.939653947423660263 ) ) ;
#9511=CIRCLE ( 'NONE', #5176, 14.00000000000000178 ) ;
#9512=LINE ( 'NONE', #17821, #16286 ) ;
#9513=CARTESIAN_POINT ( 'NONE',  ( 29.98133424373737910, -5.878503772023492502, -8.283357778048662468 ) ) ;
#9515=CARTESIAN_POINT ( 'NONE',  ( 31.88814493096863956, -1.687075024589942851, -5.783357778048658027 ) ) ;
#9516=FACE_OUTER_BOUND ( 'NONE', #6514, .T. ) ;
#9517=CARTESIAN_POINT ( 'NONE',  ( 30.08145424927873535, -6.930706697444451336, -5.783357778048663356 ) ) ;
#9521=AXIS2_PLACEMENT_3D ( 'NONE', #17338, #4968, #3628 ) ;
#9522=VERTEX_POINT ( 'NONE', #5211 ) ;
#9526=CARTESIAN_POINT ( 'NONE',  ( 26.01652455409633902, -4.902371455920928156, -5.783357778048663356 ) ) ;
#9527=EDGE_LOOP ( 'NONE', ( #2063, #9427, #7099, #13832 ) ) ;
#9530=CARTESIAN_POINT ( 'NONE',  ( 30.39102621733566423, -5.629271460726127607, -7.939653947423662927 ) ) ;
#9533=ORIENTED_EDGE ( 'NONE', *, *, #194, .F. ) ;
#9535=CARTESIAN_POINT ( 'NONE',  ( 26.87785582392756467, -3.344784462964796479, -3.283357778048662023 ) ) ;
#9539=CARTESIAN_POINT ( 'NONE',  ( 25.20704250852812933, -22.06899625087205763, -14.42769424659100785 ) ) ;
#9540=( BOUNDED_CURVE ( )  B_SPLINE_CURVE ( 3, ( #14729, #13092, #2313, #17196 ),
 .UNSPECIFIED., .F., .T. ) 
 B_SPLINE_CURVE_WITH_KNOTS ( ( 4, 4 ),
 ( 1.316154292592045083, 1.436990331221392081 ),
 .UNSPECIFIED. ) 
 CURVE ( )  GEOMETRIC_REPRESENTATION_ITEM ( )  RATIONAL_B_SPLINE_CURVE ( ( 1.000000000000000000, 0.9987835910734581546, 0.9987835910734581546, 1.000000000000000000 ) ) 
 REPRESENTATION_ITEM ( '' )  );
#9549=EDGE_LOOP ( 'NONE', ( #17563, #7586, #1112, #10588 ) ) ;
#9552=CARTESIAN_POINT ( 'NONE',  ( 30.19827253897071273, -3.144612341114420673, -7.939653947423660263 ) ) ;
#9562=ORIENTED_EDGE ( 'NONE', *, *, #16936, .T. ) ;
#9565=EDGE_LOOP ( 'NONE', ( #14077, #6307, #14391, #11517, #1632, #11250, #4718, #6108, #4154, #16514, #8630, #15363, #15709, #15638, #5870, #113, #1628, #7036, #14770, #13032, #8452, #16621, #3363, #993, #14757, #12974, #146, #5712 ) ) ;
#9569=CARTESIAN_POINT ( 'NONE',  ( 33.24613200752366282, -6.212066908601060256, -7.033357778048666908 ) ) ;
#9576=ORIENTED_EDGE ( 'NONE', *, *, #13213, .F. ) ;
#9577=CARTESIAN_POINT ( 'NONE',  ( 28.28955653359400557, -5.882457056865704637, -3.627061608673668225 ) ) ;
#9587=CARTESIAN_POINT ( 'NONE',  ( 28.75786045390062995, -2.691183018653962034, -6.861505862736159145 ) ) ;
#9589=CARTESIAN_POINT ( 'NONE',  ( 25.87953856062030766, -3.765371892057810754, -3.950981403410641857 ) ) ;
#9592=DIRECTION ( 'NONE',  ( -0.1196152422706626278, 0.9928203230275510771, 0.000000000000000000 ) ) ;
#9595=CARTESIAN_POINT ( 'NONE',  ( 28.69037342443288452, -3.126411886501869741, -3.283357778048662023 ) ) ;
#9598=FACE_OUTER_BOUND ( 'NONE', #815, .T. ) ;
#9600=CARTESIAN_POINT ( 'NONE',  ( 30.63309003953906995, -6.864245478665264244, -5.783357778048663356 ) ) ;
#9602=LINE ( 'NONE', #9689, #6147 ) ;
#9605=AXIS2_PLACEMENT_3D ( 'NONE', #5931, #11455, #10097 ) ;
#9606=AXIS2_PLACEMENT_3D ( 'NONE', #11685, #7888, #10504 ) ;
#9609=CARTESIAN_POINT ( 'NONE',  ( 5.500000000000000000, -20.49999999999999645, -6.000000000000000000 ) ) ;
#9613=CARTESIAN_POINT ( 'NONE',  ( 34.25812524399339765, -6.427500325324513319, -5.783357778048663356 ) ) ;
#9616=CARTESIAN_POINT ( 'NONE',  ( 28.91999743871649997, -5.806501378023834370, -3.627061608673668225 ) ) ;
#9620=ORIENTED_EDGE ( 'NONE', *, *, #12752, .F. ) ;
#9621=CARTESIAN_POINT ( 'NONE',  ( 32.14213199643172914, -2.910415664685331638, -3.627061608673662896 ) ) ;
#9626=CARTESIAN_POINT ( 'NONE',  ( 17.40734525178378078, -19.01589366988068974, -15.93907283187074775 ) ) ;
#9627=ORIENTED_EDGE ( 'NONE', *, *, #11915, .T. ) ;
#9628=VECTOR ( 'NONE', #12616, 1000.000000000000227 ) ;
#9630=CARTESIAN_POINT ( 'NONE',  ( 20.00000000000000000, 7.999999999999996447, 0.000000000000000000 ) ) ;
#9638=CARTESIAN_POINT ( 'NONE',  ( 30.15443244188179150, -1.895953141405084086, -5.783357778048658027 ) ) ;
#9645=EDGE_CURVE ( 'NONE', #1319, #3307, #9913, .T. ) ;
#9660=DIRECTION ( 'NONE',  ( 0.000000000000000000, 0.000000000000000000, -1.000000000000000000 ) ) ;
#9667=CARTESIAN_POINT ( 'NONE',  ( 28.89355063163679915, -2.047864499088824175, -5.783357778048658027 ) ) ;
#9671=CARTESIAN_POINT ( 'NONE',  ( 31.89397184978405519, -6.712334120981523711, -5.783357778048663356 ) ) ;
#9675=CARTESIAN_POINT ( 'NONE',  ( 29.41022140756759029, -3.239556939666760726, -7.939653947423660263 ) ) ;
#9676=LINE ( 'NONE', #15227, #7486 ) ;
#9677=CARTESIAN_POINT ( 'NONE',  ( -5.499998817156067865, -20.49639288455253450, -12.00000000000000000 ) ) ;
#9678=LINE ( 'NONE', #13865, #6996 ) ;
#9683=CARTESIAN_POINT ( 'NONE',  ( 29.35089333861488115, -5.954459450865362768, -8.283357778048662468 ) ) ;
#9684=ORIENTED_EDGE ( 'NONE', *, *, #16011, .F. ) ;
#9686=CARTESIAN_POINT ( 'NONE',  ( 30.64918316926811315, -2.463315982128351678, -6.861505862736159145 ) ) ;
#9689=CARTESIAN_POINT ( 'NONE',  ( -15.92260893619738837, -28.39189527176317540, -12.00000000000000000 ) ) ;
#9697=ORIENTED_EDGE ( 'NONE', *, *, #15992, .F. ) ;
#9700=CARTESIAN_POINT ( 'NONE',  ( 31.67382807612511542, -6.101689702897060030, -6.861505862736167138 ) ) ;
#9703=CARTESIAN_POINT ( 'NONE',  ( 31.71314141467879111, -4.216041623526076698, -3.627061608673664672 ) ) ;
#9710=ORIENTED_EDGE ( 'NONE', *, *, #17001, .F. ) ;
#9717=CARTESIAN_POINT ( 'NONE',  ( 26.01652455409633902, -4.902371455920928156, -5.783357778048663356 ) ) ;
#9719=CARTESIAN_POINT ( 'NONE',  ( 27.77288575766320378, -4.690764616287755651, -7.939653947423662039 ) ) ;
#9720=CARTESIAN_POINT ( 'NONE',  ( 45.00000000000000711, 0.000000000000000000, -5.537981825772250843 ) ) ;
#9723=CARTESIAN_POINT ( 'NONE',  ( 0.000000000000000000, 0.000000000000000000, -10.50000000000000000 ) ) ;
#9729=EDGE_LOOP ( 'NONE', ( #17051, #11759 ) ) ;
#9738=DIRECTION ( 'NONE',  ( -0.1196152422706611984, 0.9928203230275510771, 0.000000000000000000 ) ) ;
#9743=( BOUNDED_CURVE ( )  B_SPLINE_CURVE ( 2, ( #650, #11877, #2114, #17360, #15982, #6174, #3724, #11697, #17266 ),
 .UNSPECIFIED., .F., .T. ) 
 B_SPLINE_CURVE_WITH_KNOTS ( ( 3, 2, 2, 2, 3 ),
 ( 0.5576923076923077094, 0.5641025641025640969, 0.5769230769230768718, 0.5897435897435897578, 0.5961538461538461453 ),
 .UNSPECIFIED. ) 
 CURVE ( )  GEOMETRIC_REPRESENTATION_ITEM ( )  RATIONAL_B_SPLINE_CURVE ( ( 0.9330127018922194093, 0.9330127018922194093, 1.000000000000000000, 0.8660254037844387076, 1.000000000000000000, 0.8660254037844387076, 1.000000000000000000, 0.9330127018922194093, 0.9330127018922194093 ) ) 
 REPRESENTATION_ITEM ( '' )  );
#9745=DIRECTION ( 'NONE',  ( 0.000000000000000000, 0.000000000000000000, 1.000000000000000000 ) ) ;
#9746=VECTOR ( 'NONE', #3854, 1000.000000000000000 ) ;
#9747=CARTESIAN_POINT ( 'NONE',  ( 23.84286890107044954, -10.01213378893004879, -14.74186762137086859 ) ) ;
#9751=ORIENTED_EDGE ( 'NONE', *, *, #985, .F. ) ;
#9754=VERTEX_POINT ( 'NONE', #15641 ) ;
#9760=CARTESIAN_POINT ( 'NONE',  ( 25.75741033704265703, -2.751693534003876174, -5.973512092880350011 ) ) ;
#9761=CARTESIAN_POINT ( 'NONE',  ( 20.00000000000000000, 7.999999999999996447, -15.51150668642334374 ) ) ;
#9764=EDGE_CURVE ( 'NONE', #3060, #15522, #11871, .T. ) ;
#9767=VECTOR ( 'NONE', #5326, 1000.000000000000227 ) ;
#9768=CARTESIAN_POINT ( 'NONE',  ( 36.27615609941022257, -23.17738945083361557, -12.00000000000000000 ) ) ;
#9769=( BOUNDED_CURVE ( )  B_SPLINE_CURVE ( 2, ( #13587, #5228, #6782, #17708, #3804, #1168, #9320, #10578, #7790 ),
 .UNSPECIFIED., .F., .T. ) 
 B_SPLINE_CURVE_WITH_KNOTS ( ( 3, 2, 2, 2, 3 ),
 ( 0.4423076923076923461, 0.4487179487179487336, 0.4615384615384615641, 0.4743589743589743390, 0.4807692307692307820 ),
 .UNSPECIFIED. ) 
 CURVE ( )  GEOMETRIC_REPRESENTATION_ITEM ( )  RATIONAL_B_SPLINE_CURVE ( ( 0.9330127018922194093, 0.9330127018922196314, 1.000000000000000000, 0.8660254037844387076, 1.000000000000000000, 0.8660254037844387076, 1.000000000000000000, 0.9330127018922190762, 0.9330127018922194093 ) ) 
 REPRESENTATION_ITEM ( '' )  );
#9770=CARTESIAN_POINT ( 'NONE',  ( 28.15758777499317489, -7.552042790248305160, -5.783357778048669573 ) ) ;
#9771=CARTESIAN_POINT ( 'NONE',  ( 30.88577694472199298, -6.196634301449400084, -6.861505862736166250 ) ) ;
#9772=VECTOR ( 'NONE', #16741, 1000.000000000000000 ) ;
#9774=CARTESIAN_POINT ( 'NONE',  ( 14.00000000000000178, 1.714505518806294835E-15, -10.50000000000000000 ) ) ;
#9780=ORIENTED_EDGE ( 'NONE', *, *, #11689, .F. ) ;
#9783=CARTESIAN_POINT ( 'NONE',  ( 30.54048978798443059, -6.538043363838207611, -4.533357778048668685 ) ) ;
#9785=DIRECTION ( 'NONE',  ( 0.000000000000000000, 1.000000000000000000, 0.000000000000000000 ) ) ;
#9788=CARTESIAN_POINT ( 'NONE',  ( 30.82871344409320713, -3.068656662272551294, -7.939653947423660263 ) ) ;
#9793=CARTESIAN_POINT ( 'NONE',  ( 30.04066231269008469, -3.163601260824890904, -7.939653947423660263 ) ) ;
#9797=ORIENTED_EDGE ( 'NONE', *, *, #14891, .T. ) ;
#9801=CARTESIAN_POINT ( 'NONE',  ( 16.75000000000000355, -16.63579488892710145, -16.03574476417184158 ) ) ;
#9802=ORIENTED_EDGE ( 'NONE', *, *, #12695, .F. ) ;
#9804=AXIS2_PLACEMENT_3D ( 'NONE', #10644, #6231, #7866 ) ;
#9816=CARTESIAN_POINT ( 'NONE',  ( 27.86926259684567597, -5.933094176093606897, -7.939653947423664704 ) ) ;
#9817=CARTESIAN_POINT ( 'NONE',  ( 32.27410075503257758, -1.240829931302721345, -5.783357778048658027 ) ) ;
#9822=CYLINDRICAL_SURFACE ( 'NONE', #8758, 2.749999999999992006 ) ;
#9823=CARTESIAN_POINT ( 'NONE',  ( 30.42903939560917337, -1.852671564043892660, -5.783357778048658027 ) ) ;
#9828=EDGE_LOOP ( 'NONE', ( #5204, #16869, #17131, #3018, #11335, #17853 ) ) ;
#9831=SURFACE_STYLE_USAGE ( .BOTH. , #5849 ) ;
#9841=CARTESIAN_POINT ( 'NONE',  ( -30.05650519998691195, -5.408673599982547486, -13.28483438372753156 ) ) ;
#9849=DIRECTION ( 'NONE',  ( 0.000000000000000000, -1.000000000000000000, 0.000000000000000000 ) ) ;
#9854=CARTESIAN_POINT ( 'NONE',  ( 26.99805802979993885, -6.665027654307603022, -4.705209693361168455 ) ) ;
#9856=LINE ( 'NONE', #6979, #575 ) ;
#9860=CARTESIAN_POINT ( 'NONE',  ( 31.95146207396702565, -5.641142275435199416, -8.283357778048664244 ) ) ;
#9864=CARTESIAN_POINT ( 'NONE',  ( 28.05993251931039012, -3.202367565343739564, -3.283357778048662023 ) ) ;
#9867=CARTESIAN_POINT ( 'NONE',  ( 28.75786045390062995, -2.691183018653962034, -6.861505862736159145 ) ) ;
#9880=DIRECTION ( 'NONE',  ( 0.000000000000000000, 0.000000000000000000, -1.000000000000000000 ) ) ;
#9882=CARTESIAN_POINT ( 'NONE',  ( -23.43428999263575818, -9.970190943884908563, -14.83168556311182940 ) ) ;
#9884=EDGE_LOOP ( 'NONE', ( #6305, #10370, #7930, #17787 ) ) ;
#9889=CARTESIAN_POINT ( 'NONE',  ( 30.25080928106424594, -3.138282701210941994, -3.627061608673662896 ) ) ;
#9891=CARTESIAN_POINT ( 'NONE',  ( 26.01652455409633902, -4.902371455920928156, -5.783357778048663356 ) ) ;
#9895=CARTESIAN_POINT ( 'NONE',  ( 29.54600080245929306, -4.477139269648729325, -3.283357778048664688 ) ) ;
#9896=EDGE_LOOP ( 'NONE', ( #13852, #8514, #17613, #16402 ) ) ;
#9906=EDGE_LOOP ( 'NONE', ( #1402, #12792, #17047, #11782 ) ) ;
#9909=CARTESIAN_POINT ( 'NONE',  ( 27.53153627355490229, -7.237921456612971483, -5.113484796970862334 ) ) ;
#9910=CARTESIAN_POINT ( 'NONE',  ( 27.12922144900085186, -2.887401855662130146, -4.705209693361160461 ) ) ;
#9911=CARTESIAN_POINT ( 'NONE',  ( 31.32102116884452414, -5.717097954277069682, -8.283357778048662468 ) ) ;
#9913=LINE ( 'NONE', #14016, #5776 ) ;
#9914=SHAPE_DEFINITION_REPRESENTATION ( #9247, #5639 ) ;
#9915=CARTESIAN_POINT ( 'NONE',  ( 30.44283453230164227, -2.188368138933637574, -4.533357778048659803 ) ) ;
#9920=ADVANCED_FACE ( 'NONE', ( #7576, #2233 ), #14379, .T. ) ;
#9925=DIRECTION ( 'NONE',  ( 0.000000000000000000, 0.000000000000000000, -1.000000000000000000 ) ) ;
#9941=CARTESIAN_POINT ( 'NONE',  ( 29.82675284572052732, -1.925235199084722959, -5.113484796970855228 ) ) ;
#9946=EDGE_CURVE ( 'NONE', #12386, #1259, #7846, .T. ) ;
#9948=CARTESIAN_POINT ( 'NONE',  ( 26.46816385032927599, -3.594016774262162262, -3.627061608673662896 ) ) ;
#9956=ADVANCED_FACE ( 'NONE', ( #953 ), #7481, .T. ) ;
#9957=LINE ( 'NONE', #15594, #13703 ) ;
#9959=CARTESIAN_POINT ( 'NONE',  ( 30.13703915187255689, -4.405930820630744371, -7.939653947423662039 ) ) ;
#9961=CARTESIAN_POINT ( 'NONE',  ( -35.41536221060850664, -16.03270077640482683, -0.5379818257722508434 ) ) ;
#9962=CARTESIAN_POINT ( 'NONE',  ( 35.41536221060850664, -16.03270077640482683, -0.5379818257722508434 ) ) ;
#9964=EDGE_CURVE ( 'NONE', #2784, #17331, #17359, .T. ) ;
#9970=ORIENTED_EDGE ( 'NONE', *, *, #4828, .T. ) ;
#9971=CARTESIAN_POINT ( 'NONE',  ( -20.27735869291019810, -10.58859781672278899, -15.46157951461808189 ) ) ;
#9973=CARTESIAN_POINT ( 'NONE',  ( 27.75966235412334981, -2.811446176820259879, -4.705209693361160461 ) ) ;
#9976=ORIENTED_EDGE ( 'NONE', *, *, #17477, .T. ) ;
#9978=CARTESIAN_POINT ( 'NONE',  ( 29.19137779418881351, -4.519864338893556877, -3.627061608673664672 ) ) ;
#9979=FACE_OUTER_BOUND ( 'NONE', #868, .T. ) ;
#9983=EDGE_CURVE ( 'NONE', #11718, #15344, #5220, .T. ) ;
#9998=CARTESIAN_POINT ( 'NONE',  ( 26.63030083514515312, -6.709335133632020387, -6.861505862736167138 ) ) ;
#9999=CARTESIAN_POINT ( 'NONE',  ( 30.66050125466253107, -2.889050389913576655, -3.283357778048662023 ) ) ;
#10003=CARTESIAN_POINT ( 'NONE',  ( 28.28502977505876359, -2.748149777785362957, -6.861505862736158257 ) ) ;
#10005=CYLINDRICAL_SURFACE ( 'NONE', #9605, 2.499999999999999112 ) ;
#10006=DIRECTION ( 'NONE',  ( 0.000000000000000000, 0.000000000000000000, 1.000000000000000000 ) ) ;
#10014=CYLINDRICAL_SURFACE ( 'NONE', #17502, 2.749999999999992895 ) ;
#10023=ADVANCED_FACE ( 'NONE', ( #3007, #4797 ), #8714, .T. ) ;
#10030=CYLINDRICAL_SURFACE ( 'NONE', #17962, 2.000000000000001776 ) ;
#10031=EDGE_LOOP ( 'NONE', ( #4127, #13040, #10536, #14059 ) ) ;
#10032=VERTEX_POINT ( 'NONE', #10319 ) ;
#10033=ORIENTED_EDGE ( 'NONE', *, *, #2887, .F. ) ;
#10040=LINE ( 'NONE', #8605, #3821 ) ;
#10044=EDGE_CURVE ( 'NONE', #2932, #15540, #17068, .T. ) ;
#10045=CARTESIAN_POINT ( 'NONE',  ( 20.25000000000001066, -16.21813761408365195, -13.00000000000000355 ) ) ;
#10048=CARTESIAN_POINT ( 'NONE',  ( 30.88125018618674744, -3.062327022369072171, -3.627061608673662896 ) ) ;
#10049=DIRECTION ( 'NONE',  ( 0.000000000000000000, 0.000000000000000000, 1.000000000000000000 ) ) ;
#10050=CARTESIAN_POINT ( 'NONE',  ( 32.26971135134834867, -1.630906943779925955, -5.113484796970855228 ) ) ;
#10052=ORIENTED_EDGE ( 'NONE', *, *, #6195, .T. ) ;
#10057=ORIENTED_EDGE ( 'NONE', *, *, #10749, .F. ) ;
#10061=LINE ( 'NONE', #16620, #31 ) ;
#10068=CARTESIAN_POINT ( 'NONE',  ( 31.27962407439061110, -2.387360303286481855, -6.861505862736159145 ) ) ;
#10069=DIRECTION ( 'NONE',  ( -0.000000000000000000, 1.000000000000000000, -0.000000000000000000 ) ) ;
#10071=DIRECTION ( 'NONE',  ( -1.000000000000000000, 0.000000000000000000, 0.000000000000000000 ) ) ;
#10072=VERTEX_POINT ( 'NONE', #4712 ) ;
#10085=EDGE_CURVE ( 'NONE', #7303, #11429, #11594, .T. ) ;
#10090=VECTOR ( 'NONE', #17136, 1000.000000000000000 ) ;
#10091=CARTESIAN_POINT ( 'NONE',  ( 32.93832978346670615, -1.887710243310447567, -7.033357778048658027 ) ) ;
#10095=CARTESIAN_POINT ( 'NONE',  ( 29.13014440709066832, -5.781182818409868140, -7.939653947423664704 ) ) ;
#10097=DIRECTION ( 'NONE',  ( -0.1196152422706611984, 0.9928203230275510771, 0.000000000000000000 ) ) ;
#10107=CARTESIAN_POINT ( 'NONE',  ( -45.50000000000000000, -19.03270077640483038, -5.537981825772250843 ) ) ;
#10108=ORIENTED_EDGE ( 'NONE', *, *, #4941, .F. ) ;
#10109=CARTESIAN_POINT ( 'NONE',  ( 32.83754810739939956, -9.116730809865838836, -5.783357778048662468 ) ) ;
#10113=CIRCLE ( 'NONE', #17690, 5.000000000000000000 ) ;
#10114=CARTESIAN_POINT ( 'NONE',  ( -25.07353123778395343, 1.235291682954730463, -14.60266621045499669 ) ) ;
#10127=( BOUNDED_CURVE ( )  B_SPLINE_CURVE ( 2, ( #3512, #16128, #7865, #10642, #6414, #11931, #11665, #6503, #16043 ),
 .UNSPECIFIED., .F., .T. ) 
 B_SPLINE_CURVE_WITH_KNOTS ( ( 3, 2, 2, 2, 3 ),
 ( 0.6346153846153846922, 0.6410256410256410797, 0.6538461538461538547, 0.6666666666666666297, 0.6730769230769231282 ),
 .UNSPECIFIED. ) 
 CURVE ( )  GEOMETRIC_REPRESENTATION_ITEM ( )  RATIONAL_B_SPLINE_CURVE ( ( 0.9330127018922192983, 0.9330127018922198534, 1.000000000000000000, 0.8660254037844387076, 1.000000000000000000, 0.8660254037844387076, 1.000000000000000000, 0.9330127018922187432, 0.9330127018922192983 ) ) 
 REPRESENTATION_ITEM ( '' )  );
#10131=DIRECTION ( 'NONE',  ( 0.9928203230275512992, 0.1196152422706614898, -0.000000000000000000 ) ) ;
#10135=CARTESIAN_POINT ( 'NONE',  ( -21.03357387009699409, -22.15422581635157684, -15.32066355758547083 ) ) ;
#10137=CARTESIAN_POINT ( 'NONE',  ( 31.71123609653335507, -2.762457591843783256, -8.283357778048660691 ) ) ;
#10139=CARTESIAN_POINT ( 'NONE',  ( 0.000000000000000000, 0.000000000000000000, -6.000000000000000000 ) ) ;
#10143=CARTESIAN_POINT ( 'NONE',  ( 27.93049598394382116, -4.671775696577297410, -3.627061608673664672 ) ) ;
#10146=CARTESIAN_POINT ( 'NONE',  ( 26.11428532722776197, -5.713797161519015511, -3.668609639089262409 ) ) ;
#10153=EDGE_LOOP ( 'NONE', ( #6116, #11029, #14894, #2516 ) ) ;
#10155=DIRECTION ( 'NONE',  ( 0.000000000000000000, 1.000000000000000000, 3.469446951953614189E-16 ) ) ;
#10162=CARTESIAN_POINT ( 'NONE',  ( 27.02867472334902033, -6.034368414549445170, -3.627061608673668225 ) ) ;
#10163=CARTESIAN_POINT ( 'NONE',  ( 26.62577407660990758, -3.575027854551694695, -3.627061608673662008 ) ) ;
#10165=CARTESIAN_POINT ( 'NONE',  ( 28.56093688906631911, -4.595820017735426255, -3.627061608673664672 ) ) ;
#10167=DIRECTION ( 'NONE',  ( -0.1196152422706626278, 0.9928203230275510771, 0.000000000000000000 ) ) ;
#10173=PLANE ( 'NONE',  #2257 ) ;
#10183=ORIENTED_EDGE ( 'NONE', *, *, #15758, .T. ) ;
#10185=CARTESIAN_POINT ( 'NONE',  ( 26.64639396487419987, -2.308405637095112706, -5.783357778048658027 ) ) ;
#10186=VECTOR ( 'NONE', #16392, 1000.000000000000000 ) ;
#10187=CIRCLE ( 'NONE', #13683, 13.00000000000000178 ) ;
#10189=CARTESIAN_POINT ( 'NONE',  ( 32.51061761821408425, -6.300681867249914525, -4.533357778048668685 ) ) ;
#10194=CARTESIAN_POINT ( 'NONE',  ( 27.22618411036838637, -2.238552374514887866, -5.113484796970851676 ) ) ;
#10195=FACE_OUTER_BOUND ( 'NONE', #14851, .T. ) ;
#10198=ADVANCED_FACE ( 'NONE', ( #11573, #2986 ), #5774, .T. ) ;
#10199=AXIS2_PLACEMENT_3D ( 'NONE', #11808, #15537, #14180 ) ;
#10201=CONICAL_SURFACE ( 'NONE', #7622, 3.999999999999986677, 0.7853981633974400633 ) ;
#10208=CARTESIAN_POINT ( 'NONE',  ( 32.83754810739938534, -9.116730809865837060, 4.216642221951339309 ) ) ;
#10211=CARTESIAN_POINT ( 'NONE',  ( 32.26287188679368256, -2.695996373064596607, -8.283357778048660691 ) ) ;
#10220=CIRCLE ( 'NONE', #8201, 13.00000000000000178 ) ;
#10224=ORIENTED_EDGE ( 'NONE', *, *, #13003, .F. ) ;
#10227=CARTESIAN_POINT ( 'NONE',  ( -20.00000000000000000, 7.999999999999996447, -15.51150668642334374 ) ) ;
#10228=CARTESIAN_POINT ( 'NONE',  ( -28.68370877339674863, -18.82577899785919584, -13.53184763361698906 ) ) ;
#10230=DIRECTION ( 'NONE',  ( 0.000000000000000000, 0.000000000000000000, -1.000000000000000000 ) ) ;
#10233=EDGE_CURVE ( 'NONE', #947, #6789, #10299, .T. ) ;
#10234=CARTESIAN_POINT ( 'NONE',  ( 26.39379627684682106, -4.856917663858078882, -3.283357778048664688 ) ) ;
#10238=CARTESIAN_POINT ( 'NONE',  ( 25.71072941247523502, -3.058302133056337357, -4.705209693361161349 ) ) ;
#10241=FACE_OUTER_BOUND ( 'NONE', #14505, .T. ) ;
#10245=CARTESIAN_POINT ( 'NONE',  ( 31.51169109130924184, -2.986371343527201905, -3.627061608673662896 ) ) ;
#10247=CARTESIAN_POINT ( 'NONE',  ( 29.45101334415624095, -7.006662376286321603, -5.783357778048657138 ) ) ;
#10248=CARTESIAN_POINT ( 'NONE',  ( 25.79194807336802953, -3.038360733637177624, -6.974889548725401234 ) ) ;
#10249=CARTESIAN_POINT ( 'NONE',  ( -34.91600907648203389, -11.88801210197604341, -11.56671555609732671 ) ) ;
#10250=CARTESIAN_POINT ( 'NONE',  ( 27.63266882139180325, -2.199775856772564708, -5.783357778048658915 ) ) ;
#10251=CARTESIAN_POINT ( 'NONE',  ( 27.28266178881210280, -7.257709054644824853, -5.783357778048669573 ) ) ;
#10253=CARTESIAN_POINT ( 'NONE',  ( 27.72904566057427189, -3.442105416578422172, -3.627061608673662896 ) ) ;
#10255=CARTESIAN_POINT ( 'NONE',  ( 33.13353876934985465, -5.498725377814142057, -8.283357778048664244 ) ) ;
#10258=( BOUNDED_CURVE ( )  B_SPLINE_CURVE ( 2, ( #15062, #13710, #16695, #4272, #6815, #2258, #4622, #12882, #14249 ),
 .UNSPECIFIED., .F., .T. ) 
 B_SPLINE_CURVE_WITH_KNOTS ( ( 3, 2, 2, 2, 3 ),
 ( 0.8653846153846154188, 0.8717948717948718063, 0.8846153846153845812, 0.8974358974358974672, 0.9038461538461538547 ),
 .UNSPECIFIED. ) 
 CURVE ( )  GEOMETRIC_REPRESENTATION_ITEM ( )  RATIONAL_B_SPLINE_CURVE ( ( 0.9330127018922192983, 0.9330127018922198534, 1.000000000000000000, 0.8660254037844387076, 1.000000000000000000, 0.8660254037844387076, 1.000000000000000000, 0.9330127018922194093, 0.9330127018922194093 ) ) 
 REPRESENTATION_ITEM ( '' )  );
#10260=EDGE_CURVE ( 'NONE', #15308, #1274, #15117, .T. ) ;
#10269=CARTESIAN_POINT ( 'NONE',  ( -45.50000000000000000, -16.03270077640482683, -2.787981825772258837 ) ) ;
#10274=CARTESIAN_POINT ( 'NONE',  ( 28.58911057998038530, -6.046239229258517867, -3.283357778048667797 ) ) ;
#10277=PLANE ( 'NONE',  #10662 ) ;
#10282=EDGE_CURVE ( 'NONE', #963, #12549, #2056, .T. ) ;
#10288=CYLINDRICAL_SURFACE ( 'NONE', #4419, 2.499999999999999112 ) ;
#10290=CARTESIAN_POINT ( 'NONE',  ( 25.90934487712385348, 0.1208734971681838660, -5.783357778048663356 ) ) ;
#10294=CARTESIAN_POINT ( 'NONE',  ( 33.13163345120441505, -4.045141346131868154, -3.627061608673664672 ) ) ;
#10299=LINE ( 'NONE', #16133, #10429 ) ;
#10309=CARTESIAN_POINT ( 'NONE',  ( -24.62400252878131113, -22.25686381702613659, -14.56428162264008286 ) ) ;
#10311=CARTESIAN_POINT ( 'NONE',  ( 31.03132594549780876, -1.780107929003061473, -6.453230759126465266 ) ) ;
#10313=DIRECTION ( 'NONE',  ( -0.000000000000000000, -0.000000000000000000, -1.000000000000000000 ) ) ;
#10318=CARTESIAN_POINT ( 'NONE',  ( 33.32855701603872234, -2.140504347050403045, -6.861505862736158257 ) ) ;
#10319=CARTESIAN_POINT ( 'NONE',  ( -13.00000000000000178, 1.592040838891559293E-15, -6.000000000000000000 ) ) ;
#10321=ORIENTED_EDGE ( 'NONE', *, *, #6917, .F. ) ;
#10326=EDGE_CURVE ( 'NONE', #9479, #15536, #13131, .T. ) ;
#10329=CARTESIAN_POINT ( 'NONE',  ( 32.04158527077989760, -6.057382223572642665, -4.705209693361168455 ) ) ;
#10330=EDGE_LOOP ( 'NONE', ( #13202, #799 ) ) ;
#10332=CARTESIAN_POINT ( 'NONE',  ( 25.76775864925888015, -2.837585720338237749, -6.439571894700457655 ) ) ;
#10333=VERTEX_POINT ( 'NONE', #9140 ) ;
#10337=CARTESIAN_POINT ( 'NONE',  ( 33.73390066541284682, -2.518766455766909385, -3.283357778048662023 ) ) ;
#10339=VECTOR ( 'NONE', #8831, 1000.000000000000227 ) ;
#10341=CARTESIAN_POINT ( 'NONE',  ( 28.36401332423200827, -6.500457016816879374, -6.861505862736166250 ) ) ;
#10342=LINE ( 'NONE', #15895, #5238 ) ;
#10343=CARTESIAN_POINT ( 'NONE',  ( 27.16987539990068612, -2.245336462116964249, -6.453230759126464378 ) ) ;
#10344=CARTESIAN_POINT ( 'NONE',  ( 0.000000000000000000, 0.000000000000000000, -8.700000000000001066 ) ) ;
#10349=AXIS2_PLACEMENT_3D ( 'NONE', #8249, #2727, #1449 ) ;
#10352=DIRECTION ( 'NONE',  ( 0.000000000000000000, 0.000000000000000000, -1.000000000000000000 ) ) ;
#10354=ORIENTED_EDGE ( 'NONE', *, *, #1656, .T. ) ;
#10357=CARTESIAN_POINT ( 'NONE',  ( 31.89397184978405519, -6.712334120981523711, -5.783357778048663356 ) ) ;
#10358=CARTESIAN_POINT ( 'NONE',  ( 15.92260893619738837, -28.39189527176317540, -16.15082599432113142 ) ) ;
#10361=CARTESIAN_POINT ( 'NONE',  ( 28.99436501219896201, -4.543600488427916417, -3.283357778048664688 ) ) ;
#10367=CARTESIAN_POINT ( 'NONE',  ( 31.07327543742414022, -2.112412460091767308, -4.533357778048659803 ) ) ;
#10370=ORIENTED_EDGE ( 'NONE', *, *, #6215, .F. ) ;
#10389=CARTESIAN_POINT ( 'NONE',  ( -8.632250723006720250, -18.84644399697197770, -13.00000000000000178 ) ) ;
#10400=ORIENTED_EDGE ( 'NONE', *, *, #10044, .F. ) ;
#10406=DIRECTION ( 'NONE',  ( -0.000000000000000000, -0.000000000000000000, -1.000000000000000000 ) ) ;
#10407=CARTESIAN_POINT ( 'NONE',  ( -18.90235488073503944, -20.95521764957430122, -15.70196361584510392 ) ) ;
#10410=LINE ( 'NONE', #11587, #16838 ) ;
#10412=CARTESIAN_POINT ( 'NONE',  ( 26.31175009776946538, -7.352777558617343168, -6.181997573440047411 ) ) ;
#10416=CARTESIAN_POINT ( 'NONE',  ( 26.23609683341064525, -2.995005734021441768, -6.861505862736159145 ) ) ;
#10420=CLOSED_SHELL ( 'NONE', ( #8130, #8300, #75, #7140, #1111, #7860, #2450, #13546, #1157, #8545, #2323, #11140, #17492, #14873, #13867, #7625, #13408, #11710, #13464, #127, #1064, #10909, #4464, #12719, #3396, #7165, #1333, #5233, #14264, #11776, #9314, #2333, #14748, #3970, #14676, #8432, #11355, #2810, #4318, #15148, #13585, #16449, #6236, #10198, #8936, #12623, #5237, #5079, #14010, #17838, #1253, #1286, #9019, #6941, #9277, #13394, #498, #3311, #4340, #3763, #13878, #12469, #11559, #15001, #5117, #13614, #14042, #12293, #13695, #14188, #10023, #6591, #4246, #326, #9406, #9956, #15886, #9502, #9920, #7896, #1878, #5784, #8304, #10812, #6515, #17332, #14632, #5665, #13905, #4083, #11873, #4890, #2133, #5880, #15494, #11858, #3847, #5109, #6475, #15271, #9336, #14615, #8868, #8679, #6038, #5916 ) ) ;
#10423=CARTESIAN_POINT ( 'NONE',  ( 33.17094678975809074, -2.159493266760871499, -6.861505862736159145 ) ) ;
#10427=CARTESIAN_POINT ( 'NONE',  ( 31.12210306526553083, -4.287250072544045665, -8.283357778048662468 ) ) ;
#10429=VECTOR ( 'NONE', #3516, 1000.000000000000227 ) ;
#10431=CARTESIAN_POINT ( 'NONE',  ( 30.33776104811456165, -2.201027418740610919, -7.033357778048658027 ) ) ;
#10435=CARTESIAN_POINT ( 'NONE',  ( 26.97161122272022382, -2.906390775372597712, -4.705209693361161349 ) ) ;
#10438=CARTESIAN_POINT ( 'NONE',  ( 6.540214080563054644, 17.14393242671841477, -16.94648454462088694 ) ) ;
#10443=LINE ( 'NONE', #16003, #10339 ) ;
#10451=CARTESIAN_POINT ( 'NONE',  ( 31.66930131758986633, -2.967382423816733894, -3.627061608673662008 ) ) ;
#10452=LINE ( 'NONE', #16103, #10502 ) ;
#10455=CARTESIAN_POINT ( 'NONE',  ( 27.86101441917510257, -1.772519683195811657, -5.783357778048658027 ) ) ;
#10457=EDGE_CURVE ( 'NONE', #15335, #3112, #7805, .T. ) ;
#10459=CARTESIAN_POINT ( 'NONE',  ( 29.25000000000000000, -16.21813761408365195, -13.00000000000000178 ) ) ;
#10460=CARTESIAN_POINT ( 'NONE',  ( 11.38175538881591287, -22.33742387525453665, -16.67884400577319681 ) ) ;
#10463=CARTESIAN_POINT ( 'NONE',  ( 27.65467808709180630, -4.705006306174339237, -3.283357778048664688 ) ) ;
#10464=CARTESIAN_POINT ( 'NONE',  ( 31.89397184978405519, -6.712334120981523711, -5.783357778048663356 ) ) ;
#10476=CARTESIAN_POINT ( 'NONE',  ( 33.56515079149260572, -5.873822666371450119, -6.861505862736167138 ) ) ;
#10480=DIRECTION ( 'NONE',  ( 0.9928203230275510771, 0.1196152422706614621, -0.000000000000000000 ) ) ;
#10483=EDGE_CURVE ( 'NONE', #1653, #7229, #11607, .T. ) ;
#10485=CARTESIAN_POINT ( 'NONE',  ( 26.23123039439649062, -6.684454722870800225, -4.255767710538254534 ) ) ;
#10488=AXIS2_PLACEMENT_3D ( 'NONE', #15600, #382, #468 ) ;
#10492=ORIENTED_EDGE ( 'NONE', *, *, #13199, .F. ) ;
#10493=EDGE_LOOP ( 'NONE', ( #4334, #14303, #5708 ) ) ;
#10496=ORIENTED_EDGE ( 'NONE', *, *, #12537, .F. ) ;
#10502=VECTOR ( 'NONE', #6203, 1000.000000000000000 ) ;
#10504=DIRECTION ( 'NONE',  ( -1.000000000000000000, 0.000000000000000000, 0.000000000000000000 ) ) ;
#10506=SHAPE_REPRESENTATION_RELATIONSHIP ( 'NONE' , 'NONE' ,  #5639, #17227 ) ;
#10508=CARTESIAN_POINT ( 'NONE',  ( 27.60205212784272177, -2.830435096530727446, -4.705209693361161349 ) ) ;
#10516=CARTESIAN_POINT ( 'NONE',  ( 31.49429780130001788, -5.496349022752856861, -7.939653947423662927 ) ) ;
#10521=CARTESIAN_POINT ( 'NONE',  ( 8.632250723006720250, -18.84644399697197770, -13.00000000000000178 ) ) ;
#10524=CARTESIAN_POINT ( 'NONE',  ( 32.50309786422735669, -5.574681056656012323, -8.283357778048662468 ) ) ;
#10525=CARTESIAN_POINT ( 'NONE',  ( 25.83772294520678159, -3.669972453104032084, -3.627061608673662896 ) ) ;
#10526=DIRECTION ( 'NONE',  ( 0.9928203230275510771, 0.1196152422706614621, -0.000000000000000000 ) ) ;
#10534=CARTESIAN_POINT ( 'NONE',  ( -36.27615609941022257, -23.17738945083361202, -11.07596365154449636 ) ) ;
#10536=ORIENTED_EDGE ( 'NONE', *, *, #17702, .T. ) ;
#10541=CARTESIAN_POINT ( 'NONE',  ( 29.39961944441754227, -3.040961747597316300, -3.283357778048662023 ) ) ;
#10544=CARTESIAN_POINT ( 'NONE',  ( 15.92260893619738837, -28.39189527176317540, -16.15082599432113142 ) ) ;
#10561=CARTESIAN_POINT ( 'NONE',  ( 33.35047706458318828, -2.764833946905071560, -7.939653947423660263 ) ) ;
#10565=FACE_BOUND ( 'NONE', #3159, .T. ) ;
#10569=CARTESIAN_POINT ( 'NONE',  ( 31.70371634254663817, -2.036456781249897485, -4.533357778048659803 ) ) ;
#10571=ORIENTED_EDGE ( 'NONE', *, *, #8693, .F. ) ;
#10578=CARTESIAN_POINT ( 'NONE',  ( 29.19631194059803292, -2.001190877926593004, -5.113484796970855228 ) ) ;
#10580=DIRECTION ( 'NONE',  ( -1.000000000000000000, 0.000000000000000000, 0.000000000000000000 ) ) ;
#10583=CARTESIAN_POINT ( 'NONE',  ( 26.49878054387835746, -2.963357534503999968, -4.705209693361160461 ) ) ;
#10585=EDGE_CURVE ( 'NONE', #17331, #13453, #13924, .T. ) ;
#10586=CARTESIAN_POINT ( 'NONE',  ( 31.06530721954707985, -6.801974981593605030, -5.783357778048669573 ) ) ;
#10588=ORIENTED_EDGE ( 'NONE', *, *, #3067, .T. ) ;
#10591=VERTEX_POINT ( 'NONE', #8064 ) ;
#10593=CARTESIAN_POINT ( 'NONE',  ( 32.14213199643173624, -2.910415664685331638, -3.627061608673662896 ) ) ;
#10595=EDGE_CURVE ( 'NONE', #8691, #14539, #13600, .T. ) ;
#10596=VERTEX_POINT ( 'NONE', #4891 ) ;
#10598=CARTESIAN_POINT ( 'NONE',  ( 25.77386970449396841, -2.888308184441632953, -6.623114134516397300 ) ) ;
#10599=CARTESIAN_POINT ( 'NONE',  ( 28.72797218747911074, -6.756415940301135237, -4.533357778048668685 ) ) ;
#10601=CARTESIAN_POINT ( 'NONE',  ( 31.56485473504790917, -1.326280070207274564, -5.783357778048658027 ) ) ;
#10602=EDGE_CURVE ( 'NONE', #1274, #1497, #2170, .T. ) ;
#10603=( BOUNDED_CURVE ( )  B_SPLINE_CURVE ( 2, ( #16968, #8706, #14053, #10137, #12778, #9860, #15685, #15414, #11490 ),
 .UNSPECIFIED., .F., .T. ) 
 B_SPLINE_CURVE_WITH_KNOTS ( ( 3, 2, 2, 2, 3 ),
 ( 0.1730769230769231004, 0.1794871794871794879, 0.1923076923076923184, 0.2051282051282051211, 0.2115384615384615641 ),
 .UNSPECIFIED. ) 
 CURVE ( )  GEOMETRIC_REPRESENTATION_ITEM ( )  RATIONAL_B_SPLINE_CURVE ( ( 0.9330127018922194093, 0.9330127018922196314, 1.000000000000000000, 0.8660254037844387076, 1.000000000000000000, 0.8660254037844387076, 1.000000000000000000, 0.9330127018922190762, 0.9330127018922194093 ) ) 
 REPRESENTATION_ITEM ( '' )  );
#10605=CARTESIAN_POINT ( 'NONE',  ( 32.77709966008947617, -5.968767264923789284, -6.861505862736166250 ) ) ;
#10606=CARTESIAN_POINT ( 'NONE',  ( -30.07408527595751124, -27.82894256842315883, -13.18310524188696853 ) ) ;
#10608=CARTESIAN_POINT ( 'NONE',  ( 3.248936832696173393, 17.78798921770683350, -17.00000000000000000 ) ) ;
#10617=CIRCLE ( 'NONE', #15261, 2.749999999999995559 ) ;
#10618=CARTESIAN_POINT ( 'NONE',  ( 33.43363050022580296, -2.127845067243429256, -4.705209693361160461 ) ) ;
#10620=CARTESIAN_POINT ( 'NONE',  ( 29.46348657678868577, -6.667800981652280967, -7.033357778048666908 ) ) ;
#10621=CARTESIAN_POINT ( 'NONE',  ( -7.499998387031003411, -20.49508120620799900, -13.00000000000000178 ) ) ;
#10622=LINE ( 'NONE', #8196, #8359 ) ;
#10638=ORIENTED_EDGE ( 'NONE', *, *, #6111, .T. ) ;
#10642=CARTESIAN_POINT ( 'NONE',  ( 28.48022645605872327, -3.151730446115816875, -8.283357778048660691 ) ) ;
#10644=CARTESIAN_POINT ( 'NONE',  ( 36.27615609941022257, -23.17738945083361557, -12.00000000000000000 ) ) ;
#10661=CARTESIAN_POINT ( 'NONE',  ( 0.000000000000000000, 0.000000000000000000, -12.00000000000000000 ) ) ;
#10662=AXIS2_PLACEMENT_3D ( 'NONE', #14573, #6297, #16018 ) ;
#10665=CARTESIAN_POINT ( 'NONE',  ( 27.04606801335823718, -3.524390735323772006, -7.939653947423660263 ) ) ;
#10668=CARTESIAN_POINT ( 'NONE',  ( 31.03886041246737548, -3.043338102658604161, -3.627061608673662008 ) ) ;
#10676=CARTESIAN_POINT ( 'NONE',  ( 29.36638131047866906, -1.990897739957422807, -5.783357778048658915 ) ) ;
#10677=AXIS2_PLACEMENT_3D ( 'NONE', #7435, #1639, #5961 ) ;
#10678=LINE ( 'NONE', #13522, #12176 ) ;
#10682=CARTESIAN_POINT ( 'NONE',  ( 30.64556327217151122, -6.525384084031224496, -7.033357778048666908 ) ) ;
#10684=CARTESIAN_POINT ( 'NONE',  ( 32.65880277236253448, -4.102108105263264193, -7.939653947423662039 ) ) ;
#10685=CARTESIAN_POINT ( 'NONE',  ( 32.83754810739939956, -9.116730809865838836, -5.783357778048662468 ) ) ;
#10688=EDGE_LOOP ( 'NONE', ( #12813, #846, #13576, #7939, #7347 ) ) ;
#10690=VECTOR ( 'NONE', #5827, 1000.000000000000000 ) ;
#10691=EDGE_CURVE ( 'NONE', #2104, #5268, #6984, .T. ) ;
#10696=ORIENTED_EDGE ( 'NONE', *, *, #6293, .T. ) ;
#10702=CARTESIAN_POINT ( 'NONE',  ( 32.93018312783485868, -2.815471066132993805, -3.627061608673662008 ) ) ;
#10706=CARTESIAN_POINT ( 'NONE',  ( 25.33925079868512498, -2.076342398563292058, -5.783357778048658027 ) ) ;
#10709=FACE_OUTER_BOUND ( 'NONE', #17245, .T. ) ;
#10710=DIRECTION ( 'NONE',  ( -0.1196152422706611984, 0.9928203230275510771, 0.000000000000000000 ) ) ;
#10722=ORIENTED_EDGE ( 'NONE', *, *, #4737, .F. ) ;
#10727=CARTESIAN_POINT ( 'NONE',  ( 30.60986983071443390, -4.348964061499348333, -3.627061608673664672 ) ) ;
#10729=CARTESIAN_POINT ( 'NONE',  ( 30.42903939560917337, -1.852671564043892660, -5.783357778048658027 ) ) ;
#10734=DIRECTION ( 'NONE',  ( 0.3420201433256631063, 0.000000000000000000, 0.9396926207859104263 ) ) ;
#10735=CARTESIAN_POINT ( 'NONE',  ( 31.24973580796908834, -6.452593224933654170, -4.533357778048668685 ) ) ;
#10747=CARTESIAN_POINT ( 'NONE',  ( 5.500000000000000888, -20.49999999999999645, -13.00000000000000178 ) ) ;
#10749=EDGE_CURVE ( 'NONE', #227, #13758, #13357, .T. ) ;
#10750=CARTESIAN_POINT ( 'NONE',  ( 27.41826274939272423, -4.733489685532582314, -8.283357778048662468 ) ) ;
#10752=CARTESIAN_POINT ( 'NONE',  ( -15.92260893619738837, -28.39189527176317540, -12.00000000000000000 ) ) ;
#10754=CARTESIAN_POINT ( 'NONE',  ( -29.25000000000000000, -16.21813761408365195, -13.00000000000000178 ) ) ;
#10755=CARTESIAN_POINT ( 'NONE',  ( 26.39370705969127684, -2.976016814310973313, -6.861505862736158257 ) ) ;
#10758=AXIS2_PLACEMENT_3D ( 'NONE', #3977, #12490, #4064 ) ;
#10759=CARTESIAN_POINT ( 'NONE',  ( 30.43486631442457835, -6.877930660435475296, -5.783357778048669573 ) ) ;
#10762=DIRECTION ( 'NONE',  ( 0.9928203230275512992, 0.1196152422706614898, -0.000000000000000000 ) ) ;
#10767=AXIS2_PLACEMENT_3D ( 'NONE', #6500, #12016, #14841 ) ;
#10768=CARTESIAN_POINT ( 'NONE',  ( 27.30005507882132676, -4.747731375419166788, -3.627061608673664672 ) ) ;
#10774=CARTESIAN_POINT ( 'NONE',  ( 31.87265695910486230, -5.650636735497883478, -8.283357778048662468 ) ) ;
#10777=CARTESIAN_POINT ( 'NONE',  ( 33.27602027394517847, -2.146833986953896822, -4.705209693361161349 ) ) ;
#10780=CARTESIAN_POINT ( 'NONE',  ( 30.63309003953906995, -6.864245478665264244, -5.783357778048663356 ) ) ;
#10784=CARTESIAN_POINT ( 'NONE',  ( 25.71748644841968456, -2.420320648352051851, -5.783357778048663356 ) ) ;
#10791=EDGE_CURVE ( 'NONE', #13499, #17849, #10342, .T. ) ;
#10792=CARTESIAN_POINT ( 'NONE',  ( 30.18087924896149588, -5.654590020340094725, -3.627061608673668225 ) ) ;
#10795=CARTESIAN_POINT ( 'NONE',  ( 32.56242593318007295, -2.859778545457410281, -7.939653947423660263 ) ) ;
#10796=EDGE_CURVE ( 'NONE', #17749, #11736, #15084, .T. ) ;
#10809=CARTESIAN_POINT ( 'NONE',  ( 3.538288549924106796, -15.34800872113743431, -13.00000000000000178 ) ) ;
#10812=ADVANCED_FACE ( 'NONE', ( #6184 ), #5906, .F. ) ;
#10815=CARTESIAN_POINT ( 'NONE',  ( 29.04699097144805364, -6.418171698071525100, -4.705209693361169343 ) ) ;
#10817=PLANE ( 'NONE',  #14454 ) ;
#10824=CARTESIAN_POINT ( 'NONE',  ( -36.27615609941022257, -23.17738945083361557, -12.00000000000000000 ) ) ;
#10825=CARTESIAN_POINT ( 'NONE',  ( 27.36943512155133362, -2.558652073080304845, -4.533357778048659803 ) ) ;
#10829=ORIENTED_EDGE ( 'NONE', *, *, #5534, .T. ) ;
#10839=FACE_OUTER_BOUND ( 'NONE', #10936, .T. ) ;
#10840=DIRECTION ( 'NONE',  ( 0.000000000000000000, 0.000000000000000000, 1.000000000000000000 ) ) ;
#10841=FACE_OUTER_BOUND ( 'NONE', #16802, .T. ) ;
#10845=CARTESIAN_POINT ( 'NONE',  ( 21.03312194624853149, -10.28219102306256971, -15.32075016948875934 ) ) ;
#10848=CARTESIAN_POINT ( 'NONE',  ( 31.87075164095941915, -4.197052703815608687, -3.627061608673664672 ) ) ;
#10851=EDGE_CURVE ( 'NONE', #12969, #17574, #3998, .T. ) ;
#10852=CARTESIAN_POINT ( 'NONE',  ( -21.42601376483257880, 2.765314980223223529, -6.000000000000000000 ) ) ;
#10855=CARTESIAN_POINT ( 'NONE',  ( 28.10549950023367316, -2.142809097641162897, -5.783357778048658915 ) ) ;
#10862=CARTESIAN_POINT ( 'NONE',  ( 28.41265020943543362, -1.706058464416624787, -5.783357778048658027 ) ) ;
#10863=ORIENTED_EDGE ( 'NONE', *, *, #4737, .T. ) ;
#10864=CARTESIAN_POINT ( 'NONE',  ( 32.54050588463559990, -2.235448945602741766, -6.861505862736159145 ) ) ;
#10874=ORIENTED_EDGE ( 'NONE', *, *, #10457, .T. ) ;
#10875=( LENGTH_UNIT ( ) NAMED_UNIT ( * ) SI_UNIT ( .MILLI., .METRE. ) );
#10876=CARTESIAN_POINT ( 'NONE',  ( 31.69574812466957781, -6.726019302751734763, -5.783357778048669573 ) ) ;
#10878=CARTESIAN_POINT ( 'NONE',  ( -5.237433445017501299, -16.51494876461869765, -16.99438405180048761 ) ) ;
#10881=CARTESIAN_POINT ( 'NONE',  ( 32.79901970863393501, -6.593096864778464017, -5.783357778048668685 ) ) ;
#10882=B_SPLINE_CURVE_WITH_KNOTS ( 'NONE', 3,
 ( #4299, #1590, #7123, #16823, #13095, #4561 ),
 .UNSPECIFIED., .F., .F.,
 ( 4, 2, 4 ),
 ( 0.5339563158597049330, 0.5927605480271135319, 0.6515647801945221307 ),
 .UNSPECIFIED. ) ;
#10887=CARTESIAN_POINT ( 'NONE',  ( 22.62413451274595388, -22.47014588436322668, -15.00416998627796694 ) ) ;
#10892=ORIENTED_EDGE ( 'NONE', *, *, #16608, .T. ) ;
#10893=DIRECTION ( 'NONE',  ( 0.000000000000000000, 0.000000000000000000, 1.000000000000000000 ) ) ;
#10897=CARTESIAN_POINT ( 'NONE',  ( 31.41531425212677675, -1.744041783721344219, -5.783357778048658027 ) ) ;
#10902=CARTESIAN_POINT ( 'NONE',  ( 29.78612525785423060, -2.267488637519798012, -7.033357778048658027 ) ) ;
#10907=CARTESIAN_POINT ( 'NONE',  ( 28.09753128235661279, -6.832371619143005503, -4.533357778048668685 ) ) ;
#10909=ADVANCED_FACE ( 'NONE', ( #9979 ), #13078, .F. ) ;
#10914=ORIENTED_EDGE ( 'NONE', *, *, #3123, .F. ) ;
#10920=CIRCLE ( 'NONE', #6614, 2.749999999999995559 ) ;
#10922=CARTESIAN_POINT ( 'NONE',  ( 28.79925754835455010, -6.020920669644549861, -8.283357778048664244 ) ) ;
#10925=CARTESIAN_POINT ( 'NONE',  ( 28.59583933521957277, -13.42685997174391765, -13.55623838816837079 ) ) ;
#10927=ORIENTED_EDGE ( 'NONE', *, *, #12068, .T. ) ;
#10929=CARTESIAN_POINT ( 'NONE',  ( 31.55553118839817728, -4.235030543236534939, -7.939653947423662039 ) ) ;
#10931=FACE_OUTER_BOUND ( 'NONE', #12707, .T. ) ;
#10936=EDGE_LOOP ( 'NONE', ( #12289, #7282, #11095, #11577 ) ) ;
#10940=CARTESIAN_POINT ( 'NONE',  ( 28.77978050244509944, -3.315512618508630549, -7.939653947423660263 ) ) ;
#10942=ORIENTED_EDGE ( 'NONE', *, *, #938, .F. ) ;
#10947=CIRCLE ( 'NONE', #12418, 2.749999999999988454 ) ;
#10949=EDGE_CURVE ( 'NONE', #12531, #1954, #3317, .T. ) ;
#10950=CARTESIAN_POINT ( 'NONE',  ( 29.27960797773944179, -6.689954721521948144, -4.533357778048668685 ) ) ;
#10953=DIRECTION ( 'NONE',  ( 0.000000000000000000, 0.000000000000000000, 1.000000000000000000 ) ) ;
#10957=LINE ( 'NONE', #13712, #14254 ) ;
#10964=FACE_OUTER_BOUND ( 'NONE', #9527, .T. ) ;
#10965=ORIENTED_EDGE ( 'NONE', *, *, #14376, .F. ) ;
#10966=AXIS2_PLACEMENT_3D ( 'NONE', #12200, #1145, #2685 ) ;
#10968=CARTESIAN_POINT ( 'NONE',  ( 28.89355063163679915, -2.047864499088824175, -5.783357778048658915 ) ) ;
#10972=CARTESIAN_POINT ( 'NONE',  ( 26.31128205117621022, -7.047579375861630524, -7.033357778048666908 ) ) ;
#10973=CARTESIAN_POINT ( 'NONE',  ( 25.11802603177690330, -19.03270077640482683, -10.53798182577225084 ) ) ;
#10976=CARTESIAN_POINT ( 'NONE',  ( 29.97449477918272009, -6.943593201308171814, -5.113484796970856117 ) ) ;
#10978=PRODUCT_DEFINITION ( 'UNKNOWN', '', #17901, #9158 ) ;
#10979=AXIS2_PLACEMENT_3D ( 'NONE', #3650, #8993, #3560 ) ;
#10984=ORIENTED_EDGE ( 'NONE', *, *, #3088, .T. ) ;
#10987=ORIENTED_EDGE ( 'NONE', *, *, #3672, .T. ) ;
#10988=ORIENTED_EDGE ( 'NONE', *, *, #11657, .F. ) ;
#10991=CARTESIAN_POINT ( 'NONE',  ( 31.04338717100262102, -6.177645381738930297, -6.861505862736167138 ) ) ;
#11002=ORIENTED_EDGE ( 'NONE', *, *, #14879, .T. ) ;
#11003=CIRCLE ( 'NONE', #3790, 2.749999999999995559 ) ;
#11012=CARTESIAN_POINT ( 'NONE',  ( 33.09223089549517738, -4.049888575955752579, -8.283357778048662468 ) ) ;
#11022=AXIS2_PLACEMENT_3D ( 'NONE', #8855, #4411, #11174 ) ;
#11023=CARTESIAN_POINT ( 'NONE',  ( 28.91999743871649997, -5.806501378023834370, -3.627061608673668225 ) ) ;
#11024=EDGE_CURVE ( 'NONE', #8021, #6497, #14240, .T. ) ;
#11027=CARTESIAN_POINT ( 'NONE',  ( 31.92212620501791775, -6.708942077180482855, -6.453230759126470595 ) ) ;
#11028=ORIENTED_EDGE ( 'NONE', *, *, #1484, .F. ) ;
#11029=ORIENTED_EDGE ( 'NONE', *, *, #1420, .T. ) ;
#11032=CARTESIAN_POINT ( 'NONE',  ( 30.25533603959949502, -6.272589980291270351, -6.861505862736166250 ) ) ;
#11039=VECTOR ( 'NONE', #16149, 1000.000000000000227 ) ;
#11040=EDGE_CURVE ( 'NONE', #2553, #548, #1608, .T. ) ;
#11042=CARTESIAN_POINT ( 'NONE',  ( 26.79905070906540132, -3.354278923027479209, -3.283357778048662023 ) ) ;
#11044=CARTESIAN_POINT ( 'NONE',  ( 31.30154412293507349, -3.011689903141150815, -7.939653947423660263 ) ) ;
#11046=EDGE_CURVE ( 'NONE', #13310, #4693, #2394, .T. ) ;
#11047=CARTESIAN_POINT ( 'NONE',  ( 28.04870365451522218, -4.657534006690712935, -8.283357778048662468 ) ) ;
#11048=DIRECTION ( 'NONE',  ( 0.000000000000000000, -1.000000000000000000, -3.469446951953614189E-16 ) ) ;
#11053=B_SPLINE_CURVE_WITH_KNOTS ( 'NONE', 3,
 ( #8968, #11680, #14417, #4789, #805, #13046, #14331, #2094, #17438, #11584, #14236, #720, #10407, #17057, #7618, #15962, #14608, #10135, #11766, #1914, #14511, #3529, #8704, #5962, #15683, #10309, #6245, #4969, #17339, #4877, #15866, #6335, #17250, #8883, #9061, #15588, #1825, #10228, #6156, #11488, #3264, #7525, #7701 ),
 .UNSPECIFIED., .F., .F.,
 ( 4, 2, 2, 1, 2, 2, 2, 2, 2, 2, 2, 2, 2, 2, 2, 2, 2, 2, 2, 2, 2, 4 ),
 ( 0.01976914256504654077, 0.02100445419277401429, 0.02162211000663775626, 0.02223976582050150169, 0.02285742163436524366, 0.02347507744822898562, 0.02471038907595646955, 0.02594570070368395695, 0.02718101233141144435, 0.02779866814527519325, 0.02841632395913894216, 0.02965163558686643996, 0.03088694721459393777, 0.03150460302845767974, 0.03212225884232142170, 0.03335757047004890563, 0.03459288209777638956, 0.03582819372550387349, 0.03644584953936762239, 0.03706350535323135742, 0.03829881698095885523, 0.03953412860868634610 ),
 .UNSPECIFIED. ) ;
#11055=EDGE_CURVE ( 'NONE', #12535, #6942, #16357, .T. ) ;
#11056=VERTEX_POINT ( 'NONE', #9175 ) ;
#11060=CARTESIAN_POINT ( 'NONE',  ( -16.95520570318904419, -14.57695177659950581, -16.00609026697356541 ) ) ;
#11062=CARTESIAN_POINT ( 'NONE',  ( 29.80442540930208750, -6.953886339277345563, -5.783357778048669573 ) ) ;
#11065=CARTESIAN_POINT ( 'NONE',  ( 25.84216048658649001, -4.923378882637265974, -3.283357778048664688 ) ) ;
#11066=PLANE ( 'NONE',  #5120 ) ;
#11073=CARTESIAN_POINT ( 'NONE',  ( 45.50000000000000000, -16.03270077640482683, -8.287981825772238409 ) ) ;
#11080=CARTESIAN_POINT ( 'NONE',  ( 26.62577407660990758, -3.575027854551694695, -3.627061608673662008 ) ) ;
#11082=CYLINDRICAL_SURFACE ( 'NONE', #12992, 5.000000000000000000 ) ;
#11086=CARTESIAN_POINT ( 'NONE',  ( 28.11132641904908169, -7.168068194032743534, -5.783357778048668685 ) ) ;
#11087=CARTESIAN_POINT ( 'NONE',  ( 13.00000000000000178, 0.000000000000000000, -12.00000000000000000 ) ) ;
#11090=ORIENTED_EDGE ( 'NONE', *, *, #16397, .F. ) ;
#11091=EDGE_CURVE ( 'NONE', #2761, #1161, #12088, .T. ) ;
#11095=ORIENTED_EDGE ( 'NONE', *, *, #3542, .T. ) ;
#11097=EDGE_LOOP ( 'NONE', ( #13386, #2659, #5030, #11352 ) ) ;
#11102=CARTESIAN_POINT ( 'NONE',  ( 26.31556265977298992, -7.384422263489805793, -5.783357778048663356 ) ) ;
#11104=CARTESIAN_POINT ( 'NONE',  ( 45.50000000000000000, -16.03270077640482683, -5.537981825772250843 ) ) ;
#11105=CARTESIAN_POINT ( 'NONE',  ( 16.91330062320331962, -14.78391025039656625, -16.01216328675237577 ) ) ;
#11110=DIRECTION ( 'NONE',  ( -1.000000000000000000, 0.000000000000000000, 0.000000000000000000 ) ) ;
#11111=VERTEX_POINT ( 'NONE', #7091 ) ;
#11115=CARTESIAN_POINT ( 'NONE',  ( 26.49461065740898391, -7.352653653197164907, -5.783357778048668685 ) ) ;
#11117=CARTESIAN_POINT ( 'NONE',  ( 25.76974524478944062, -2.854074692636065169, -5.141149657938114181 ) ) ;
#11118=CARTESIAN_POINT ( 'NONE',  ( 30.05650519998692971, -5.408673599982567026, -13.28483438372752445 ) ) ;
#11120=CARTESIAN_POINT ( 'NONE',  ( 31.51612863268893960, -4.239777773060436239, -3.283357778048664688 ) ) ;
#11124=CARTESIAN_POINT ( 'NONE',  ( 35.74085044863416982, -23.57886868891565513, -11.27079897466147251 ) ) ;
#11125=CARTESIAN_POINT ( 'NONE',  ( 27.33945763453056088, -4.742984145595265488, -8.283357778048662468 ) ) ;
#11126=CARTESIAN_POINT ( 'NONE',  ( 29.36638131047866196, -1.990897739957422807, -5.783357778048658027 ) ) ;
#11135=CARTESIAN_POINT ( 'NONE',  ( 32.36819060393585801, 0.8990368551114588103, -5.783357778048663356 ) ) ;
#11138=LINE ( 'NONE', #1571, #3534 ) ;
#11140=ADVANCED_FACE ( 'NONE', ( #9516 ), #4271, .F. ) ;
#11141=CARTESIAN_POINT ( 'NONE',  ( 31.45915434921569798, -2.992700983430681028, -7.939653947423660263 ) ) ;
#11142=DIRECTION ( 'NONE',  ( -0.000000000000000000, 1.000000000000000000, 0.000000000000000000 ) ) ;
#11144=CARTESIAN_POINT ( 'NONE',  ( 31.51169109130924184, -2.986371343527201905, -3.627061608673662896 ) ) ;
#11149=CARTESIAN_POINT ( 'NONE',  ( 19.91592223102268733, -21.66952118561269458, -15.52717098632164117 ) ) ;
#11150=EDGE_LOOP ( 'NONE', ( #7010, #14200, #14131, #11653 ) ) ;
#11156=CARTESIAN_POINT ( 'NONE',  ( 32.34167700165585302, -2.686501913001913433, -8.283357778048660691 ) ) ;
#11158=FACE_OUTER_BOUND ( 'NONE', #13644, .T. ) ;
#11161=CARTESIAN_POINT ( 'NONE',  ( 25.78518620311324838, -3.676302093007511651, -7.939653947423660263 ) ) ;
#11163=CARTESIAN_POINT ( 'NONE',  ( 31.15208055228630357, -2.102918000029084578, -4.533357778048659803 ) ) ;
#11172=VERTEX_POINT ( 'NONE', #9600 ) ;
#11174=DIRECTION ( 'NONE',  ( -0.1196152422706611984, 0.9928203230275510771, 0.000000000000000000 ) ) ;
#11176=VERTEX_POINT ( 'NONE', #1371 ) ;
#11178=AXIS2_PLACEMENT_3D ( 'NONE', #12424, #2904, #11312 ) ;
#11184=DIRECTION ( 'NONE',  ( 0.000000000000000000, 0.000000000000000000, 1.000000000000000000 ) ) ;
#11188=DIRECTION ( 'NONE',  ( 1.000000000000000000, 0.000000000000000000, 0.000000000000000000 ) ) ;
#11189=DIRECTION ( 'NONE',  ( -1.000000000000000000, 0.000000000000000000, -0.000000000000000000 ) ) ;
#11201=CARTESIAN_POINT ( 'NONE',  ( 28.91555989733679866, -4.553094948490599592, -3.283357778048664688 ) ) ;
#11206=CARTESIAN_POINT ( 'NONE',  ( -36.07773319708005744, -23.32620662758124297, -11.14818368178938357 ) ) ;
#11207=CARTESIAN_POINT ( 'NONE',  ( 0.000000000000000000, 0.000000000000000000, -12.00000000000000000 ) ) ;
#11208=CARTESIAN_POINT ( 'NONE',  ( 45.00000000000000711, -19.03270077640482683, -10.53798182577225084 ) ) ;
#11209=EDGE_CURVE ( 'NONE', #11560, #2108, #17457, .T. ) ;
#11210=CARTESIAN_POINT ( 'NONE',  ( 27.96989853965305528, -4.667028466753395222, -8.283357778048662468 ) ) ;
#11213=CARTESIAN_POINT ( 'NONE',  ( 30.01874226414561875, -2.539271660970221944, -6.861505862736159145 ) ) ;
#11214=VECTOR ( 'NONE', #16474, 1000.000000000000114 ) ;
#11225=CIRCLE ( 'NONE', #2576, 2.749999999999988454 ) ;
#11226=ORIENTED_EDGE ( 'NONE', *, *, #13488, .F. ) ;
#11230=AXIS2_PLACEMENT_3D ( 'NONE', #13009, #12917, #857 ) ;
#11233=ORIENTED_EDGE ( 'NONE', *, *, #17416, .T. ) ;
#11234=CARTESIAN_POINT ( 'NONE',  ( 28.73594040535616756, -2.066853418799292630, -5.783357778048658027 ) ) ;
#11235=DIRECTION ( 'NONE',  ( 0.000000000000000000, 0.000000000000000000, 1.000000000000000000 ) ) ;
#11245=ORIENTED_EDGE ( 'NONE', *, *, #14215, .F. ) ;
#11246=CARTESIAN_POINT ( 'NONE',  ( 32.32036211097666012, -1.624804527518282748, -5.783357778048663356 ) ) ;
#11250=ORIENTED_EDGE ( 'NONE', *, *, #14893, .T. ) ;
#11251=LINE ( 'NONE', #12914, #12806 ) ;
#11252=CARTESIAN_POINT ( 'NONE',  ( 25.74134610602432360, -2.427642893298174620, -5.783357778048658027 ) ) ;
#11254=CARTESIAN_POINT ( 'NONE',  ( 32.37175601071535880, -5.590505156207296267, -3.283357778048667797 ) ) ;
#11259=FACE_OUTER_BOUND ( 'NONE', #15717, .T. ) ;
#11268=DIRECTION ( 'NONE',  ( 0.9928203230275510771, 0.1196152422706614621, -0.000000000000000000 ) ) ;
#11269=CARTESIAN_POINT ( 'NONE',  ( 26.27749392786456895, -6.324743385012030927, -8.283357778048664244 ) ) ;
#11279=CARTESIAN_POINT ( 'NONE',  ( 27.02423718196931546, -4.780961985016209503, -3.283357778048664688 ) ) ;
#11282=DIRECTION ( 'NONE',  ( 0.000000000000000000, 0.000000000000000000, 1.000000000000000000 ) ) ;
#11286=VERTEX_POINT ( 'NONE', #14306 ) ;
#11295=EDGE_LOOP ( 'NONE', ( #5559, #6451, #3103, #9751 ) ) ;
#11296=CARTESIAN_POINT ( 'NONE',  ( 26.23609683341064525, -2.995005734021441768, -6.861505862736159145 ) ) ;
#11297=CARTESIAN_POINT ( 'NONE',  ( 32.96626681528915981, -4.065064760026301016, -5.783357778048663356 ) ) ;
#11302=LINE ( 'NONE', #15504, #1787 ) ;
#11307=CARTESIAN_POINT ( 'NONE',  ( 26.24565837299761739, -7.163851760794091916, -7.234565377303040279 ) ) ;
#11310=CARTESIAN_POINT ( 'NONE',  ( 29.62489513447700062, -6.348545659133139729, -6.861505862736166250 ) ) ;
#11312=DIRECTION ( 'NONE',  ( -0.1196152422706611984, 0.9928203230275510771, 0.000000000000000000 ) ) ;
#11322=ORIENTED_EDGE ( 'NONE', *, *, #1459, .T. ) ;
#11326=EDGE_LOOP ( 'NONE', ( #7766, #1053, #7251, #11793 ) ) ;
#11327=CARTESIAN_POINT ( 'NONE',  ( -25.01528890617809253, -10.29849948291661121, -14.47305271942837557 ) ) ;
#11329=CARTESIAN_POINT ( 'NONE',  ( 27.77288575766320378, -4.690764616287755651, -7.939653947423662039 ) ) ;
#11331=CARTESIAN_POINT ( 'NONE',  ( 30.78070346053490880, -6.209293581256383199, -4.705209693361168455 ) ) ;
#11333=DIRECTION ( 'NONE',  ( 0.9928203230275512992, 0.1196152422706614898, -0.000000000000000000 ) ) ;
#11335=ORIENTED_EDGE ( 'NONE', *, *, #2895, .T. ) ;
#11340=ORIENTED_EDGE ( 'NONE', *, *, #9289, .F. ) ;
#11344=EDGE_CURVE ( 'NONE', #9029, #5484, #8773, .T. ) ;
#11349=ORIENTED_EDGE ( 'NONE', *, *, #1459, .F. ) ;
#11350=CIRCLE ( 'NONE', #1251, 3.999999999999994671 ) ;
#11352=ORIENTED_EDGE ( 'NONE', *, *, #3204, .F. ) ;
#11354=ORIENTED_EDGE ( 'NONE', *, *, #12851, .F. ) ;
#11355=ADVANCED_FACE ( 'NONE', ( #15752 ), #17124, .F. ) ;
#11356=CARTESIAN_POINT ( 'NONE',  ( 33.59503905791412137, -1.808589744724287129, -4.533357778048659803 ) ) ;
#11357=CARTESIAN_POINT ( 'NONE',  ( 31.88017671309158274, -6.376637546091784792, -4.533357778048668685 ) ) ;
#11361=CARTESIAN_POINT ( 'NONE',  ( 29.65098506949083301, -2.583579140294649523, -4.705209693361160461 ) ) ;
#11364=CARTESIAN_POINT ( 'NONE',  ( 26.69778786461289855, -6.274106265784127778, -3.283357778048667797 ) ) ;
#11368=MANIFOLD_SOLID_BREP ( 'Thread1', #10420 ) ;
#11372=FILL_AREA_STYLE ('',( #12744 ) ) ;
#11376=ORIENTED_EDGE ( 'NONE', *, *, #5256, .T. ) ;
#11379=CARTESIAN_POINT ( 'NONE',  ( 15.92260893619738837, -28.39189527176317540, -6.000000000000000000 ) ) ;
#11381=CARTESIAN_POINT ( 'NONE',  ( 0.000000000000000000, 0.000000000000000000, -12.00000000000000000 ) ) ;
#11385=LINE ( 'NONE', #257, #10090 ) ;
#11404=DIRECTION ( 'NONE',  ( -0.1196152422706611984, 0.9928203230275510771, 0.000000000000000000 ) ) ;
#11409=CARTESIAN_POINT ( 'NONE',  ( 31.08270050955629671, -4.291997302367946077, -3.627061608673664672 ) ) ;
#11411=CARTESIAN_POINT ( 'NONE',  ( 32.41296236253129592, -1.951006642345344044, -4.533357778048659803 ) ) ;
#11412=CARTESIAN_POINT ( 'NONE',  ( 26.30054492745253825, -7.259773351106304951, -5.235134217867734030 ) ) ;
#11416=( BOUNDED_CURVE ( )  B_SPLINE_CURVE ( 2, ( #16984, #4538, #4897, #7638, #10423, #13339, #14435, #17458, #4988, #920, #6454, #17555, #11784, #2290, #7808, #14624, #559, #13068, #15985, #4803, #4721, #7719, #2019, #6078, #13161, #10593, #5074, #16162, #17363, #12976, #9083, #17267, #13244, #11609, #10329, #17172, #3645, #10245, #2205, #3370, #8901, #3551, #3725, #10516, #6356, #824, #11878, #16077, #15793, #9250, #15884, #11971, #9167, #14709, #6264, #14793, #7452, #7544, #6175, #651, #11699, #739, #3459, #8989, #14534, #2115, #12052, #3989, #11032, #17814, #14878, #4176, #5513, #15142, #9338, #10676, #7901, #9675, #12328, #2385, #16505, #17639, #6617, #7986, #16423, #1660, #5332, #14959, #9587, #10940, #2544, #12245, #15048, #1358, #5159, #16348, #13521, #2726, #16250, #10855, #8069, #1189, #16596, #1279, #13696, #6881, #4076, #2465, #8248, #13779, #12410, #13435, #1014, #17727, #8164, #6539, #3822, #1094, #5248, #12147, #10768, #6706, #3908, #9420, #13606, #9505, #2635, #6800, #17893, #5424, #9854, #91, #4520, #9948, #12870, #1636, #11296, #14049, #16684, #456, #4437, #11115, #7169, #15409, #8421, #176, #5598 ),
 .UNSPECIFIED., .F., .T. ) 
 B_SPLINE_CURVE_WITH_KNOTS ( ( 3, 2, 2, 2, 2, 2, 2, 2, 2, 2, 2, 2, 2, 2, 2, 2, 2, 2, 2, 2, 2, 2, 2, 2, 2, 2, 2, 2, 2, 2, 2, 2, 2, 2, 2, 2, 2, 2, 2, 2, 2, 2, 2, 2, 2, 2, 2, 2, 2, 2, 2, 2, 2, 2, 2, 2, 2, 2, 2, 2, 2, 2, 2, 2, 2, 2, 2, 2, 2, 2, 2, 2, 2, 3 ),
 ( 0.000000000000000000, 0.01322951968774666726, 0.02645903937549333451, 0.03968855906324000177, 0.05291807875098666902, 0.06614759843873332934, 0.07937711812648000353, 0.09260663781422667773, 0.1058361575019733380, 0.1190656771897200122, 0.1322951968774666587, 0.1455247165652133190, 0.1587542362529600071, 0.1719837559407066396, 0.1852132756284533555, 0.1984427953162000158, 0.2116723150039466761, 0.2249018346916933364, 0.2381313543794400245, 0.2513608740671866570, 0.2645903937549333174, 0.2778199134426800332, 0.2910494331304266380, 0.3042789528181733538, 0.3175084725059200141, 0.3307379921936667300, 0.3439675118814132793, 0.3571970315691599951, 0.3704265512569067109, 0.3836560709446533712, 0.3968855906324000316, 0.4101151103201466364, 0.4233446300078933522, 0.4365741496956400125, 0.4498036693833866728, 0.4630331890711333331, 0.4762627087588800490, 0.4894922284466267093, 0.5027217481343733141, 0.5159512678221199744, 0.5291807875098666347, 0.5424103071976132950, 0.5556398268853600664, 0.5688693465731067267, 0.5820988662608532760, 0.5953283859485999363, 0.6085579056363467076, 0.6217874253240932569, 0.6350169450118400283, 0.6482464646995866886, 0.6614759843873334599, 0.6747055040750800092, 0.6879350237628265585, 0.7011645434505734409, 0.7143940631383199902, 0.7276235828260666505, 0.7408531025138134218, 0.7540826222015599711, 0.7673121418893067425, 0.7805416615770532918, 0.7937711812648000631, 0.8070007009525467234, 0.8202302206402932727, 0.8334597403280399330, 0.8466892600157867044, 0.8599187797035333647, 0.8731482993912800250, 0.8863778190790266853, 0.8996073387667733456, 0.9128368584545200060, 0.9260663781422666663, 0.9392958978300133266, 0.9525254175177600979, 0.9555550897579921932 ),
 .UNSPECIFIED. ) 
 CURVE ( )  GEOMETRIC_REPRESENTATION_ITEM ( )  RATIONAL_B_SPLINE_CURVE ( ( 1.000000000000000000, 0.8660254037844387076, 1.000000000000000000, 0.8660254037844387076, 1.000000000000000000, 0.8660254037844387076, 1.000000000000000000, 0.8660254037844387076, 1.000000000000000000, 0.8660254037844387076, 1.000000000000000000, 0.8660254037844387076, 1.000000000000000000, 0.8660254037844387076, 1.000000000000000000, 0.8660254037844387076, 1.000000000000000000, 0.8660254037844387076, 1.000000000000000000, 0.8660254037844387076, 1.000000000000000000, 0.8660254037844387076, 1.000000000000000000, 0.8660254037844387076, 1.000000000000000000, 0.8660254037844387076, 1.000000000000000000, 0.8660254037844387076, 1.000000000000000000, 0.8660254037844387076, 1.000000000000000000, 0.8660254037844387076, 1.000000000000000000, 0.8660254037844387076, 1.000000000000000000, 0.8660254037844387076, 1.000000000000000000, 0.8660254037844387076, 1.000000000000000000, 0.8660254037844387076, 1.000000000000000000, 0.8660254037844387076, 1.000000000000000000, 0.8660254037844387076, 1.000000000000000000, 0.8660254037844387076, 1.000000000000000000, 0.8660254037844387076, 1.000000000000000000, 0.8660254037844387076, 1.000000000000000000, 0.8660254037844387076, 1.000000000000000000, 0.8660254037844387076, 1.000000000000000000, 0.8660254037844387076, 1.000000000000000000, 0.8660254037844387076, 1.000000000000000000, 0.8660254037844387076, 1.000000000000000000, 0.8660254037844387076, 1.000000000000000000, 0.8660254037844387076, 1.000000000000000000, 0.8660254037844387076, 1.000000000000000000, 0.8660254037844387076, 1.000000000000000000, 0.8660254037844387076, 1.000000000000000000, 0.8660254037844387076, 1.000000000000000000, 0.8660254037844387076, 1.000000000000000000, 0.8660254037844387076, 1.000000000000000000, 0.8660254037844387076, 1.000000000000000000, 0.8660254037844387076, 1.000000000000000000, 0.8660254037844387076, 1.000000000000000000, 0.8660254037844387076, 1.000000000000000000, 0.8660254037844387076, 1.000000000000000000, 0.8660254037844387076, 1.000000000000000000, 0.8660254037844387076, 1.000000000000000000, 0.8660254037844387076, 1.000000000000000000, 0.8660254037844387076, 1.000000000000000000, 0.8660254037844387076, 1.000000000000000000, 0.8660254037844387076, 1.000000000000000000, 0.8660254037844387076, 1.000000000000000000, 0.8660254037844387076, 1.000000000000000000, 0.8660254037844387076, 1.000000000000000000, 0.8660254037844387076, 1.000000000000000000, 0.8660254037844387076, 1.000000000000000000, 0.8660254037844387076, 1.000000000000000000, 0.8660254037844387076, 1.000000000000000000, 0.8660254037844387076, 1.000000000000000000, 0.8660254037844387076, 1.000000000000000000, 0.8660254037844387076, 1.000000000000000000, 0.8660254037844387076, 1.000000000000000000, 0.8660254037844387076, 1.000000000000000000, 0.8660254037844387076, 1.000000000000000000, 0.8660254037844387076, 1.000000000000000000, 0.8660254037844387076, 1.000000000000000000, 0.8660254037844387076, 1.000000000000000000, 0.8660254037844387076, 1.000000000000000000, 0.8660254037844387076, 1.000000000000000000, 0.8660254037844387076, 1.000000000000000000, 0.8660254037844387076, 1.000000000000000000, 0.8660254037844387076, 1.000000000000000000, 0.8660254037844387076, 1.000000000000000000, 0.8660254037844387076, 1.000000000000000000, 0.9693186809021840933, 0.9526899265169710418 ) ) 
 REPRESENTATION_ITEM ( '' )  );
#11418=VERTEX_POINT ( 'NONE', #7758 ) ;
#11419=VERTEX_POINT ( 'NONE', #13290 ) ;
#11423=CARTESIAN_POINT ( 'NONE',  ( -19.73861724507318627, -10.88265359452670644, -15.55811197012310743 ) ) ;
#11424=ORIENTED_EDGE ( 'NONE', *, *, #11842, .F. ) ;
#11425=CARTESIAN_POINT ( 'NONE',  ( 27.88665588685489993, -3.423116496867954162, -3.627061608673662008 ) ) ;
#11428=CARTESIAN_POINT ( 'NONE',  ( 32.16857880351144416, -6.669052543620333395, -5.783357778048668685 ) ) ;
#11429=VERTEX_POINT ( 'NONE', #6834 ) ;
#11431=CARTESIAN_POINT ( 'NONE',  ( 32.87199790123699472, -1.558343308739095656, -5.783357778048663356 ) ) ;
#11439=PLANE ( 'NONE',  #2021 ) ;
#11443=CARTESIAN_POINT ( 'NONE',  ( 25.11802603177690330, -19.03270077640483038, -0.5379818257722508434 ) ) ;
#11444=CARTESIAN_POINT ( 'NONE',  ( 27.17934203385504333, -30.00000000000000355, 0.000000000000000000 ) ) ;
#11447=CARTESIAN_POINT ( 'NONE',  ( 26.66770885555339987, -3.370103022578743612, -8.283357778048660691 ) ) ;
#11448=CARTESIAN_POINT ( 'NONE',  ( 33.52375369703867847, -2.544085015380856518, -8.283357778048658915 ) ) ;
#11452=DIRECTION ( 'NONE',  ( 0.000000000000000000, 0.000000000000000000, 1.000000000000000000 ) ) ;
#11453=CARTESIAN_POINT ( 'NONE',  ( 29.77797860222238313, -3.195249460342344250, -3.627061608673662008 ) ) ;
#11455=DIRECTION ( 'NONE',  ( 0.9928203230275512992, 0.1196152422706614898, -0.000000000000000000 ) ) ;
#11475=VERTEX_POINT ( 'NONE', #12283 ) ;
#11480=EDGE_CURVE ( 'NONE', #11111, #17553, #7941, .T. ) ;
#11485=DIRECTION ( 'NONE',  ( -0.3420201433256631618, 0.000000000000000000, 0.9396926207859104263 ) ) ;
#11488=CARTESIAN_POINT ( 'NONE',  ( -29.04317620846695647, -17.86624673319742840, -13.43120144060744003 ) ) ;
#11490=CARTESIAN_POINT ( 'NONE',  ( 31.97277696464621854, -6.702839660918840536, -5.783357778048663356 ) ) ;
#11496=CARTESIAN_POINT ( 'NONE',  ( 26.03917326857634151, -4.899642733102906433, -3.627061608673664672 ) ) ;
#11498=CARTESIAN_POINT ( 'NONE',  ( 33.23365877489121090, -6.550928303235100891, -5.783357778048663356 ) ) ;
#11511=AXIS2_PLACEMENT_3D ( 'NONE', #11297, #14329, #4259 ) ;
#11512=CARTESIAN_POINT ( 'NONE',  ( 26.19678349485696955, -4.880653813392439311, -3.627061608673664672 ) ) ;
#11514=CARTESIAN_POINT ( 'NONE',  ( 26.82722439997946395, -4.804698134550569044, -3.627061608673664672 ) ) ;
#11515=EDGE_CURVE ( 'NONE', #13858, #4517, #1400, .T. ) ;
#11516=CARTESIAN_POINT ( 'NONE',  ( 27.71165237056504438, -5.952083095804076684, -7.939653947423664704 ) ) ;
#11517=ORIENTED_EDGE ( 'NONE', *, *, #1141, .T. ) ;
#11518=DIRECTION ( 'NONE',  ( 0.9928203230275512992, 0.1196152422706614898, -0.000000000000000000 ) ) ;
#11539=CARTESIAN_POINT ( 'NONE',  ( 33.09223089549517738, -4.049888575955752579, -8.283357778048662468 ) ) ;
#11544=DIRECTION ( 'NONE',  ( 0.9928203230275510771, 0.1196152422706614621, -0.000000000000000000 ) ) ;
#11546=DIRECTION ( 'NONE',  ( -0.1196152422706611984, 0.9928203230275510771, 0.000000000000000000 ) ) ;
#11548=AXIS2_PLACEMENT_3D ( 'NONE', #14101, #1687, #7222 ) ;
#11550=ORIENTED_EDGE ( 'NONE', *, *, #1899, .T. ) ;
#11557=CARTESIAN_POINT ( 'NONE',  ( 25.71748644841968456, -2.420320648352051851, -5.783357778048663356 ) ) ;
#11559=ADVANCED_FACE ( 'NONE', ( #6283 ), #13264, .F. ) ;
#11560=VERTEX_POINT ( 'NONE', #12995 ) ;
#11561=LINE ( 'NONE', #17129, #17534 ) ;
#11566=CARTESIAN_POINT ( 'NONE',  ( 26.66018910156667232, -2.644102211984857842, -4.533357778048659803 ) ) ;
#11573=FACE_OUTER_BOUND ( 'NONE', #8617, .T. ) ;
#11577=ORIENTED_EDGE ( 'NONE', *, *, #13189, .F. ) ;
#11580=CARTESIAN_POINT ( 'NONE',  ( 20.00000000000000355, 7.999999999999996447, -6.000000000000000000 ) ) ;
#11582=CARTESIAN_POINT ( 'NONE',  ( -8.876997858717690093, 16.38553564496311310, -16.83638096351226920 ) ) ;
#11584=CARTESIAN_POINT ( 'NONE',  ( -17.70832741558421830, -19.55032950225749389, -15.89323616604937328 ) ) ;
#11587=CARTESIAN_POINT ( 'NONE',  ( -19.43845002722867221, 2.988003976273734708, 0.000000000000000000 ) ) ;
#11589=CARTESIAN_POINT ( 'NONE',  ( 28.99436501219896201, -4.543600488427916417, -3.283357778048664688 ) ) ;
#11590=LINE ( 'NONE', #4707, #7310 ) ;
#11591=CARTESIAN_POINT ( 'NONE',  ( 26.07857582428556853, -4.894895503279006022, -8.283357778048662468 ) ) ;
#11594=CIRCLE ( 'NONE', #13057, 5.000000000000000000 ) ;
#11596=CARTESIAN_POINT ( 'NONE',  ( 28.12741954877813555, -2.767138697495831856, -6.861505862736159145 ) ) ;
#11599=CARTESIAN_POINT ( 'NONE',  ( 26.17715024865825768, -6.235583268514400146, -3.900143082538624739 ) ) ;
#11604=ORIENTED_EDGE ( 'NONE', *, *, #13283, .T. ) ;
#11606=AXIS2_PLACEMENT_3D ( 'NONE', #14437, #3287, #13246 ) ;
#11607=CIRCLE ( 'NONE', #9297, 5.000000000000000000 ) ;
#11609=CARTESIAN_POINT ( 'NONE',  ( 32.16857880351144416, -6.669052543620333395, -5.783357778048668685 ) ) ;
#11613=VERTEX_POINT ( 'NONE', #3579 ) ;
#11614=CARTESIAN_POINT ( 'NONE',  ( 27.15566825608056689, -6.646038734597135011, -4.705209693361169343 ) ) ;
#11615=CARTESIAN_POINT ( 'NONE',  ( 25.74134610602432360, -2.427642893298174620, -5.783357778048658027 ) ) ;
#11617=CARTESIAN_POINT ( 'NONE',  ( 26.23609683341064525, -2.995005734021441768, -6.861505862736159145 ) ) ;
#11619=CARTESIAN_POINT ( 'NONE',  ( 33.01342578063301403, -4.059383036018435753, -8.283357778048662468 ) ) ;
#11627=VECTOR ( 'NONE', #14262, 1000.000000000000227 ) ;
#11629=VERTEX_POINT ( 'NONE', #10534 ) ;
#11631=DIRECTION ( 'NONE',  ( -1.000000000000000000, 0.000000000000000000, 0.000000000000000000 ) ) ;
#11637=LINE ( 'NONE', #16102, #4384 ) ;
#11641=CARTESIAN_POINT ( 'NONE',  ( 29.75233713454258933, -1.544652646670201523, -5.783357778048658027 ) ) ;
#11647=CARTESIAN_POINT ( 'NONE',  ( 31.66250999073069750, -5.675955295111850596, -3.283357778048667797 ) ) ;
#11653=ORIENTED_EDGE ( 'NONE', *, *, #11055, .F. ) ;
#11657=EDGE_CURVE ( 'NONE', #1954, #14246, #9540, .T. ) ;
#11663=CARTESIAN_POINT ( 'NONE',  ( 33.32855701603872234, -2.140504347050403045, -6.861505862736158257 ) ) ;
#11665=CARTESIAN_POINT ( 'NONE',  ( 28.75424055680402802, -6.753251120556833520, -7.033357778048666908 ) ) ;
#11669=EDGE_CURVE ( 'NONE', #1954, #11901, #13362, .T. ) ;
#11679=CARTESIAN_POINT ( 'NONE',  ( -12.26589791205140045, 14.78806204439702121, -16.57179146834700845 ) ) ;
#11680=CARTESIAN_POINT ( 'NONE',  ( -16.75000000000000000, -16.63059030033399921, -16.03574476417184869 ) ) ;
#11682=CARTESIAN_POINT ( 'NONE',  ( 33.18226487515251932, -2.585227674546096477, -3.283357778048662023 ) ) ;
#11685=CARTESIAN_POINT ( 'NONE',  ( 23.00000000000000000, -16.21813761408365195, -13.00000000000000178 ) ) ;
#11689=EDGE_CURVE ( 'NONE', #5257, #1336, #1220, .T. ) ;
#11690=CARTESIAN_POINT ( 'NONE',  ( 25.60565592828815440, -3.070961412863312034, -6.861505862736159145 ) ) ;
#11697=CARTESIAN_POINT ( 'NONE',  ( 29.40036258452792950, -7.012764792547963033, -6.453230759126474148 ) ) ;
#11699=CARTESIAN_POINT ( 'NONE',  ( 30.45225960443380231, -4.367952981209816343, -3.627061608673664672 ) ) ;
#11701=DIRECTION ( 'NONE',  ( -0.000000000000000000, -0.000000000000000000, -1.000000000000000000 ) ) ;
#11702=CARTESIAN_POINT ( 'NONE',  ( -35.19141017012124451, -14.17387298022714148, -11.46934516270795079 ) ) ;
#11705=CARTESIAN_POINT ( 'NONE',  ( 27.62849893492243325, -6.589071975465733644, -4.705209693361168455 ) ) ;
#11707=CARTESIAN_POINT ( 'NONE',  ( 27.33945763453056088, -4.742984145595265488, -8.283357778048662468 ) ) ;
#11710=ADVANCED_FACE ( 'NONE', ( #10964 ), #3843, .F. ) ;
#11713=EDGE_CURVE ( 'NONE', #11286, #4257, #17171, .T. ) ;
#11718=VERTEX_POINT ( 'NONE', #14979 ) ;
#11722=CARTESIAN_POINT ( 'NONE',  ( 15.92260893619738837, -28.39189527176317540, -6.000000000000000000 ) ) ;
#11725=CARTESIAN_POINT ( 'NONE',  ( 28.55903157092087952, -3.142235986053133256, -8.283357778048658915 ) ) ;
#11727=FACE_BOUND ( 'NONE', #5984, .T. ) ;
#11729=EDGE_CURVE ( 'NONE', #10591, #6646, #878, .T. ) ;
#11730=LINE ( 'NONE', #5025, #17785 ) ;
#11733=ORIENTED_EDGE ( 'NONE', *, *, #17570, .F. ) ;
#11736=VERTEX_POINT ( 'NONE', #9613 ) ;
#11742=B_SPLINE_CURVE_WITH_KNOTS ( 'NONE', 3,
 ( #15315, #8423, #13959, #11582, #12773, #17151, #6155, #15587, #11679, #7524, #4699, #8604, #17249, #15501, #1823, #10227 ),
 .UNSPECIFIED., .F., .F.,
 ( 4, 2, 2, 2, 2, 2, 2, 4 ),
 ( 0.000000000000000000, 0.004966453901722449327, 0.007449680852583671388, 0.008691294328014282852, 0.009932907803444893449, 0.01489936170516735839, 0.01738258865602858652, 0.01986581560688981465 ),
 .UNSPECIFIED. ) ;
#11747=CARTESIAN_POINT ( 'NONE',  ( 32.81641299864316608, -4.083119185552795294, -7.939653947423662039 ) ) ;
#11759=ORIENTED_EDGE ( 'NONE', *, *, #3542, .F. ) ;
#11766=CARTESIAN_POINT ( 'NONE',  ( -21.42418507870700850, -22.26964835135415655, -15.24537475165205791 ) ) ;
#11768=CARTESIAN_POINT ( 'NONE',  ( 32.97895737133300287, -1.545456804875373402, -5.113484796970854340 ) ) ;
#11775=CARTESIAN_POINT ( 'NONE',  ( 27.30005507882132676, -4.747731375419166788, -3.627061608673664672 ) ) ;
#11776=ADVANCED_FACE ( 'NONE', ( #1299 ), #6638, .F. ) ;
#11779=CARTESIAN_POINT ( 'NONE',  ( 28.30694982360322953, -3.372479377640031473, -7.939653947423660263 ) ) ;
#11781=DIRECTION ( 'NONE',  ( 0.9928203230275510771, 0.1196152422706614621, -0.000000000000000000 ) ) ;
#11782=ORIENTED_EDGE ( 'NONE', *, *, #12527, .F. ) ;
#11784=CARTESIAN_POINT ( 'NONE',  ( 32.97402322492378346, -4.064130265842336165, -3.627061608673664672 ) ) ;
#11792=CARTESIAN_POINT ( 'NONE',  ( 30.44283453230164227, -2.188368138933637574, -4.533357778048659803 ) ) ;
#11793=ORIENTED_EDGE ( 'NONE', *, *, #14556, .T. ) ;
#11794=CARTESIAN_POINT ( 'NONE',  ( 26.86653773853314320, -2.919050055179571945, -6.861505862736159145 ) ) ;
#11795=EDGE_CURVE ( 'NONE', #15536, #16822, #16817, .T. ) ;
#11796=CARTESIAN_POINT ( 'NONE',  ( 32.83754810739938534, -9.116730809865837060, -15.78335777804866424 ) ) ;
#11797=CARTESIAN_POINT ( 'NONE',  ( 33.64386668575551198, -3.983427357176565486, -8.283357778048662468 ) ) ;
#11803=CARTESIAN_POINT ( 'NONE',  ( -15.92260893619738837, -28.39189527176317540, -6.000000000000000000 ) ) ;
#11804=DIRECTION ( 'NONE',  ( 0.1113444980252557837, -0.9937818688019538493, 0.000000000000000000 ) ) ;
#11805=VECTOR ( 'NONE', #1928, 1000.000000000000000 ) ;
#11806=DIRECTION ( 'NONE',  ( 0.000000000000000000, 0.000000000000000000, -1.000000000000000000 ) ) ;
#11807=VERTEX_POINT ( 'NONE', #13799 ) ;
#11808=CARTESIAN_POINT ( 'NONE',  ( -7.499998387031003411, -20.49508120620799900, -12.00000000000000000 ) ) ;
#11812=CARTESIAN_POINT ( 'NONE',  ( 32.80318959510331212, -2.203800746085299522, -4.705209693361160461 ) ) ;
#11815=CARTESIAN_POINT ( 'NONE',  ( 30.72436838703367812, -6.515889623968540434, -7.033357778048666908 ) ) ;
#11818=CARTESIAN_POINT ( 'NONE',  ( 26.31556265977298992, -7.384422263489805793, -5.783357778048663356 ) ) ;
#11821=VECTOR ( 'NONE', #1704, 1000.000000000000227 ) ;
#11822=CARTESIAN_POINT ( 'NONE',  ( 32.52441275490655670, -6.636378442139655220, -5.783357778048663356 ) ) ;
#11834=CARTESIAN_POINT ( 'NONE',  ( -15.92260893619738837, -28.39189527176317540, -6.000000000000000000 ) ) ;
#11835=EDGE_CURVE ( 'NONE', #3411, #7377, #17830, .T. ) ;
#11838=CARTESIAN_POINT ( 'NONE',  ( 33.56062403295735663, -2.739515387291124426, -3.627061608673662008 ) ) ;
#11842=EDGE_CURVE ( 'NONE', #12386, #227, #11138, .T. ) ;
#11858=ADVANCED_FACE ( 'NONE', ( #14158 ), #393, .F. ) ;
#11859=FACE_OUTER_BOUND ( 'NONE', #736, .T. ) ;
#11861=CARTESIAN_POINT ( 'NONE',  ( 31.37049041475757605, -6.775403295959669947, -6.453230759126470595 ) ) ;
#11862=CARTESIAN_POINT ( 'NONE',  ( 30.35023428074701002, -1.862166024106576057, -5.783357778048664244 ) ) ;
#11867=ORIENTED_EDGE ( 'NONE', *, *, #8641, .F. ) ;
#11868=CARTESIAN_POINT ( 'NONE',  ( 27.49697864365563760, -2.843094376337701679, -6.861505862736159145 ) ) ;
#11871=CIRCLE ( 'NONE', #4635, 6.249999999999996447 ) ;
#11873=ADVANCED_FACE ( 'NONE', ( #5621 ), #4370, .T. ) ;
#11877=CARTESIAN_POINT ( 'NONE',  ( 29.06119811526816576, -2.017469425591354337, -6.453230759126464378 ) ) ;
#11878=CARTESIAN_POINT ( 'NONE',  ( 31.41114436565740320, -6.133337902414513820, -4.705209693361168455 ) ) ;
#11884=AXIS2_PLACEMENT_3D ( 'NONE', #12863, #3251, #5680 ) ;
#11886=CARTESIAN_POINT ( 'NONE',  ( 31.70371634254663817, -2.036456781249897485, -4.533357778048659803 ) ) ;
#11888=CARTESIAN_POINT ( 'NONE',  ( 26.03917326857634151, -4.899642733102906433, -3.627061608673664672 ) ) ;
#11890=CARTESIAN_POINT ( 'NONE',  ( 32.51061761821408425, -6.300681867249914525, -4.533357778048668685 ) ) ;
#11893=EDGE_CURVE ( 'NONE', #11629, #15856, #5898, .T. ) ;
#11897=AXIS2_PLACEMENT_3D ( 'NONE', #14692, #7703, #10580 ) ;
#11901=VERTEX_POINT ( 'NONE', #8451 ) ;
#11903=DIRECTION ( 'NONE',  ( -0.000000000000000000, -0.000000000000000000, -1.000000000000000000 ) ) ;
#11904=CARTESIAN_POINT ( 'NONE',  ( 32.50119254608192421, -4.121097024973739309, -3.627061608673664672 ) ) ;
#11906=CARTESIAN_POINT ( 'NONE',  ( 29.12189622942009493, -1.620608325512071568, -5.783357778048658027 ) ) ;
#11912=CARTESIAN_POINT ( 'NONE',  ( 29.25000000000000000, -16.63088773646508756, -13.37255996287878013 ) ) ;
#11914=ORIENTED_EDGE ( 'NONE', *, *, #1761, .F. ) ;
#11915=EDGE_CURVE ( 'NONE', #5268, #7494, #10061, .T. ) ;
#11929=CARTESIAN_POINT ( 'NONE',  ( 32.18597209352066812, -4.159074864394664672, -7.939653947423662039 ) ) ;
#11931=CARTESIAN_POINT ( 'NONE',  ( 28.72045243349238675, -6.030415129707233035, -8.283357778048664244 ) ) ;
#11933=DIRECTION ( 'NONE',  ( -0.1196152422706611984, 0.9928203230275510771, 0.000000000000000000 ) ) ;
#11935=DIRECTION ( 'NONE',  ( 1.000000000000000000, 0.000000000000000000, 0.000000000000000000 ) ) ;
#11936=CARTESIAN_POINT ( 'NONE',  ( -25.74999999999998934, -16.21813761408365195, -13.00000000000000355 ) ) ;
#11940=( BOUNDED_CURVE ( )  B_SPLINE_CURVE ( 2, ( #6158, #11682, #2274, #11768, #8970 ),
 .UNSPECIFIED., .F., .T. ) 
 B_SPLINE_CURVE_WITH_KNOTS ( ( 3, 2, 3 ),
 ( 0.000000000000000000, 0.01282051282051282007, 0.01923076923076924918 ),
 .UNSPECIFIED. ) 
 CURVE ( )  GEOMETRIC_REPRESENTATION_ITEM ( )  RATIONAL_B_SPLINE_CURVE ( ( 1.000000000000000000, 0.8660254037844387076, 1.000000000000000000, 0.9330127018922191873, 0.9330127018922194093 ) ) 
 REPRESENTATION_ITEM ( '' )  );
#11944=ORIENTED_EDGE ( 'NONE', *, *, #12752, .T. ) ;
#11950=EDGE_CURVE ( 'NONE', #13310, #1298, #15968, .T. ) ;
#11960=CARTESIAN_POINT ( 'NONE',  ( 25.88156304229571703, -4.918631652813365562, -7.939653947423662039 ) ) ;
#11962=CARTESIAN_POINT ( 'NONE',  ( 32.06767520579373354, -2.292415704734142690, -6.861505862736158257 ) ) ;
#11970=FACE_OUTER_BOUND ( 'NONE', #1331, .T. ) ;
#11971=CARTESIAN_POINT ( 'NONE',  ( 30.62726312072365431, -1.838986382273682718, -5.783357778048658915 ) ) ;
#11979=CARTESIAN_POINT ( 'NONE',  ( 32.69820532807177216, -4.097360875439379768, -3.283357778048664688 ) ) ;
#11981=CARTESIAN_POINT ( 'NONE',  ( 32.56242593318007295, -2.859778545457410281, -7.939653947423660263 ) ) ;
#11989=ORIENTED_EDGE ( 'NONE', *, *, #5209, .T. ) ;
#11991=CARTESIAN_POINT ( 'NONE',  ( -27.17934203385504333, -30.00000000000000355, -12.00000000000000000 ) ) ;
#11993=PRODUCT ( 'Caliper Body Half', 'Caliper Body Half', '', ( #5653 ) ) ;
#11996=EDGE_CURVE ( 'NONE', #5005, #16638, #2735, .T. ) ;
#11999=CARTESIAN_POINT ( 'NONE',  ( 27.92859066579839222, -3.218191664895003967, -8.283357778048658915 ) ) ;
#12016=DIRECTION ( 'NONE',  ( -0.000000000000000000, -0.000000000000000000, -1.000000000000000000 ) ) ;
#12017=CARTESIAN_POINT ( 'NONE',  ( 31.54230778485832332, -2.355712103769039611, -4.705209693361160461 ) ) ;
#12021=DIRECTION ( 'NONE',  ( -1.000000000000000000, 0.000000000000000000, 0.000000000000000000 ) ) ;
#12022=CARTESIAN_POINT ( 'NONE',  ( 32.32036211097666012, -1.624804527518282748, -5.783357778048663356 ) ) ;
#12028=ORIENTED_EDGE ( 'NONE', *, *, #5016, .T. ) ;
#12039=EDGE_CURVE ( 'NONE', #2012, #8375, #13054, .T. ) ;
#12040=DIRECTION ( 'NONE',  ( 1.000000000000000000, 0.000000000000000000, 0.000000000000000000 ) ) ;
#12041=CARTESIAN_POINT ( 'NONE',  ( 26.39823381822651882, -6.110324093391315436, -3.627061608673668225 ) ) ;
#12044=CARTESIAN_POINT ( 'NONE',  ( 30.91186687973582536, -2.431667782610909434, -4.705209693361160461 ) ) ;
#12047=EDGE_CURVE ( 'NONE', #13311, #10072, #11003, .T. ) ;
#12048=CARTESIAN_POINT ( 'NONE',  ( 35.62429925076629189, -17.76690233603958546, -10.53798182577225084 ) ) ;
#12052=CARTESIAN_POINT ( 'NONE',  ( 30.13703915187255689, -4.405930820630744371, -7.939653947423662039 ) ) ;
#12055=CYLINDRICAL_SURFACE ( 'NONE', #15649, 2.499999999999999112 ) ;
#12058=CARTESIAN_POINT ( 'NONE',  ( 30.93441382992541477, -1.402235749049144609, -5.783357778048658027 ) ) ;
#12060=CARTESIAN_POINT ( 'NONE',  ( 33.38562051666750818, -5.268481986227246061, -7.939653947423664704 ) ) ;
#12061=EDGE_CURVE ( 'NONE', #496, #2012, #17175, .T. ) ;
#12068=EDGE_CURVE ( 'NONE', #8375, #16681, #7277, .T. ) ;
#12075=CARTESIAN_POINT ( 'NONE',  ( 27.82847066025702887, -2.165988739474055791, -5.783357778048658027 ) ) ;
#12077=CARTESIAN_POINT ( 'NONE',  ( 32.95662993491456660, -6.574107945067995118, -5.783357778048669573 ) ) ;
#12080=CARTESIAN_POINT ( 'NONE',  ( 25.47811240618384687, -2.786519109605914757, -4.533357778048659803 ) ) ;
#12083=CARTESIAN_POINT ( 'NONE',  ( 9.099998387031005720, -19.29508120620799971, -16.81964500401478091 ) ) ;
#12088=( BOUNDED_CURVE ( )  B_SPLINE_CURVE ( 2, ( #17904, #8342, #12257, #4092, #11047, #5526, #6990, #2903, #16435 ),
 .UNSPECIFIED., .F., .T. ) 
 B_SPLINE_CURVE_WITH_KNOTS ( ( 3, 2, 2, 2, 3 ),
 ( 0.6346153846153846922, 0.6410256410256410797, 0.6538461538461538547, 0.6666666666666666297, 0.6730769230769231282 ),
 .UNSPECIFIED. ) 
 CURVE ( )  GEOMETRIC_REPRESENTATION_ITEM ( )  RATIONAL_B_SPLINE_CURVE ( ( 0.9330127018922192983, 0.9330127018922198534, 1.000000000000000000, 0.8660254037844387076, 1.000000000000000000, 0.8660254037844387076, 1.000000000000000000, 0.9330127018922187432, 0.9330127018922192983 ) ) 
 REPRESENTATION_ITEM ( '' )  );
#12091=ORIENTED_EDGE ( 'NONE', *, *, #6673, .T. ) ;
#12095=ORIENTED_EDGE ( 'NONE', *, *, #10851, .F. ) ;
#12102=CARTESIAN_POINT ( 'NONE',  ( 30.91186687973582536, -2.431667782610909434, -4.705209693361160461 ) ) ;
#12103=ORIENTED_EDGE ( 'NONE', *, *, #8527, .T. ) ;
#12105=CARTESIAN_POINT ( 'NONE',  ( 30.41656616297672500, -2.191532958677927745, -7.033357778048658027 ) ) ;
#12107=DIRECTION ( 'NONE',  ( -1.000000000000000000, 0.000000000000000000, -0.000000000000000000 ) ) ;
#12109=DIRECTION ( 'NONE',  ( 0.000000000000000000, 1.000000000000000000, 0.000000000000000000 ) ) ;
#12110=CARTESIAN_POINT ( 'NONE',  ( -45.50000000000000000, -19.03270077640483038, -5.537981825772250843 ) ) ;
#12116=ORIENTED_EDGE ( 'NONE', *, *, #15055, .T. ) ;
#12117=EDGE_CURVE ( 'NONE', #15522, #29, #10678, .T. ) ;
#12120=VECTOR ( 'NONE', #16666, 1000.000000000000114 ) ;
#12125=EDGE_LOOP ( 'NONE', ( #12408, #3864, #17177, #17372 ) ) ;
#12134=CYLINDRICAL_SURFACE ( 'NONE', #10758, 2.499999999999999112 ) ;
#12135=CARTESIAN_POINT ( 'NONE',  ( 26.63030083514515312, -6.709335133632020387, -6.861505862736167138 ) ) ;
#12136=PLANE ( 'NONE',  #5576 ) ;
#12138=CARTESIAN_POINT ( 'NONE',  ( 30.81132015408399027, -5.578634341498224458, -3.627061608673668225 ) ) ;
#12140=FACE_OUTER_BOUND ( 'NONE', #14259, .T. ) ;
#12141=DIRECTION ( 'NONE',  ( -0.000000000000000000, -0.000000000000000000, -1.000000000000000000 ) ) ;
#12142=AXIS2_PLACEMENT_3D ( 'NONE', #7602, #9305, #11933 ) ;
#12145=VERTEX_POINT ( 'NONE', #1191 ) ;
#12147=CARTESIAN_POINT ( 'NONE',  ( 27.50150540219088313, -5.977401655418041138, -3.627061608673667781 ) ) ;
#12152=CARTESIAN_POINT ( 'NONE',  ( 30.40162818048570514, -5.827866652795590241, -3.283357778048667797 ) ) ;
#12153=ORIENTED_EDGE ( 'NONE', *, *, #12382, .T. ) ;
#12155=DIRECTION ( 'NONE',  ( -1.000000000000000000, 0.000000000000000000, 0.000000000000000000 ) ) ;
#12162=AXIS2_PLACEMENT_3D ( 'NONE', #1952, #10352, #13180 ) ;
#12165=ORIENTED_EDGE ( 'NONE', *, *, #3067, .F. ) ;
#12169=SURFACE_STYLE_FILL_AREA ( #1119 ) ;
#12171=VECTOR ( 'NONE', #17643, 1000.000000000000000 ) ;
#12172=CARTESIAN_POINT ( 'NONE',  ( 32.70264286945147347, -5.350767304972614546, -3.627061608673668225 ) ) ;
#12175=CARTESIAN_POINT ( 'NONE',  ( 32.64557936882268052, -2.222789665795767089, -4.705209693361161349 ) ) ;
#12176=VECTOR ( 'NONE', #12330, 1000.000000000000114 ) ;
#12183=ORIENTED_EDGE ( 'NONE', *, *, #1716, .T. ) ;
#12189=ORIENTED_EDGE ( 'NONE', *, *, #17178, .F. ) ;
#12191=DIRECTION ( 'NONE',  ( 1.000000000000000000, 0.000000000000000000, 0.000000000000000000 ) ) ;
#12196=CARTESIAN_POINT ( 'NONE',  ( 29.03376756790819613, -4.538853258604016006, -7.939653947423662039 ) ) ;
#12200=CARTESIAN_POINT ( 'NONE',  ( -2.016448651773435938E-27, -20.49999999999999645, -13.00000000000000178 ) ) ;
#12221=CARTESIAN_POINT ( 'NONE',  ( 27.55969062878875064, -7.234529412811931515, -5.783357778048668685 ) ) ;
#12228=CARTESIAN_POINT ( 'NONE',  ( 18.06432791129289939, -12.37828432491873443, -15.83774382844986484 ) ) ;
#12232=AXIS2_PLACEMENT_3D ( 'NONE', #15238, #6992, #16696 ) ;
#12233=( BOUNDED_CURVE ( )  B_SPLINE_CURVE ( 2, ( #5907, #10343, #2128, #662, #11707, #7650, #6276, #6185, #14547 ),
 .UNSPECIFIED., .F., .F. ) 
 B_SPLINE_CURVE_WITH_KNOTS ( ( 3, 2, 2, 2, 3 ),
 ( 0.7884615384615384359, 0.7948717948717948234, 0.8076923076923077094, 0.8205128205128204844, 0.8269230769230769829 ),
 .UNSPECIFIED. ) 
 CURVE ( )  GEOMETRIC_REPRESENTATION_ITEM ( )  RATIONAL_B_SPLINE_CURVE ( ( 0.9330127018922194093, 0.9330127018922194093, 1.000000000000000000, 0.8660254037844387076, 1.000000000000000000, 0.8660254037844387076, 1.000000000000000000, 0.9330127018922187432, 0.9330127018922192983 ) ) 
 REPRESENTATION_ITEM ( '' )  );
#12234=CARTESIAN_POINT ( 'NONE',  ( 32.19919549706052209, -6.038393303862174655, -4.705209693361169343 ) ) ;
#12237=CARTESIAN_POINT ( 'NONE',  ( 50.00000000000000000, -16.03270077640482683, -5.537981825772250843 ) ) ;
#12239=AXIS2_PLACEMENT_3D ( 'NONE', #3057, #1614, #1890 ) ;
#12245=CARTESIAN_POINT ( 'NONE',  ( 28.97253418081003673, -5.800171738120336151, -7.939653947423662927 ) ) ;
#12248=CYLINDRICAL_SURFACE ( 'NONE', #42, 2.000000000000001776 ) ;
#12254=CARTESIAN_POINT ( 'NONE',  ( 27.18555652250208610, -2.580805812949960920, -7.033357778048658027 ) ) ;
#12256=CARTESIAN_POINT ( 'NONE',  ( 32.14665875496697822, -6.044722943765660439, -6.861505862736166250 ) ) ;
#12257=CARTESIAN_POINT ( 'NONE',  ( 27.89480254248674740, -2.495355674045408367, -7.033357778048658027 ) ) ;
#12263=B_SPLINE_CURVE_WITH_KNOTS ( 'NONE', 3,
 ( #933, #1026, #6469, #15897, #7911, #4910, #17567, #7730, #13532, #6630, #10438, #9094, #15998, #10608 ),
 .UNSPECIFIED., .F., .F.,
 ( 4, 2, 2, 2, 2, 2, 4 ),
 ( 0.000000000000000000, 0.004968481363098090076, 0.007452722044647132511, 0.009936962726196174947, 0.01490544408929426155, 0.01738968477084330486, 0.01987392545239234642 ),
 .UNSPECIFIED. ) ;
#12266=CARTESIAN_POINT ( 'NONE',  ( 3.538288549924106796, -15.34800872113743431, -16.99955934415557479 ) ) ;
#12268=EDGE_LOOP ( 'NONE', ( #4994, #1353, #15242, #3054 ) ) ;
#12270=CARTESIAN_POINT ( 'NONE',  ( 29.17398450417959310, -7.029842018119214941, -5.783357778048669573 ) ) ;
#12274=CARTESIAN_POINT ( 'NONE',  ( 33.14902674121363901, -1.535163666906202318, -5.783357778048658027 ) ) ;
#12278=ORIENTED_EDGE ( 'NONE', *, *, #13895, .F. ) ;
#12279=CARTESIAN_POINT ( 'NONE',  ( 28.40369292566375492, -19.36532336263649512, -13.60921607110385523 ) ) ;
#12283=CARTESIAN_POINT ( 'NONE',  ( 19.43845002722867221, 2.988003976273734263, 0.000000000000000000 ) ) ;
#12289=ORIENTED_EDGE ( 'NONE', *, *, #6655, .F. ) ;
#12291=CARTESIAN_POINT ( 'NONE',  ( 29.67743187657054449, -6.342216019229654833, -4.705209693361169343 ) ) ;
#12293=ADVANCED_FACE ( 'NONE', ( #13610 ), #12248, .T. ) ;
#12304=ORIENTED_EDGE ( 'NONE', *, *, #11893, .F. ) ;
#12317=CARTESIAN_POINT ( 'NONE',  ( 26.79770707206266778, -11.23794579741151090, -14.03572743982056181 ) ) ;
#12320=CARTESIAN_POINT ( 'NONE',  ( 32.07220196432897552, -5.426722983814484813, -3.627061608673668225 ) ) ;
#12322=DIRECTION ( 'NONE',  ( 0.1196152422706621143, -0.9928203230275509661, 0.000000000000000000 ) ) ;
#12323=CARTESIAN_POINT ( 'NONE',  ( 31.58296173575813981, -1.713646710223874381, -6.453230759126465266 ) ) ;
#12326=EDGE_CURVE ( 'NONE', #9522, #9058, #5516, .T. ) ;
#12328=CARTESIAN_POINT ( 'NONE',  ( 29.50659824675005893, -4.481886499472614638, -7.939653947423662039 ) ) ;
#12330=DIRECTION ( 'NONE',  ( 0.8243186046180107640, -0.5661261679878571984, -0.000000000000000000 ) ) ;
#12336=CARTESIAN_POINT ( 'NONE',  ( 28.28511899221430070, -4.629050627332469858, -3.283357778048664688 ) ) ;
#12338=EDGE_LOOP ( 'NONE', ( #8836, #2723, #14936, #3791 ) ) ;
#12339=CARTESIAN_POINT ( 'NONE',  ( 33.60446413004628141, -3.988174587000466342, -3.627061608673664672 ) ) ;
#12347=CARTESIAN_POINT ( 'NONE',  ( -28.91489957058744409, -14.18850833160549207, -13.46727466850441601 ) ) ;
#12348=ORIENTED_EDGE ( 'NONE', *, *, #11893, .T. ) ;
#12349=CARTESIAN_POINT ( 'NONE',  ( 30.92509028327567933, -4.310986222078405206, -7.939653947423662039 ) ) ;
#12350=DIRECTION ( 'NONE',  ( 0.000000000000000000, 0.000000000000000000, 1.000000000000000000 ) ) ;
#12351=EDGE_CURVE ( 'NONE', #16041, #11613, #9678, .T. ) ;
#12353=CARTESIAN_POINT ( 'NONE',  ( 32.67202617590239555, -5.981426544730773287, -4.705209693361168455 ) ) ;
#12358=CARTESIAN_POINT ( 'NONE',  ( 23.43992347230441453, -22.46596520570847844, -14.83047979245100656 ) ) ;
#12360=ORIENTED_EDGE ( 'NONE', *, *, #11729, .T. ) ;
#12361=EDGE_CURVE ( 'NONE', #6537, #7694, #4805, .T. ) ;
#12363=B_SPLINE_CURVE_WITH_KNOTS ( 'NONE', 1,
 ( #15585, #7080 ),
 .UNSPECIFIED., .F., .F.,
 ( 2, 2 ),
 ( 0.000000000000000000, 1.000000000000000000 ),
 .UNSPECIFIED. ) ;
#12366=EDGE_LOOP ( 'NONE', ( #6003, #295, #1751, #12908 ) ) ;
#12367=ORIENTED_EDGE ( 'NONE', *, *, #1138, .F. ) ;
#12369=DIRECTION ( 'NONE',  ( 0.1196152422706605323, -0.9928203230275512992, 0.000000000000000000 ) ) ;
#12370=EDGE_CURVE ( 'NONE', #13758, #15536, #9018, .T. ) ;
#12371=CARTESIAN_POINT ( 'NONE',  ( 28.30694982360322953, -3.372479377640031473, -7.939653947423660263 ) ) ;
#12382=EDGE_CURVE ( 'NONE', #2104, #16590, #10040, .T. ) ;
#12383=ORIENTED_EDGE ( 'NONE', *, *, #12039, .F. ) ;
#12386=VERTEX_POINT ( 'NONE', #1549 ) ;
#12402=CARTESIAN_POINT ( 'NONE',  ( 28.41655006632555569, -6.494127376913395366, -4.705209693361169343 ) ) ;
#12404=ORIENTED_EDGE ( 'NONE', *, *, #16011, .T. ) ;
#12405=CARTESIAN_POINT ( 'NONE',  ( 31.90644508241650357, -6.373472726347483963, -7.033357778048666908 ) ) ;
#12408=ORIENTED_EDGE ( 'NONE', *, *, #16637, .F. ) ;
#12410=CARTESIAN_POINT ( 'NONE',  ( 27.60205212784272177, -2.830435096530727446, -4.705209693361161349 ) ) ;
#12411=( BOUNDED_CURVE ( )  B_SPLINE_CURVE ( 2, ( #17155, #10311, #15868, #4879, #17341, #6057, #6434, #11861, #3440 ),
 .UNSPECIFIED., .F., .T. ) 
 B_SPLINE_CURVE_WITH_KNOTS ( ( 3, 2, 2, 2, 3 ),
 ( 0.2500000000000000000, 0.2564102564102563875, 0.2692307692307692180, 0.2820512820512820484, 0.2884615384615384914 ),
 .UNSPECIFIED. ) 
 CURVE ( )  GEOMETRIC_REPRESENTATION_ITEM ( )  RATIONAL_B_SPLINE_CURVE ( ( 0.9330127018922194093, 0.9330127018922195203, 1.000000000000000000, 0.8660254037844387076, 1.000000000000000000, 0.8660254037844387076, 1.000000000000000000, 0.9330127018922190762, 0.9330127018922194093 ) ) 
 REPRESENTATION_ITEM ( '' )  );
#12418=AXIS2_PLACEMENT_3D ( 'NONE', #17852, #5372, #7942 ) ;
#12420=CARTESIAN_POINT ( 'NONE',  ( 27.65467808709180630, -4.705006306174339237, -3.283357778048664688 ) ) ;
#12422=CARTESIAN_POINT ( 'NONE',  ( 29.39282811755836633, -5.749534618892433002, -3.627061608673667781 ) ) ;
#12424=CARTESIAN_POINT ( 'NONE',  ( 26.01652455409633902, -4.902371455920928156, -5.783357778048663356 ) ) ;
#12426=AXIS2_PLACEMENT_3D ( 'NONE', #9723, #11452, #17019 ) ;
#12432=ORIENTED_EDGE ( 'NONE', *, *, #14879, .F. ) ;
#12433=ORIENTED_EDGE ( 'NONE', *, *, #2769, .F. ) ;
#12435=CARTESIAN_POINT ( 'NONE',  ( 34.91600907648203389, -11.88801210197604341, -11.56671555609732671 ) ) ;
#12437=EDGE_LOOP ( 'NONE', ( #5572, #8902 ) ) ;
#12439=CARTESIAN_POINT ( 'NONE',  ( 29.78250536075762867, -6.329556739422670830, -6.861505862736167138 ) ) ;
#12440=CARTESIAN_POINT ( 'NONE',  ( 28.82057243903374655, -7.082618055128190093, -5.783357778048668685 ) ) ;
#12443=EDGE_CURVE ( 'NONE', #7377, #3411, #11053, .T. ) ;
#12444=CARTESIAN_POINT ( 'NONE',  ( 27.32822876973539294, -6.198150586942257512, -3.283357778048667797 ) ) ;
#12457=ORIENTED_EDGE ( 'NONE', *, *, #6806, .F. ) ;
#12462=CARTESIAN_POINT ( 'NONE',  ( 29.56783163384821833, -3.220568019956291383, -7.939653947423660263 ) ) ;
#12468=AXIS2_PLACEMENT_3D ( 'NONE', #11207, #8334, #183 ) ;
#12469=ADVANCED_FACE ( 'NONE', ( #11859 ), #8799, .F. ) ;
#12472=DIRECTION ( 'NONE',  ( 0.000000000000000000, 0.000000000000000000, 1.000000000000000000 ) ) ;
#12474=ORIENTED_EDGE ( 'NONE', *, *, #5286, .F. ) ;
#12482=CARTESIAN_POINT ( 'NONE',  ( 32.95080301609915097, -1.548848848676412260, -5.783357778048663356 ) ) ;
#12490=DIRECTION ( 'NONE',  ( 0.9928203230275512992, 0.1196152422706614898, -0.000000000000000000 ) ) ;
#12491=CARTESIAN_POINT ( 'NONE',  ( 21.62432203902686823, -10.11801842300244125, -15.20615207729255403 ) ) ;
#12492=DIRECTION ( 'NONE',  ( -0.000000000000000000, -0.000000000000000000, -1.000000000000000000 ) ) ;
#12495=ORIENTED_EDGE ( 'NONE', *, *, #6450, .T. ) ;
#12499=CYLINDRICAL_SURFACE ( 'NONE', #13860, 95.00000000000000000 ) ;
#12500=VECTOR ( 'NONE', #8076, 1000.000000000000114 ) ;
#12501=ORIENTED_EDGE ( 'NONE', *, *, #2485, .F. ) ;
#12508=LINE ( 'NONE', #9677, #8672 ) ;
#12513=VECTOR ( 'NONE', #12109, 1000.000000000000000 ) ;
#12516=CARTESIAN_POINT ( 'NONE',  ( 29.14074637024071635, -5.979778010479330774, -3.283357778048667797 ) ) ;
#12518=CARTESIAN_POINT ( 'NONE',  ( 31.25770402584614516, -1.763030703431812674, -5.783357778048658027 ) ) ;
#12520=DIRECTION ( 'NONE',  ( 0.9928203230275512992, 0.1196152422706614898, -0.000000000000000000 ) ) ;
#12526=CARTESIAN_POINT ( 'NONE',  ( 29.95125523467787332, -2.974500528818129652, -3.283357778048662023 ) ) ;
#12527=EDGE_CURVE ( 'NONE', #14539, #5005, #9769, .T. ) ;
#12529=CARTESIAN_POINT ( 'NONE',  ( -17.60362937644963921, -13.05831870693043584, -15.90927928682413928 ) ) ;
#12531=VERTEX_POINT ( 'NONE', #13502 ) ;
#12532=CARTESIAN_POINT ( 'NONE',  ( 28.39010325924584421, -2.735490497978389612, -4.705209693361160461 ) ) ;
#12535=VERTEX_POINT ( 'NONE', #14945 ) ;
#12536=CARTESIAN_POINT ( 'NONE',  ( 31.88814493096863956, -1.687075024589942851, -5.783357778048658027 ) ) ;
#12537=EDGE_CURVE ( 'NONE', #3273, #16640, #1695, .T. ) ;
#12548=CARTESIAN_POINT ( 'NONE',  ( 25.71748644841968456, -2.420320648352051851, -5.783357778048663356 ) ) ;
#12549=VERTEX_POINT ( 'NONE', #16326 ) ;
#12551=ORIENTED_EDGE ( 'NONE', *, *, #11842, .T. ) ;
#12552=FACE_OUTER_BOUND ( 'NONE', #15903, .T. ) ;
#12554=CARTESIAN_POINT ( 'NONE',  ( 27.14244485254070938, -4.766720295129625029, -7.939653947423662039 ) ) ;
#12555=CARTESIAN_POINT ( 'NONE',  ( 31.29094215978502547, -2.813094711071706389, -3.283357778048662023 ) ) ;
#12565=ORIENTED_EDGE ( 'NONE', *, *, #10949, .T. ) ;
#12566=VERTEX_POINT ( 'NONE', #997 ) ;
#12569=CYLINDRICAL_SURFACE ( 'NONE', #12239, 5.000000000000000000 ) ;
#12572=ORIENTED_EDGE ( 'NONE', *, *, #6411, .T. ) ;
#12578=CARTESIAN_POINT ( 'NONE',  ( 33.50243880635947846, -1.482387629897225390, -5.783357778048663356 ) ) ;
#12584=CARTESIAN_POINT ( 'NONE',  ( 17.93919565825226670, -12.54482367096064621, -15.85739159820981747 ) ) ;
#12586=EDGE_CURVE ( 'NONE', #16822, #15540, #15702, .T. ) ;
#12595=CARTESIAN_POINT ( 'NONE',  ( 29.37220822929407760, -7.016156836349003001, -5.783357778048668685 ) ) ;
#12596=DIRECTION ( 'NONE',  ( -1.000000000000000000, 0.000000000000000000, 0.000000000000000000 ) ) ;
#12599=CARTESIAN_POINT ( 'NONE',  ( 32.32036211097666012, -1.624804527518282748, -5.783357778048663356 ) ) ;
#12602=CARTESIAN_POINT ( 'NONE',  ( 31.94462260941237020, -6.706231704719880504, -5.113484796970860558 ) ) ;
#12606=CARTESIAN_POINT ( 'NONE',  ( 27.49335874655903567, -6.905162478240574053, -7.033357778048666908 ) ) ;
#12608=CARTESIAN_POINT ( 'NONE',  ( 30.78070346053490880, -6.209293581256383199, -4.705209693361168455 ) ) ;
#12615=ORIENTED_EDGE ( 'NONE', *, *, #7915, .T. ) ;
#12616=DIRECTION ( 'NONE',  ( 0.9928203230275510771, 0.1196152422706614621, -0.000000000000000000 ) ) ;
#12620=ORIENTED_EDGE ( 'NONE', *, *, #443, .T. ) ;
#12621=CARTESIAN_POINT ( 'NONE',  ( 26.62577407660990758, -3.575027854551694695, -3.627061608673662008 ) ) ;
#12623=ADVANCED_FACE ( 'NONE', ( #14859, #3973 ), #9488, .F. ) ;
#12625=CARTESIAN_POINT ( 'NONE',  ( 29.62036837594175154, -3.214238380052812261, -3.627061608673662896 ) ) ;
#12640=CARTESIAN_POINT ( 'NONE',  ( 25.86833963875586306, -3.039313213345869791, -4.705209693361160461 ) ) ;
#12641=CARTESIAN_POINT ( 'NONE',  ( 33.04340326765378677, -1.875050963503474222, -4.533357778048659803 ) ) ;
#12646=EDGE_CURVE ( 'NONE', #3121, #16638, #1075, .T. ) ;
#12647=DIRECTION ( 'NONE',  ( -1.000000000000000000, 0.000000000000000000, 0.000000000000000000 ) ) ;
#12648=CARTESIAN_POINT ( 'NONE',  ( -11.38175538881593774, -22.33742387525457573, -16.67884400577319681 ) ) ;
#12665=LINE ( 'NONE', #12758, #4023 ) ;
#12679=LINE ( 'NONE', #2996, #3720 ) ;
#12683=DIRECTION ( 'NONE',  ( -0.000000000000000000, -0.000000000000000000, -1.000000000000000000 ) ) ;
#12689=CARTESIAN_POINT ( 'NONE',  ( 29.01637427789896151, -7.048830937829683840, -5.783357778048668685 ) ) ;
#12694=DIRECTION ( 'NONE',  ( -0.000000000000000000, -0.000000000000000000, -1.000000000000000000 ) ) ;
#12695=EDGE_CURVE ( 'NONE', #5484, #7696, #7262, .T. ) ;
#12697=FACE_BOUND ( 'NONE', #5309, .T. ) ;
#12698=( BOUNDED_CURVE ( )  B_SPLINE_CURVE ( 2, ( #10185, #12828, #14186, #11447, #1959, #1777, #15457, #6109, #7307 ),
 .UNSPECIFIED., .F., .T. ) 
 B_SPLINE_CURVE_WITH_KNOTS ( ( 3, 2, 2, 2, 3 ),
 ( 0.7884615384615384359, 0.7948717948717948234, 0.8076923076923077094, 0.8205128205128204844, 0.8269230769230769829 ),
 .UNSPECIFIED. ) 
 CURVE ( )  GEOMETRIC_REPRESENTATION_ITEM ( )  RATIONAL_B_SPLINE_CURVE ( ( 0.9330127018922194093, 0.9330127018922194093, 1.000000000000000000, 0.8660254037844387076, 1.000000000000000000, 0.8660254037844387076, 1.000000000000000000, 0.9330127018922187432, 0.9330127018922192983 ) ) 
 REPRESENTATION_ITEM ( '' )  );
#12704=CARTESIAN_POINT ( 'NONE',  ( -23.00000000000000000, -16.21813761408365195, -13.00000000000000178 ) ) ;
#12706=CARTESIAN_POINT ( 'NONE',  ( 27.23882169172318513, -6.009049854935478052, -7.939653947423662927 ) ) ;
#12707=EDGE_LOOP ( 'NONE', ( #9697, #14622, #11867, #6923 ) ) ;
#12708=CARTESIAN_POINT ( 'NONE',  ( 28.77978050244509944, -3.315512618508630993, -7.939653947423660263 ) ) ;
#12709=FACE_OUTER_BOUND ( 'NONE', #4254, .T. ) ;
#12714=CARTESIAN_POINT ( 'NONE',  ( 18.32374253600956493, -20.38504502893476200, -15.79679025666372283 ) ) ;
#12715=EDGE_LOOP ( 'NONE', ( #5895, #16367, #12572, #15538 ) ) ;
#12718=AXIS2_PLACEMENT_3D ( 'NONE', #2079, #3513, #13301 ) ;
#12719=ADVANCED_FACE ( 'NONE', ( #7237 ), #12753, .F. ) ;
#12728=CARTESIAN_POINT ( 'NONE',  ( 27.10304229683147526, -4.771467524953526329, -3.283357778048664688 ) ) ;
#12729=CARTESIAN_POINT ( 'NONE',  ( 33.55383270609817714, -5.448088258586239796, -3.283357778048667797 ) ) ;
#12730=CARTESIAN_POINT ( 'NONE',  ( 31.38859741546781379, -7.162769935976271540, -5.783357778048669573 ) ) ;
#12733=CARTESIAN_POINT ( 'NONE',  ( 30.35023428074701002, -1.862166024106576057, -5.783357778048664244 ) ) ;
#12734=CARTESIAN_POINT ( 'NONE',  ( 29.02054416436834217, -2.659534819136519790, -4.705209693361160461 ) ) ;
#12744=FILL_AREA_STYLE_COLOUR ( '', #919 ) ;
#12749=ORIENTED_EDGE ( 'NONE', *, *, #2508, .T. ) ;
#12752=EDGE_CURVE ( 'NONE', #17749, #2915, #8411, .T. ) ;
#12753=CYLINDRICAL_SURFACE ( 'NONE', #1810, 2.499999999999999112 ) ;
#12755=CARTESIAN_POINT ( 'NONE',  ( 32.38298487551052318, -4.135338714860305132, -8.283357778048662468 ) ) ;
#12756=VERTEX_POINT ( 'NONE', #5583 ) ;
#12758=CARTESIAN_POINT ( 'NONE',  ( 15.92260893619738837, -28.39189527176317540, -6.000000000000000000 ) ) ;
#12767=EDGE_LOOP ( 'NONE', ( #16503, #1970, #491, #10863, #8445 ) ) ;
#12769=ORIENTED_EDGE ( 'NONE', *, *, #654, .F. ) ;
#12773=CARTESIAN_POINT ( 'NONE',  ( -9.647391702364178201, 16.07861560120820243, -16.78732711007196698 ) ) ;
#12778=CARTESIAN_POINT ( 'NONE',  ( 31.83134908525019213, -4.201799933639492224, -8.283357778048662468 ) ) ;
#12784=CARTESIAN_POINT ( 'NONE',  ( 31.71314141467879111, -4.216041623526076698, -3.627061608673664672 ) ) ;
#12786=FACE_OUTER_BOUND ( 'NONE', #9896, .T. ) ;
#12787=CARTESIAN_POINT ( 'NONE',  ( 27.17934203385504333, -30.00000000000000355, 0.000000000000000000 ) ) ;
#12792=ORIENTED_EDGE ( 'NONE', *, *, #3548, .T. ) ;
#12796=CIRCLE ( 'NONE', #8449, 2.749999999999992895 ) ;
#12798=ORIENTED_EDGE ( 'NONE', *, *, #11729, .F. ) ;
#12799=CARTESIAN_POINT ( 'NONE',  ( -17.07594129529364579, -14.18356557013591868, -15.98851070825981324 ) ) ;
#12802=CARTESIAN_POINT ( 'NONE',  ( 26.37178701114681800, -2.351687214456304797, -5.783357778048658915 ) ) ;
#12803=CARTESIAN_POINT ( 'NONE',  ( 30.88577694472199298, -6.196634301449400084, -6.861505862736166250 ) ) ;
#12805=LINE ( 'NONE', #400, #3178 ) ;
#12806=VECTOR ( 'NONE', #497, 1000.000000000000000 ) ;
#12808=VECTOR ( 'NONE', #236, 1000.000000000000000 ) ;
#12813=ORIENTED_EDGE ( 'NONE', *, *, #17646, .T. ) ;
#12816=DIRECTION ( 'NONE',  ( -0.000000000000000000, -0.000000000000000000, 1.000000000000000000 ) ) ;
#12825=CARTESIAN_POINT ( 'NONE',  ( -34.91600907648203389, -11.88801210197604341, -11.56671555609732671 ) ) ;
#12828=CARTESIAN_POINT ( 'NONE',  ( 26.61823960964035507, -2.311797680896151341, -6.453230759126464378 ) ) ;
#12829=CARTESIAN_POINT ( 'NONE',  ( 26.39823381822651882, -6.110324093391315436, -3.627061608673668225 ) ) ;
#12830=CARTESIAN_POINT ( 'NONE',  ( 30.52163964716380917, -2.178873678870954400, -4.533357778048659803 ) ) ;
#12835=EDGE_CURVE ( 'NONE', #12145, #8066, #3247, .T. ) ;
#12836=CARTESIAN_POINT ( 'NONE',  ( 27.63266882139180680, -2.199775856772564708, -5.783357778048658027 ) ) ;
#12841=ORIENTED_EDGE ( 'NONE', *, *, #14940, .T. ) ;
#12846=DIRECTION ( 'NONE',  ( -0.000000000000000000, -0.000000000000000000, -1.000000000000000000 ) ) ;
#12847=VERTEX_POINT ( 'NONE', #9187 ) ;
#12848=CARTESIAN_POINT ( 'NONE',  ( 28.64916707261694384, -6.765910400363817523, -4.533357778048668685 ) ) ;
#12851=EDGE_CURVE ( 'NONE', #11613, #1319, #8683, .T. ) ;
#12859=EDGE_CURVE ( 'NONE', #14228, #6328, #9273, .T. ) ;
#12863=CARTESIAN_POINT ( 'NONE',  ( 34.91600907648203389, -11.88801210197604341, -12.00000000000000000 ) ) ;
#12870=CARTESIAN_POINT ( 'NONE',  ( 26.34117031759772942, -2.982346454214467535, -4.705209693361161349 ) ) ;
#12871=CARTESIAN_POINT ( 'NONE',  ( 20.00000000000000355, -30.00000000000000355, -17.00000000000000000 ) ) ;
#12880=CARTESIAN_POINT ( 'NONE',  ( 33.54323074294813267, -5.249493066516778050, -7.939653947423664704 ) ) ;
#12881=DIRECTION ( 'NONE',  ( 0.000000000000000000, 0.000000000000000000, 1.000000000000000000 ) ) ;
#12882=CARTESIAN_POINT ( 'NONE',  ( 26.87859896403794835, -7.316587507915443211, -6.453230759126474148 ) ) ;
#12890=ORIENTED_EDGE ( 'NONE', *, *, #16124, .T. ) ;
#12898=CARTESIAN_POINT ( 'NONE',  ( 29.51982165028991645, -6.361204938940122844, -4.705209693361168455 ) ) ;
#12908=ORIENTED_EDGE ( 'NONE', *, *, #13451, .F. ) ;
#12910=ORIENTED_EDGE ( 'NONE', *, *, #2636, .F. ) ;
#12911=CARTESIAN_POINT ( 'NONE',  ( 8.809730593168891843, -18.96833375928839516, -16.83727734034771473 ) ) ;
#12912=LINE ( 'NONE', #495, #7580 ) ;
#12914=CARTESIAN_POINT ( 'NONE',  ( 23.02601376483258022, 3.965314980223224151, 0.000000000000000000 ) ) ;
#12915=CARTESIAN_POINT ( 'NONE',  ( 33.00219691583784964, -5.514549477365426888, -3.283357778048667797 ) ) ;
#12916=DIRECTION ( 'NONE',  ( 0.1113444980252557837, 0.9937818688019538493, -0.000000000000000000 ) ) ;
#12917=DIRECTION ( 'NONE',  ( 0.000000000000000000, 0.000000000000000000, 1.000000000000000000 ) ) ;
#12931=ORIENTED_EDGE ( 'NONE', *, *, #106, .F. ) ;
#12932=CARTESIAN_POINT ( 'NONE',  ( -25.11802603177690330, -19.03270077640483038, -0.5379818257722508434 ) ) ;
#12935=CARTESIAN_POINT ( 'NONE',  ( 26.14456121274580624, -5.685614013951941992, -8.283357778048664244 ) ) ;
#12936=VECTOR ( 'NONE', #5170, 1000.000000000000000 ) ;
#12958=DIRECTION ( 'NONE',  ( -0.1196152422706611151, 0.9928203230275511881, 0.000000000000000000 ) ) ;
#12965=CARTESIAN_POINT ( 'NONE',  ( 28.36401332423200827, -6.500457016816879374, -6.861505862736166250 ) ) ;
#12969=VERTEX_POINT ( 'NONE', #12075 ) ;
#12971=AXIS2_PLACEMENT_3D ( 'NONE', #6263, #2017, #13338 ) ;
#12974=ORIENTED_EDGE ( 'NONE', *, *, #3204, .T. ) ;
#12976=CARTESIAN_POINT ( 'NONE',  ( 31.93198502805756789, -2.935734224299280548, -7.939653947423660263 ) ) ;
#12977=EDGE_LOOP ( 'NONE', ( #10892, #16891 ) ) ;
#12978=CARTESIAN_POINT ( 'NONE',  ( 29.15568435273173264, -2.343444316361667834, -7.033357778048658027 ) ) ;
#12980=AXIS2_PLACEMENT_3D ( 'NONE', #16143, #14775, #4786 ) ;
#12981=CARTESIAN_POINT ( 'NONE',  ( 28.52162355051263987, -6.481468097106410475, -6.861505862736167138 ) ) ;
#12983=VECTOR ( 'NONE', #16977, 1000.000000000000000 ) ;
#12985=CARTESIAN_POINT ( 'NONE',  ( 27.93049598394382116, -4.671775696577297410, -3.627061608673664672 ) ) ;
#12987=CARTESIAN_POINT ( 'NONE',  ( 32.84384354600314282, -1.561735352540135180, -6.453230759126467042 ) ) ;
#12992=AXIS2_PLACEMENT_3D ( 'NONE', #9720, #2853, #6669 ) ;
#12995=CARTESIAN_POINT ( 'NONE',  ( 25.74999999999998934, -16.21813761408365195, -13.00000000000000355 ) ) ;
#13001=CARTESIAN_POINT ( 'NONE',  ( 3.538288549924106796, -15.34800872113743431, -16.99955934415557479 ) ) ;
#13003=EDGE_CURVE ( 'NONE', #2915, #17680, #15550, .T. ) ;
#13006=CARTESIAN_POINT ( 'NONE',  ( 30.61929490284659394, -6.528548903775525325, -4.533357778048668685 ) ) ;
#13009=CARTESIAN_POINT ( 'NONE',  ( 7.499998387031003411, -20.49508120620799900, -12.00000000000000000 ) ) ;
#13021=EDGE_LOOP ( 'NONE', ( #13528, #7064, #2463, #7564 ) ) ;
#13022=CARTESIAN_POINT ( 'NONE',  ( -3.248936832696171617, -15.16081378324841111, -17.00000000000000000 ) ) ;
#13024=EDGE_CURVE ( 'NONE', #5360, #2932, #8163, .T. ) ;
#13032=ORIENTED_EDGE ( 'NONE', *, *, #106, .T. ) ;
#13038=EDGE_LOOP ( 'NONE', ( #3076, #17598, #10354, #12931 ) ) ;
#13040=ORIENTED_EDGE ( 'NONE', *, *, #8255, .F. ) ;
#13043=CARTESIAN_POINT ( 'NONE',  ( -8.812506826975363694, -18.97024042328638416, -16.83711976780714181 ) ) ;
#13044=CARTESIAN_POINT ( 'NONE',  ( -3.248936832696171617, 17.78798921770683350, -17.00000000000000000 ) ) ;
#13046=CARTESIAN_POINT ( 'NONE',  ( -17.08586189024356727, -18.24992599651649527, -15.98693133205340189 ) ) ;
#13048=CARTESIAN_POINT ( 'NONE',  ( -7.499998387031003411, -20.49508120620799900, -13.00000000000000178 ) ) ;
#13054=CIRCLE ( 'NONE', #2372, 5.000000000000000000 ) ;
#13057=AXIS2_PLACEMENT_3D ( 'NONE', #3276, #1835, #3175 ) ;
#13058=CARTESIAN_POINT ( 'NONE',  ( 28.10549950023366961, -2.142809097641162897, -5.783357778048658027 ) ) ;
#13059=CARTESIAN_POINT ( 'NONE',  ( 0.000000000000000000, 0.000000000000000000, -10.50000000000000000 ) ) ;
#13065=ORIENTED_EDGE ( 'NONE', *, *, #2887, .T. ) ;
#13066=DIRECTION ( 'NONE',  ( 0.9928203230275512992, 0.1196152422706614898, -0.000000000000000000 ) ) ;
#13068=CARTESIAN_POINT ( 'NONE',  ( 32.56242593318006584, -2.859778545457409837, -7.939653947423660263 ) ) ;
#13069=VERTEX_POINT ( 'NONE', #16437 ) ;
#13071=CARTESIAN_POINT ( 'NONE',  ( 25.96814307759224150, -4.500799614243312874, -8.119953194407841579 ) ) ;
#13074=EDGE_CURVE ( 'NONE', #17574, #1161, #10957, .T. ) ;
#13076=CARTESIAN_POINT ( 'NONE',  ( 26.46816385032927599, -3.594016774262162706, -3.627061608673662896 ) ) ;
#13078=CYLINDRICAL_SURFACE ( 'NONE', #6406, 2.499999999999999112 ) ;
#13079=CARTESIAN_POINT ( 'NONE',  ( 33.15485366002904755, -6.560422763297783177, -5.783357778048663356 ) ) ;
#13082=ORIENTED_EDGE ( 'NONE', *, *, #992, .T. ) ;
#13084=CARTESIAN_POINT ( 'NONE',  ( -25.11802603177690330, -16.03270077640482683, -10.53798182577225084 ) ) ;
#13086=EDGE_LOOP ( 'NONE', ( #17449, #10927, #3733, #17823, #15162 ) ) ;
#13092=CARTESIAN_POINT ( 'NONE',  ( -23.47400307746860548, -29.47066586337336247, -14.90105725137467552 ) ) ;
#13093=CARTESIAN_POINT ( 'NONE',  ( 34.91600907648203389, -11.88801210197604341, -11.56671555609732671 ) ) ;
#13095=CARTESIAN_POINT ( 'NONE',  ( 26.21973641492267859, -6.589053366008232437, -7.643209271886766132 ) ) ;
#13103=CARTESIAN_POINT ( 'NONE',  ( 29.78612525785423060, -2.267488637519798012, -7.033357778048658027 ) ) ;
#13104=CARTESIAN_POINT ( 'NONE',  ( 25.11802603177690330, -19.03270077640483038, -0.5379818257722508434 ) ) ;
#13118=ORIENTED_EDGE ( 'NONE', *, *, #8317, .F. ) ;
#13119=CARTESIAN_POINT ( 'NONE',  ( 27.82847066025702887, -2.165988739474055791, -5.783357778048658027 ) ) ;
#13131=LINE ( 'NONE', #6233, #610 ) ;
#13139=CARTESIAN_POINT ( 'NONE',  ( 19.71718888926881164, -28.93397812220195675, -15.64003640126281347 ) ) ;
#13143=DIRECTION ( 'NONE',  ( 0.9928203230275512992, 0.1196152422706614482, 0.000000000000000000 ) ) ;
#13151=CARTESIAN_POINT ( 'NONE',  ( 27.75549246765397271, -7.200742295513423485, -5.783357778048668685 ) ) ;
#13154=DIRECTION ( 'NONE',  ( -0.1414213562373112243, -0.9899494936611663576, 0.000000000000000000 ) ) ;
#13158=ORIENTED_EDGE ( 'NONE', *, *, #17416, .F. ) ;
#13161=CARTESIAN_POINT ( 'NONE',  ( 32.34358231980129261, -4.140085944684206432, -3.627061608673664672 ) ) ;
#13162=ORIENTED_EDGE ( 'NONE', *, *, #5854, .F. ) ;
#13169=CARTESIAN_POINT ( 'NONE',  ( 27.63266882139180680, -2.199775856772564708, -5.783357778048658027 ) ) ;
#13172=CARTESIAN_POINT ( 'NONE',  ( -2.016448651773435938E-27, -20.49999999999999645, -6.000000000000000000 ) ) ;
#13174=CARTESIAN_POINT ( 'NONE',  ( 25.90934487712385348, 0.1208734971681838660, -5.783357778048663356 ) ) ;
#13176=FACE_OUTER_BOUND ( 'NONE', #3927, .T. ) ;
#13178=EDGE_LOOP ( 'NONE', ( #1564, #12551, #10492, #13734, #3621, #2869 ) ) ;
#13179=LINE ( 'NONE', #11803, #1982 ) ;
#13180=DIRECTION ( 'NONE',  ( -1.000000000000000000, 0.000000000000000000, 0.000000000000000000 ) ) ;
#13187=CARTESIAN_POINT ( 'NONE',  ( 32.32618902979206865, -6.650063623909865385, -5.783357778048669573 ) ) ;
#13189=EDGE_CURVE ( 'NONE', #17076, #8674, #3179, .T. ) ;
#13190=CARTESIAN_POINT ( 'NONE',  ( 28.49145532429760053, -1.696564004353941613, -5.783357778048658027 ) ) ;
#13197=CARTESIAN_POINT ( 'NONE',  ( 31.86581749455020329, -6.715726164782562790, -5.113484796970860558 ) ) ;
#13199=EDGE_CURVE ( 'NONE', #6265, #227, #7778, .T. ) ;
#13202=ORIENTED_EDGE ( 'NONE', *, *, #9983, .T. ) ;
#13206=ORIENTED_EDGE ( 'NONE', *, *, #16971, .F. ) ;
#13207=DIRECTION ( 'NONE',  ( -1.000000000000000000, 0.000000000000000000, 0.000000000000000000 ) ) ;
#13211=DIRECTION ( 'NONE',  ( -0.1196152422706597551, 0.9928203230275514102, 0.000000000000000000 ) ) ;
#13213=EDGE_CURVE ( 'NONE', #16314, #8286, #7094, .T. ) ;
#13215=DIRECTION ( 'NONE',  ( -0.000000000000000000, -0.000000000000000000, -1.000000000000000000 ) ) ;
#13218=CARTESIAN_POINT ( 'NONE',  ( 31.63927044622584717, -1.706862622621797110, -5.113484796970854340 ) ) ;
#13236=CARTESIAN_POINT ( 'NONE',  ( 26.49461065740898036, -7.352653653197164019, -5.783357778048668685 ) ) ;
#13239=CARTESIAN_POINT ( 'NONE',  ( 20.25000000000000355, -16.21813761408365195, 0.000000000000000000 ) ) ;
#13243=DIRECTION ( 'NONE',  ( -0.1196152422706611984, 0.9928203230275510771, 0.000000000000000000 ) ) ;
#13244=CARTESIAN_POINT ( 'NONE',  ( 32.14665875496697822, -6.044722943765660439, -6.861505862736166250 ) ) ;
#13246=DIRECTION ( 'NONE',  ( 0.000000000000000000, 0.000000000000000000, -1.000000000000000000 ) ) ;
#13247=CARTESIAN_POINT ( 'NONE',  ( 25.80383423833348644, -3.137017275366889901, -7.141595990038014818 ) ) ;
#13248=ORIENTED_EDGE ( 'NONE', *, *, #8489, .T. ) ;
#13250=CARTESIAN_POINT ( 'NONE',  ( 33.10345976029034176, -2.594722134608779207, -3.283357778048662023 ) ) ;
#13254=CARTESIAN_POINT ( 'NONE',  ( 26.49461065740898036, -7.352653653197164019, -5.783357778048668685 ) ) ;
#13256=LINE ( 'NONE', #838, #14102 ) ;
#13261=( BOUNDED_CURVE ( )  B_SPLINE_CURVE ( 2, ( #10729, #6580, #12105, #8293, #14926, #5383, #15006, #17687, #5210 ),
 .UNSPECIFIED., .F., .T. ) 
 B_SPLINE_CURVE_WITH_KNOTS ( ( 3, 2, 2, 2, 3 ),
 ( 0.3269230769230769273, 0.3333333333333333148, 0.3461538461538461453, 0.3589743589743589758, 0.3653846153846154188 ),
 .UNSPECIFIED. ) 
 CURVE ( )  GEOMETRIC_REPRESENTATION_ITEM ( )  RATIONAL_B_SPLINE_CURVE ( ( 0.9330127018922194093, 0.9330127018922194093, 1.000000000000000000, 0.8660254037844387076, 1.000000000000000000, 0.8660254037844387076, 1.000000000000000000, 0.9330127018922190762, 0.9330127018922194093 ) ) 
 REPRESENTATION_ITEM ( '' )  );
#13262=CIRCLE ( 'NONE', #11511, 5.000000000000000888 ) ;
#13264=PLANE ( 'NONE',  #16243 ) ;
#13265=CIRCLE ( 'NONE', #17929, 2.000000000000001776 ) ;
#13267=ORIENTED_EDGE ( 'NONE', *, *, #12361, .T. ) ;
#13270=CARTESIAN_POINT ( 'NONE',  ( 33.76207435632690590, -3.969185667289998332, -3.627061608673664672 ) ) ;
#13274=CARTESIAN_POINT ( 'NONE',  ( 27.36943512155133362, -2.558652073080304845, -4.533357778048659803 ) ) ;
#13283=EDGE_CURVE ( 'NONE', #13718, #6265, #16073, .T. ) ;
#13286=ORIENTED_EDGE ( 'NONE', *, *, #10691, .T. ) ;
#13288=ORIENTED_EDGE ( 'NONE', *, *, #5707, .F. ) ;
#13290=CARTESIAN_POINT ( 'NONE',  ( 29.25000000000000000, -16.21813761408365195, -13.37255996287876236 ) ) ;
#13291=CARTESIAN_POINT ( 'NONE',  ( 32.21340264088064487, -1.637691031382005669, -6.453230759126468818 ) ) ;
#13301=DIRECTION ( 'NONE',  ( 1.000000000000000000, 0.000000000000000000, 0.000000000000000000 ) ) ;
#13303=AXIS2_PLACEMENT_3D ( 'NONE', #14191, #4927, #14472 ) ;
#13305=CARTESIAN_POINT ( 'NONE',  ( 33.15485366002904755, -6.560422763297783177, -5.783357778048663356 ) ) ;
#13307=CARTESIAN_POINT ( 'NONE',  ( 26.61898274975073164, -6.283600725846810953, -3.283357778048667797 ) ) ;
#13310=VERTEX_POINT ( 'NONE', #7714 ) ;
#13311=VERTEX_POINT ( 'NONE', #13239 ) ;
#13316=AXIS2_PLACEMENT_3D ( 'NONE', #5298, #4137, #12107 ) ;
#13328=CARTESIAN_POINT ( 'NONE',  ( 27.14244485254070938, -4.766720295129625029, -7.939653947423662039 ) ) ;
#13330=CARTESIAN_POINT ( 'NONE',  ( 33.46007730730551799, -5.886481946178435010, -4.705209693361169343 ) ) ;
#13335=CIRCLE ( 'NONE', #5214, 2.499999999999998668 ) ;
#13338=DIRECTION ( 'NONE',  ( -0.1196152422706621143, -0.9928203230275509661, 0.000000000000000000 ) ) ;
#13339=CARTESIAN_POINT ( 'NONE',  ( 33.19286683830256379, -2.783822866615540459, -7.939653947423660263 ) ) ;
#13347=CARTESIAN_POINT ( 'NONE',  ( 31.30979230060565044, -7.172264396038955603, -5.783357778048669573 ) ) ;
#13350=ORIENTED_EDGE ( 'NONE', *, *, #11209, .F. ) ;
#13351=CARTESIAN_POINT ( 'NONE',  ( 29.01637427789896151, -7.048830937829683840, -5.783357778048668685 ) ) ;
#13352=CARTESIAN_POINT ( 'NONE',  ( -27.17934203385504333, -30.00000000000000355, -13.93658524716016878 ) ) ;
#13353=CARTESIAN_POINT ( 'NONE',  ( 30.32207992551315812, -1.865558067907615802, -6.453230759126468818 ) ) ;
#13357=CIRCLE ( 'NONE', #2084, 2.000000000000001776 ) ;
#13359=CIRCLE ( 'NONE', #8431, 2.499999999999998668 ) ;
#13361=LINE ( 'NONE', #3659, #8338 ) ;
#13362=LINE ( 'NONE', #11991, #15950 ) ;
#13369=CARTESIAN_POINT ( 'NONE',  ( 30.48043329534786849, -5.818372192732907067, -3.283357778048667797 ) ) ;
#13370=CARTESIAN_POINT ( 'NONE',  ( -3.443595183066686438, -15.28297513750540837, -16.99984776326509106 ) ) ;
#13381=ORIENTED_EDGE ( 'NONE', *, *, #10085, .T. ) ;
#13386=ORIENTED_EDGE ( 'NONE', *, *, #1420, .F. ) ;
#13389=CIRCLE ( 'NONE', #9606, 6.249999999999998224 ) ;
#13391=CARTESIAN_POINT ( 'NONE',  ( 34.43754810739937966, -7.916730809865823559, -5.783357778048663356 ) ) ;
#13393=CARTESIAN_POINT ( 'NONE',  ( 31.66930131758986988, -2.967382423816733894, -3.627061608673662008 ) ) ;
#13394=ADVANCED_FACE ( 'NONE', ( #7449 ), #15978, .T. ) ;
#13398=CARTESIAN_POINT ( 'NONE',  ( 29.77044413525282707, -1.932019286686802895, -6.453230759126468818 ) ) ;
#13401=CARTESIAN_POINT ( 'NONE',  ( 25.93714794488954212, -2.393855775999666591, -5.783357778048658027 ) ) ;
#13408=ADVANCED_FACE ( 'NONE', ( #10241 ), #3546, .F. ) ;
#13418=CYLINDRICAL_SURFACE ( 'NONE', #13652, 13.00000000000000178 ) ;
#13423=CARTESIAN_POINT ( 'NONE',  ( 27.65911562847151117, -5.958412735707574015, -3.627061608673668225 ) ) ;
#13427=CARTESIAN_POINT ( 'NONE',  ( 32.69811611091622439, -2.216460025892273311, -6.861505862736158257 ) ) ;
#13431=CYLINDRICAL_SURFACE ( 'NONE', #1987, 2.499999999999999112 ) ;
#13435=CARTESIAN_POINT ( 'NONE',  ( 27.47505859511117521, -2.218764776483033163, -5.783357778048658915 ) ) ;
#13438=LINE ( 'NONE', #5251, #3782 ) ;
#13440=CARTESIAN_POINT ( 'NONE',  ( 32.96459815279162342, -1.884545423566157174, -4.533357778048659803 ) ) ;
#13441=ORIENTED_EDGE ( 'NONE', *, *, #938, .T. ) ;
#13443=CARTESIAN_POINT ( 'NONE',  ( 32.34358231980129261, -4.140085944684206432, -3.627061608673664672 ) ) ;
#13445=DIRECTION ( 'NONE',  ( 0.000000000000000000, 1.000000000000000000, 0.000000000000000000 ) ) ;
#13449=VECTOR ( 'NONE', #8351, 1000.000000000000227 ) ;
#13451=EDGE_CURVE ( 'NONE', #7372, #9007, #14789, .T. ) ;
#13452=ORIENTED_EDGE ( 'NONE', *, *, #8873, .F. ) ;
#13453=VERTEX_POINT ( 'NONE', #13775 ) ;
#13455=CARTESIAN_POINT ( 'NONE',  ( -28.84390385427241199, -13.99246034770667713, -13.48718205731130304 ) ) ;
#13456=EDGE_LOOP ( 'NONE', ( #8771, #4547, #3963, #11354 ) ) ;
#13461=CARTESIAN_POINT ( 'NONE',  ( 32.69811611091622439, -2.216460025892273311, -6.861505862736158257 ) ) ;
#13463=CARTESIAN_POINT ( 'NONE',  ( -34.91600907648203389, -11.88801210197604341, 0.000000000000000000 ) ) ;
#13464=ADVANCED_FACE ( 'NONE', ( #8156 ), #13431, .F. ) ;
#13465=CARTESIAN_POINT ( 'NONE',  ( 33.30246708102489350, -5.905470865888903020, -4.705209693361168455 ) ) ;
#13466=DIRECTION ( 'NONE',  ( 0.000000000000000000, 0.000000000000000000, 1.000000000000000000 ) ) ;
#13468=DIRECTION ( 'NONE',  ( 0.000000000000000000, -1.000000000000000000, 0.000000000000000000 ) ) ;
#13478=LINE ( 'NONE', #9298, #9060 ) ;
#13482=CARTESIAN_POINT ( 'NONE',  ( 31.43723430067123914, -2.368371383576012956, -6.861505862736158257 ) ) ;
#13484=FACE_OUTER_BOUND ( 'NONE', #1577, .T. ) ;
#13488=EDGE_CURVE ( 'NONE', #9311, #5626, #6795, .T. ) ;
#13490=CARTESIAN_POINT ( 'NONE',  ( 28.19013153391124860, -7.158573733970061248, -5.783357778048657138 ) ) ;
#13495=ORIENTED_EDGE ( 'NONE', *, *, #218, .T. ) ;
#13499=VERTEX_POINT ( 'NONE', #2535 ) ;
#13502=CARTESIAN_POINT ( 'NONE',  ( -35.74085044863416272, -23.57886868891566223, -11.27079897466147607 ) ) ;
#13505=CARTESIAN_POINT ( 'NONE',  ( 28.53771668024168662, -2.080538600569502794, -5.783357778048658027 ) ) ;
#13510=ORIENTED_EDGE ( 'NONE', *, *, #3300, .T. ) ;
#13511=EDGE_CURVE ( 'NONE', #2866, #17749, #15832, .T. ) ;
#13513=CARTESIAN_POINT ( 'NONE',  ( 32.28234893270314387, -5.401404424200516807, -7.939653947423664704 ) ) ;
#13518=EDGE_CURVE ( 'NONE', #4359, #2334, #16744, .T. ) ;
#13521=CARTESIAN_POINT ( 'NONE',  ( 28.56093688906631911, -4.595820017735426255, -3.627061608673664672 ) ) ;
#13522=CARTESIAN_POINT ( 'NONE',  ( 8.632250723006720250, -18.84644399697197770, -13.00000000000000178 ) ) ;
#13526=CARTESIAN_POINT ( 'NONE',  ( 30.30397292480292037, -1.478191427891014431, -5.783357778048658027 ) ) ;
#13528=ORIENTED_EDGE ( 'NONE', *, *, #13897, .F. ) ;
#13529=CARTESIAN_POINT ( 'NONE',  ( 32.51858583609114106, -1.611119345748072362, -5.783357778048658027 ) ) ;
#13531=CARTESIAN_POINT ( 'NONE',  ( 23.00000000000000000, -16.21813761408365195, -13.00000000000000178 ) ) ;
#13532=CARTESIAN_POINT ( 'NONE',  ( 9.700633612364448766, 16.10095840566074799, -16.79370834700961979 ) ) ;
#13542=FILL_AREA_STYLE_COLOUR ( '', #5007 ) ;
#13544=CARTESIAN_POINT ( 'NONE',  ( 32.72003615946069743, -2.840789625746940938, -7.939653947423660263 ) ) ;
#13546=ADVANCED_FACE ( 'NONE', ( #10931 ), #1714, .T. ) ;
#13547=CARTESIAN_POINT ( 'NONE',  ( 33.28924367748503244, -4.026152426421394814, -7.939653947423662039 ) ) ;
#13562=DIRECTION ( 'NONE',  ( -0.1196152422706620172, 0.9928203230275510771, 0.000000000000000000 ) ) ;
#13563=CARTESIAN_POINT ( 'NONE',  ( 30.93831368681553684, -6.190304661545915188, -4.705209693361169343 ) ) ;
#13576=ORIENTED_EDGE ( 'NONE', *, *, #6749, .T. ) ;
#13585=ADVANCED_FACE ( 'NONE', ( #12140 ), #17721, .F. ) ;
#13587=CARTESIAN_POINT ( 'NONE',  ( 30.08145424927873535, -6.930706697444451336, -5.783357778048663356 ) ) ;
#13589=CARTESIAN_POINT ( 'NONE',  ( 31.61111609099199171, -1.710254666422835745, -5.783357778048661579 ) ) ;
#13593=CARTESIAN_POINT ( 'NONE',  ( 17.08564552898659272, -14.18688536295006664, -15.98696333172761719 ) ) ;
#13594=CARTESIAN_POINT ( 'NONE',  ( 32.87199790123699472, -1.558343308739095656, -5.783357778048663356 ) ) ;
#13595=EDGE_CURVE ( 'NONE', #8375, #5422, #3901, .T. ) ;
#13596=CARTESIAN_POINT ( 'NONE',  ( 32.32618902979206865, -6.650063623909865385, -5.783357778048669573 ) ) ;
#13599=CARTESIAN_POINT ( 'NONE',  ( 33.76207435632690590, -3.969185667289998332, -3.627061608673664672 ) ) ;
#13600=LINE ( 'NONE', #6261, #4943 ) ;
#13606=CARTESIAN_POINT ( 'NONE',  ( 26.86653773853314320, -2.919050055179571945, -6.861505862736159145 ) ) ;
#13609=CARTESIAN_POINT ( 'NONE',  ( 0.000000000000000000, 0.000000000000000000, -10.50000000000000000 ) ) ;
#13610=FACE_OUTER_BOUND ( 'NONE', #5201, .T. ) ;
#13613=CARTESIAN_POINT ( 'NONE',  ( 32.85952466860454280, -1.897204703373130741, -7.033357778048658027 ) ) ;
#13614=ADVANCED_FACE ( 'NONE', ( #169, #6970 ), #12499, .T. ) ;
#13616=CARTESIAN_POINT ( 'NONE',  ( 32.01513846370018967, -2.298745344637636912, -4.705209693361161349 ) ) ;
#13627=CARTESIAN_POINT ( 'NONE',  ( -26.79938379600875109, -11.23877132507977805, -14.03531701109484331 ) ) ;
#13628=EDGE_LOOP ( 'NONE', ( #5648, #13065, #4029, #14625 ) ) ;
#13630=ORIENTED_EDGE ( 'NONE', *, *, #16836, .T. ) ;
#13631=CARTESIAN_POINT ( 'NONE',  ( 28.93739072872572393, -3.296523698798161650, -7.939653947423660263 ) ) ;
#13633=CARTESIAN_POINT ( 'NONE',  ( 32.77709966008947617, -5.968767264923789284, -6.861505862736166250 ) ) ;
#13635=VECTOR ( 'NONE', #12141, 1000.000000000000000 ) ;
#13638=CARTESIAN_POINT ( 'NONE',  ( 28.59863824134335530, -19.00380184606325429, -13.55546330914018149 ) ) ;
#13644=EDGE_LOOP ( 'NONE', ( #12620, #8987, #13162, #2606 ) ) ;
#13650=CARTESIAN_POINT ( 'NONE',  ( 26.56758885001203652, -2.317900097157796324, -5.783357778048670461 ) ) ;
#13651=CARTESIAN_POINT ( 'NONE',  ( 30.43486631442457835, -6.877930660435475296, -5.783357778048669573 ) ) ;
#13652=AXIS2_PLACEMENT_3D ( 'NONE', #10661, #14861, #16233 ) ;
#13656=CARTESIAN_POINT ( 'NONE',  ( -5.499998817156067865, -20.49639288455253450, -6.000000000000000000 ) ) ;
#13658=EDGE_CURVE ( 'NONE', #2496, #6942, #7838, .T. ) ;
#13660=DIRECTION ( 'NONE',  ( -0.000000000000000000, -0.000000000000000000, -1.000000000000000000 ) ) ;
#13664=ORIENTED_EDGE ( 'NONE', *, *, #3245, .T. ) ;
#13665=VECTOR ( 'NONE', #4527, 1000.000000000000000 ) ;
#13671=ORIENTED_EDGE ( 'NONE', *, *, #5131, .T. ) ;
#13674=DIRECTION ( 'NONE',  ( -0.000000000000000000, 0.000000000000000000, -1.000000000000000000 ) ) ;
#13677=CARTESIAN_POINT ( 'NONE',  ( 28.82057243903374655, -7.082618055128190093, -5.783357778048668685 ) ) ;
#13680=CARTESIAN_POINT ( 'NONE',  ( 17.39700462756752231, -13.41815250082780508, -15.94071721526680108 ) ) ;
#13681=DIRECTION ( 'NONE',  ( 1.000000000000000000, 0.000000000000000000, 0.000000000000000000 ) ) ;
#13683=AXIS2_PLACEMENT_3D ( 'NONE', #10344, #16089, #14807 ) ;
#13685=CARTESIAN_POINT ( 'NONE',  ( 33.33308377457396432, -5.274811626130743392, -3.627061608673668225 ) ) ;
#13686=EDGE_CURVE ( 'NONE', #12847, #17090, #8592, .T. ) ;
#13695=ADVANCED_FACE ( 'NONE', ( #13853 ), #10030, .T. ) ;
#13696=CARTESIAN_POINT ( 'NONE',  ( 28.36401332423200827, -6.500457016816879374, -6.861505862736166250 ) ) ;
#13697=CARTESIAN_POINT ( 'NONE',  ( 25.76524775868381667, -2.816745038626284892, -5.277258820486252944 ) ) ;
#13701=DIRECTION ( 'NONE',  ( -0.1196152422706626278, 0.9928203230275510771, 0.000000000000000000 ) ) ;
#13702=LINE ( 'NONE', #16691, #12500 ) ;
#13703=VECTOR ( 'NONE', #16972, 1000.000000000000000 ) ;
#13704=CARTESIAN_POINT ( 'NONE',  ( 29.86122125502053848, -4.439161430227785310, -8.283357778048662468 ) ) ;
#13706=STYLED_ITEM ( 'NONE', ( #3931 ), #17227 ) ;
#13707=CARTESIAN_POINT ( 'NONE',  ( 33.28924367748503244, -4.026152426421394814, -7.939653947423662039 ) ) ;
#13709=DIRECTION ( 'NONE',  ( 1.000000000000000000, 0.000000000000000000, 0.000000000000000000 ) ) ;
#13710=CARTESIAN_POINT ( 'NONE',  ( 26.53943449477818106, -2.321292140958837624, -6.453230759126469707 ) ) ;
#13712=CARTESIAN_POINT ( 'NONE',  ( 26.31556265977298992, -7.384422263489805793, -5.783357778048663356 ) ) ;
#13713=EDGE_CURVE ( 'NONE', #1609, #10333, #1630, .T. ) ;
#13718=VERTEX_POINT ( 'NONE', #263 ) ;
#13719=CARTESIAN_POINT ( 'NONE',  ( 30.19827253897071273, -3.144612341114421561, -7.939653947423660263 ) ) ;
#13721=CARTESIAN_POINT ( 'NONE',  ( 32.51858583609114106, -1.611119345748072362, -5.783357778048658027 ) ) ;
#13723=CARTESIAN_POINT ( 'NONE',  ( -45.00000000000000711, 0.000000000000000000, -5.537981825772250843 ) ) ;
#13727=CARTESIAN_POINT ( 'NONE',  ( 29.77118727536321074, -5.903822331637461396, -3.283357778048667797 ) ) ;
#13733=CARTESIAN_POINT ( 'NONE',  ( 32.60321786976872005, -6.626883982076972934, -5.783357778048663356 ) ) ;
#13734=ORIENTED_EDGE ( 'NONE', *, *, #13283, .F. ) ;
#13737=EDGE_LOOP ( 'NONE', ( #12348, #12615, #13082 ) ) ;
#13738=CARTESIAN_POINT ( 'NONE',  ( -35.74085044863416272, -18.73429073671335132, -11.27079897466147607 ) ) ;
#13739=CARTESIAN_POINT ( 'NONE',  ( 31.44176105920648823, -5.502678662656354192, -3.627061608673668225 ) ) ;
#13758=VERTEX_POINT ( 'NONE', #13656 ) ;
#13760=EDGE_CURVE ( 'NONE', #10596, #1653, #1245, .T. ) ;
#13770=EDGE_CURVE ( 'NONE', #6942, #14539, #4708, .T. ) ;
#13771=CARTESIAN_POINT ( 'NONE',  ( 28.49970350196817392, -5.857138497251738407, -7.939653947423664704 ) ) ;
#13775=CARTESIAN_POINT ( 'NONE',  ( 3.248936832696172505, -15.16081378324841289, -17.00000000000000000 ) ) ;
#13779=CARTESIAN_POINT ( 'NONE',  ( 27.72904566057427189, -3.442105416578421284, -3.627061608673662896 ) ) ;
#13789=CARTESIAN_POINT ( 'NONE',  ( 28.44643833274707845, -2.428894455266221275, -7.033357778048658027 ) ) ;
#13793=DIRECTION ( 'NONE',  ( 0.9928203230275512992, 0.1196152422706614898, -0.000000000000000000 ) ) ;
#13798=DIRECTION ( 'NONE',  ( 0.9928203230275510771, 0.1196152422706614621, -0.000000000000000000 ) ) ;
#13799=CARTESIAN_POINT ( 'NONE',  ( -45.00000000000000711, -16.03270077640482683, -10.53798182577225084 ) ) ;
#13800=EDGE_LOOP ( 'NONE', ( #5562, #11245, #3794, #12383 ) ) ;
#13801=EDGE_CURVE ( 'NONE', #17553, #14662, #17386, .T. ) ;
#13802=CARTESIAN_POINT ( 'NONE',  ( 29.65098506949083301, -2.583579140294649523, -4.705209693361160461 ) ) ;
#13804=CARTESIAN_POINT ( 'NONE',  ( 26.66770885555339987, -3.370103022578743612, -8.283357778048658915 ) ) ;
#13809=CARTESIAN_POINT ( 'NONE',  ( 18.90799107099199716, -20.96007437013451380, -15.70102267215298042 ) ) ;
#13817=CYLINDRICAL_SURFACE ( 'NONE', #14182, 2.499999999999999112 ) ;
#13819=CARTESIAN_POINT ( 'NONE',  ( 33.75714020991769360, -6.487859128256953767, -5.113484796970860558 ) ) ;
#13820=CARTESIAN_POINT ( 'NONE',  ( 31.45915434921569798, -2.992700983430681028, -7.939653947423660263 ) ) ;
#13826=CIRCLE ( 'NONE', #8034, 5.000000000000000000 ) ;
#13827=CARTESIAN_POINT ( 'NONE',  ( 26.31556265977298992, -7.384422263489805793, -5.783357778048663356 ) ) ;
#13830=ORIENTED_EDGE ( 'NONE', *, *, #2968, .F. ) ;
#13832=ORIENTED_EDGE ( 'NONE', *, *, #1656, .F. ) ;
#13843=VECTOR ( 'NONE', #9025, 1000.000000000000114 ) ;
#13848=CARTESIAN_POINT ( 'NONE',  ( 24.63290760229943643, -10.17177306796459035, -14.56289668145355698 ) ) ;
#13850=CARTESIAN_POINT ( 'NONE',  ( 29.67743187657054449, -6.342216019229654833, -4.705209693361169343 ) ) ;
#13852=ORIENTED_EDGE ( 'NONE', *, *, #9496, .T. ) ;
#13853=FACE_OUTER_BOUND ( 'NONE', #16985, .T. ) ;
#13855=EDGE_CURVE ( 'NONE', #17066, #512, #4129, .T. ) ;
#13858=VERTEX_POINT ( 'NONE', #1412 ) ;
#13860=AXIS2_PLACEMENT_3D ( 'NONE', #3074, #9849, #13947 ) ;
#13861=CARTESIAN_POINT ( 'NONE',  ( 28.69037342443288452, -3.126411886501869741, -3.283357778048662023 ) ) ;
#13865=CARTESIAN_POINT ( 'NONE',  ( 9.099998387031005720, -19.29508120620799971, -12.00000000000000000 ) ) ;
#13867=ADVANCED_FACE ( 'NONE', ( #14018 ), #8567, .T. ) ;
#13872=CARTESIAN_POINT ( 'NONE',  ( 28.75424055680402802, -6.753251120556833520, -7.033357778048666908 ) ) ;
#13873=CARTESIAN_POINT ( 'NONE',  ( 30.04066231269008469, -3.163601260824890904, -7.939653947423660263 ) ) ;
#13875=FACE_OUTER_BOUND ( 'NONE', #8225, .T. ) ;
#13876=CARTESIAN_POINT ( 'NONE',  ( -45.00000000000000711, -19.03270077640482683, -10.53798182577225084 ) ) ;
#13878=ADVANCED_FACE ( 'NONE', ( #329, #15547, #3129 ), #8663, .T. ) ;
#13882=EDGE_LOOP ( 'NONE', ( #10987, #15434 ) ) ;
#13883=EDGE_LOOP ( 'NONE', ( #16075, #1991 ) ) ;
#13885=DIRECTION ( 'NONE',  ( 0.000000000000000000, 0.000000000000000000, 1.000000000000000000 ) ) ;
#13888=CARTESIAN_POINT ( 'NONE',  ( 29.56783163384821833, -3.220568019956291383, -7.939653947423660263 ) ) ;
#13891=CARTESIAN_POINT ( 'NONE',  ( 30.25533603959949502, -6.272589980291270351, -6.861505862736166250 ) ) ;
#13895=EDGE_CURVE ( 'NONE', #8205, #11419, #9114, .T. ) ;
#13896=CARTESIAN_POINT ( 'NONE',  ( 17.60442140056922611, -19.37930158608179809, -15.90915821310915135 ) ) ;
#13897=EDGE_CURVE ( 'NONE', #15676, #7696, #6209, .T. ) ;
#13898=ORIENTED_EDGE ( 'NONE', *, *, #16971, .T. ) ;
#13905=ADVANCED_FACE ( 'NONE', ( #11727, #17299 ), #10277, .T. ) ;
#13911=CARTESIAN_POINT ( 'NONE',  ( 27.25621498173240198, -3.499072175709823984, -3.627061608673662008 ) ) ;
#13913=CARTESIAN_POINT ( 'NONE',  ( -5.500000000000000888, -20.49999999999999645, -13.00000000000000178 ) ) ;
#13915=CARTESIAN_POINT ( 'NONE',  ( 30.58169613980036772, -2.898544849976259385, -3.283357778048662023 ) ) ;
#13919=CARTESIAN_POINT ( 'NONE',  ( 26.83664947211162399, -6.984282976826746037, -4.533357778048668685 ) ) ;
#13924=CIRCLE ( 'NONE', #8428, 6.249999999999996447 ) ;
#13931=ORIENTED_EDGE ( 'NONE', *, *, #9964, .F. ) ;
#13939=CYLINDRICAL_SURFACE ( 'NONE', #376, 2.749999999999992006 ) ;
#13940=CARTESIAN_POINT ( 'NONE',  ( 22.22415228291801981, -10.00312865908476567, -15.08655899088414820 ) ) ;
#13941=CARTESIAN_POINT ( 'NONE',  ( -1.917618200156724081E-28, -7.000000000000001776, -12.00000000000000000 ) ) ;
#13947=DIRECTION ( 'NONE',  ( 0.000000000000000000, 0.000000000000000000, -1.000000000000000000 ) ) ;
#13952=ORIENTED_EDGE ( 'NONE', *, *, #13760, .F. ) ;
#13958=LINE ( 'NONE', #5687, #16739 ) ;
#13959=CARTESIAN_POINT ( 'NONE',  ( -6.528882441595574626, 17.18907124314410950, -16.95629972507819971 ) ) ;
#13962=CARTESIAN_POINT ( 'NONE',  ( 32.24155699611449677, -1.634298987580965923, -5.783357778048664244 ) ) ;
#13968=CARTESIAN_POINT ( 'NONE',  ( 27.42949161418789572, -3.278323244185609830, -3.283357778048662023 ) ) ;
#13970=CARTESIAN_POINT ( 'NONE',  ( 31.51169109130924184, -2.986371343527201905, -3.627061608673662896 ) ) ;
#13973=CARTESIAN_POINT ( 'NONE',  ( -3.538288549924106796, -15.34800872113743431, -16.99955934415556769 ) ) ;
#13978=CIRCLE ( 'NONE', #6466, 2.749999999999988454 ) ;
#13986=CARTESIAN_POINT ( 'NONE',  ( 29.81239362717914787, -2.264323817775507397, -4.533357778048659803 ) ) ;
#13988=CARTESIAN_POINT ( 'NONE',  ( -22.62696978904229184, -9.966234395617776798, -15.00355996101822242 ) ) ;
#13989=EDGE_LOOP ( 'NONE', ( #12278, #8918, #5391, #10638 ) ) ;
#13990=CARTESIAN_POINT ( 'NONE',  ( 28.30694982360322953, -3.372479377640031473, -7.939653947423660263 ) ) ;
#13992=CARTESIAN_POINT ( 'NONE',  ( 29.45101334415624095, -7.006662376286320715, -5.783357778048657138 ) ) ;
#13995=CARTESIAN_POINT ( 'NONE',  ( 31.91459173804834748, -5.445711903524953712, -3.627061608673667781 ) ) ;
#13998=CARTESIAN_POINT ( 'NONE',  ( 29.32081432955537537, -3.050456207659999475, -3.283357778048662023 ) ) ;
#14005=PLANE ( 'NONE',  #9239 ) ;
#14007=CARTESIAN_POINT ( 'NONE',  ( 32.30788887834420819, -1.963665922152317833, -7.033357778048658027 ) ) ;
#14010=ADVANCED_FACE ( 'NONE', ( #4573 ), #14380, .F. ) ;
#14014=CARTESIAN_POINT ( 'NONE',  ( 27.75966235412334981, -2.811446176820259879, -4.705209693361160461 ) ) ;
#14015=CARTESIAN_POINT ( 'NONE',  ( 33.24613200752366282, -6.212066908601060256, -7.033357778048666908 ) ) ;
#14016=CARTESIAN_POINT ( 'NONE',  ( 20.00000000000000355, 7.999999999999996447, -6.000000000000000000 ) ) ;
#14018=FACE_OUTER_BOUND ( 'NONE', #4695, .T. ) ;
#14023=ORIENTED_EDGE ( 'NONE', *, *, #12859, .T. ) ;
#14027=VERTEX_POINT ( 'NONE', #15825 ) ;
#14034=CARTESIAN_POINT ( 'NONE',  ( 30.42903939560917337, -1.852671564043892660, -5.783357778048658027 ) ) ;
#14041=ORIENTED_EDGE ( 'NONE', *, *, #14215, .T. ) ;
#14042=ADVANCED_FACE ( 'NONE', ( #1123, #10709 ), #3853, .T. ) ;
#14044=CARTESIAN_POINT ( 'NONE',  ( -21.42601376483257880, 2.765314980223223529, -6.000000000000000000 ) ) ;
#14046=ORIENTED_EDGE ( 'NONE', *, *, #17551, .F. ) ;
#14049=CARTESIAN_POINT ( 'NONE',  ( 26.25801688195511474, -3.619335333876111171, -7.939653947423660263 ) ) ;
#14050=PLANE ( 'NONE',  #5154 ) ;
#14053=CARTESIAN_POINT ( 'NONE',  ( 31.67744797322171735, -2.039621600994187656, -7.033357778048658027 ) ) ;
#14059=ORIENTED_EDGE ( 'NONE', *, *, #12835, .F. ) ;
#14060=CARTESIAN_POINT ( 'NONE',  ( 28.87615734162756453, -4.557842178314484016, -7.939653947423662039 ) ) ;
#14074=CARTESIAN_POINT ( 'NONE',  ( -24.62787796620740011, -10.18046270510853368, -14.56338605435095701 ) ) ;
#14076=CARTESIAN_POINT ( 'NONE',  ( 27.67650891848073158, -3.448435056481901295, -7.939653947423660263 ) ) ;
#14077=ORIENTED_EDGE ( 'NONE', *, *, #2831, .F. ) ;
#14078=CARTESIAN_POINT ( 'NONE',  ( 31.41114436565740320, -6.133337902414513820, -4.705209693361168455 ) ) ;
#14082=( BOUNDED_CURVE ( )  B_SPLINE_CURVE ( 2, ( #13305, #4953, #981, #16047, #3277, #885, #15696, #10050, #7269 ),
 .UNSPECIFIED., .F., .T. ) 
 B_SPLINE_CURVE_WITH_KNOTS ( ( 3, 2, 2, 2, 3 ),
 ( 0.1346153846153846367, 0.1410256410256410242, 0.1538461538461538547, 0.1666666666666666574, 0.1730769230769231004 ),
 .UNSPECIFIED. ) 
 CURVE ( )  GEOMETRIC_REPRESENTATION_ITEM ( )  RATIONAL_B_SPLINE_CURVE ( ( 0.9330127018922194093, 0.9330127018922196314, 1.000000000000000000, 0.8660254037844387076, 1.000000000000000000, 0.8660254037844387076, 1.000000000000000000, 0.9330127018922190762, 0.9330127018922194093 ) ) 
 REPRESENTATION_ITEM ( '' )  );
#14083=CARTESIAN_POINT ( 'NONE',  ( 23.84191717697471091, -22.42419738538529472, -14.74207411150917757 ) ) ;
#14097=CARTESIAN_POINT ( 'NONE',  ( 33.76397967447234549, -5.422769698972272678, -8.283357778048662468 ) ) ;
#14098=CARTESIAN_POINT ( 'NONE',  ( 32.30788887834420819, -1.963665922152317833, -7.033357778048658027 ) ) ;
#14101=CARTESIAN_POINT ( 'NONE',  ( -2.016448651773435938E-27, -20.49999999999999645, -12.00000000000000000 ) ) ;
#14102=VECTOR ( 'NONE', #13445, 1000.000000000000000 ) ;
#14104=FACE_OUTER_BOUND ( 'NONE', #17614, .T. ) ;
#14105=DIRECTION ( 'NONE',  ( -0.000000000000000000, -1.000000000000000000, -0.000000000000000000 ) ) ;
#14108=EDGE_CURVE ( 'NONE', #12566, #7917, #10622, .T. ) ;
#14114=ORIENTED_EDGE ( 'NONE', *, *, #17430, .F. ) ;
#14118=CARTESIAN_POINT ( 'NONE',  ( 33.21234388421201800, -5.489230917751459771, -8.283357778048664244 ) ) ;
#14123=DIRECTION ( 'NONE',  ( -0.000000000000000000, -0.000000000000000000, 1.000000000000000000 ) ) ;
#14131=ORIENTED_EDGE ( 'NONE', *, *, #13770, .F. ) ;
#14134=ORIENTED_EDGE ( 'NONE', *, *, #12851, .T. ) ;
#14135=CARTESIAN_POINT ( 'NONE',  ( 26.18940839444933033, -6.337336286969802224, -7.823481096485427777 ) ) ;
#14139=CARTESIAN_POINT ( 'NONE',  ( 26.01652455409633902, -4.902371455920928156, -5.783357778048663356 ) ) ;
#14145=CARTESIAN_POINT ( 'NONE',  ( 28.56093688906631911, -4.595820017735426255, -3.627061608673664672 ) ) ;
#14154=VERTEX_POINT ( 'NONE', #9194 ) ;
#14158=FACE_OUTER_BOUND ( 'NONE', #9884, .T. ) ;
#14162=VECTOR ( 'NONE', #15741, 1000.000000000000227 ) ;
#14164=ORIENTED_EDGE ( 'NONE', *, *, #14556, .F. ) ;
#14165=CARTESIAN_POINT ( 'NONE',  ( 30.76748005699505129, -4.329975141788874993, -7.939653947423662039 ) ) ;
#14175=CIRCLE ( 'NONE', #12718, 14.00000000000000178 ) ;
#14179=EDGE_LOOP ( 'NONE', ( #1799, #10984 ) ) ;
#14180=DIRECTION ( 'NONE',  ( 1.000000000000000000, 0.000000000000000000, 0.000000000000000000 ) ) ;
#14181=ORIENTED_EDGE ( 'NONE', *, *, #8627, .F. ) ;
#14182=AXIS2_PLACEMENT_3D ( 'NONE', #9717, #17772, #15095 ) ;
#14186=CARTESIAN_POINT ( 'NONE',  ( 26.63392073224175505, -2.647267031729148012, -7.033357778048658027 ) ) ;
#14187=CARTESIAN_POINT ( 'NONE',  ( 27.45766530510195835, -4.728742455708699666, -3.627061608673664672 ) ) ;
#14188=ADVANCED_FACE ( 'NONE', ( #8548, #15527 ), #11066, .F. ) ;
#14189=CARTESIAN_POINT ( 'NONE',  ( 31.71123609653335507, -2.762457591843783256, -8.283357778048658915 ) ) ;
#14191=CARTESIAN_POINT ( 'NONE',  ( -1.917618200156724081E-28, -7.000000000000001776, -6.000000000000000000 ) ) ;
#14192=CARTESIAN_POINT ( 'NONE',  ( 28.51709679197739078, -3.347160818026084339, -3.627061608673662008 ) ) ;
#14195=DIRECTION ( 'NONE',  ( 0.9928203230275512992, 0.1196152422706614898, -0.000000000000000000 ) ) ;
#14200=ORIENTED_EDGE ( 'NONE', *, *, #10595, .T. ) ;
#14205=VECTOR ( 'NONE', #10049, 1000.000000000000000 ) ;
#14208=EDGE_LOOP ( 'NONE', ( #1844, #8859, #12495, #10914 ) ) ;
#14210=DIRECTION ( 'NONE',  ( 0.6000000000000001998, -0.7999999999999999334, -0.000000000000000000 ) ) ;
#14212=CARTESIAN_POINT ( 'NONE',  ( 32.53688598753899441, -6.297517047505613697, -7.033357778048666908 ) ) ;
#14215=EDGE_CURVE ( 'NONE', #5422, #496, #10113, .T. ) ;
#14216=( GEOMETRIC_REPRESENTATION_CONTEXT ( 3 ) GLOBAL_UNCERTAINTY_ASSIGNED_CONTEXT ( ( #7178 ) ) GLOBAL_UNIT_ASSIGNED_CONTEXT ( ( #10875, #16444, #2660 ) ) REPRESENTATION_CONTEXT ( 'NONE', 'WORKASPACE' ) );
#14224=CARTESIAN_POINT ( 'NONE',  ( -35.62429925076629189, -17.76690233603958546, -10.53798182577225084 ) ) ;
#14228=VERTEX_POINT ( 'NONE', #6913 ) ;
#14235=CARTESIAN_POINT ( 'NONE',  ( 29.79859849048667897, -1.928627242885762705, -5.783357778048664244 ) ) ;
#14236=CARTESIAN_POINT ( 'NONE',  ( -18.05624385570398260, -20.06430210183123464, -15.83921756800030245 ) ) ;
#14239=DIRECTION ( 'NONE',  ( 0.9899494936611662466, 0.1414213562373111965, 0.000000000000000000 ) ) ;
#14240=CIRCLE ( 'NONE', #4389, 2.749999999999992895 ) ;
#14241=FACE_OUTER_BOUND ( 'NONE', #16857, .T. ) ;
#14246=VERTEX_POINT ( 'NONE', #17922 ) ;
#14247=CARTESIAN_POINT ( 'NONE',  ( 26.99805802979993885, -6.665027654307603022, -4.705209693361168455 ) ) ;
#14249=CARTESIAN_POINT ( 'NONE',  ( 26.85044460880409645, -7.319979551716484067, -5.783357778048668685 ) ) ;
#14254=VECTOR ( 'NONE', #15064, 1000.000000000000227 ) ;
#14255=EDGE_LOOP ( 'NONE', ( #4124, #3124, #14041, #1073, #13830 ) ) ;
#14256=CARTESIAN_POINT ( 'NONE',  ( 31.26353094466156080, -6.788289799823394866, -5.783357778048663356 ) ) ;
#14257=ORIENTED_EDGE ( 'NONE', *, *, #1804, .T. ) ;
#14259=EDGE_LOOP ( 'NONE', ( #7533, #1801, #4111, #13118 ) ) ;
#14260=DIRECTION ( 'NONE',  ( -0.000000000000000000, -0.000000000000000000, -1.000000000000000000 ) ) ;
#14262=DIRECTION ( 'NONE',  ( 0.9928203230275510771, 0.1196152422706614621, -0.000000000000000000 ) ) ;
#14263=CARTESIAN_POINT ( 'NONE',  ( 27.91310269393460430, -7.181753375802955475, -5.783357778048669573 ) ) ;
#14264=ADVANCED_FACE ( 'NONE', ( #12709 ), #1579, .F. ) ;
#14265=CARTESIAN_POINT ( 'NONE',  ( 32.04158527077989760, -6.057382223572642665, -4.705209693361168455 ) ) ;
#14280=DIRECTION ( 'NONE',  ( -1.000000000000000000, 0.000000000000000000, -0.000000000000000000 ) ) ;
#14283=CARTESIAN_POINT ( 'NONE',  ( 21.42601376483257880, 2.765314980223224417, 0.000000000000000000 ) ) ;
#14288=CARTESIAN_POINT ( 'NONE',  ( 27.46709037723411839, -6.908327297984874882, -4.533357778048668685 ) ) ;
#14289=EDGE_CURVE ( 'NONE', #9007, #2012, #16627, .T. ) ;
#14290=CARTESIAN_POINT ( 'NONE',  ( 31.78252145740879797, -2.026962321187214311, -4.533357778048659803 ) ) ;
#14291=DIRECTION ( 'NONE',  ( -1.000000000000000000, 0.000000000000000000, 0.000000000000000000 ) ) ;
#14303=ORIENTED_EDGE ( 'NONE', *, *, #10791, .T. ) ;
#14306=CARTESIAN_POINT ( 'NONE',  ( 33.40745134805642635, -4.011910736534825439, -3.283357778048664688 ) ) ;
#14307=CARTESIAN_POINT ( 'NONE',  ( 26.31284730449749532, -7.327874027665321144, -6.311983372246984914 ) ) ;
#14310=AXIS2_PLACEMENT_3D ( 'NONE', #6061, #11142, #16711 ) ;
#14312=CARTESIAN_POINT ( 'NONE',  ( 25.95846283556874212, -3.455553161483297053, -8.283357778048660691 ) ) ;
#14319=EDGE_LOOP ( 'NONE', ( #11028, #3968, #6775, #17434, #4986 ) ) ;
#14320=ORIENTED_EDGE ( 'NONE', *, *, #8641, .T. ) ;
#14329=DIRECTION ( 'NONE',  ( -0.9928203230275514102, -0.1196152422706598939, 0.000000000000000000 ) ) ;
#14331=CARTESIAN_POINT ( 'NONE',  ( -17.22607755114822226, -18.63699807132245212, -15.96626374682043981 ) ) ;
#14334=CARTESIAN_POINT ( 'NONE',  ( 29.21955148510287614, -5.970283550416647600, -3.283357778048667797 ) ) ;
#14339=CARTESIAN_POINT ( 'NONE',  ( 26.34117031759772942, -2.982346454214467535, -4.705209693361161349 ) ) ;
#14341=CARTESIAN_POINT ( 'NONE',  ( 33.00219691583784964, -5.514549477365426888, -3.283357778048667797 ) ) ;
#14342=CARTESIAN_POINT ( 'NONE',  ( 26.30654288775393113, -7.309557114202778649, -5.423232652803458009 ) ) ;
#14346=ORIENTED_EDGE ( 'NONE', *, *, #7062, .F. ) ;
#14351=CARTESIAN_POINT ( 'NONE',  ( 29.30958546476020743, -4.505622649006972402, -8.283357778048662468 ) ) ;
#14355=CARTESIAN_POINT ( 'NONE',  ( 28.34209327568754233, -5.876127416962207306, -7.939653947423664704 ) ) ;
#14356=ORIENTED_EDGE ( 'NONE', *, *, #1079, .F. ) ;
#14359=CARTESIAN_POINT ( 'NONE',  ( 14.00000000000000178, 1.714505518806294835E-15, -8.700000000000001066 ) ) ;
#14364=ORIENTED_EDGE ( 'NONE', *, *, #11480, .F. ) ;
#14365=EDGE_CURVE ( 'NONE', #2915, #6589, #5968, .T. ) ;
#14370=VERTEX_POINT ( 'NONE', #8826 ) ;
#14376=EDGE_CURVE ( 'NONE', #9029, #15676, #4018, .T. ) ;
#14378=CARTESIAN_POINT ( 'NONE',  ( 28.67914455963771303, -4.581578327848842669, -8.283357778048662468 ) ) ;
#14379=PLANE ( 'NONE',  #8994 ) ;
#14380=CYLINDRICAL_SURFACE ( 'NONE', #11230, 2.000000000000001776 ) ;
#14383=CARTESIAN_POINT ( 'NONE',  ( -36.27615609941022257, -23.17738945083361557, -12.00000000000000000 ) ) ;
#14391=ORIENTED_EDGE ( 'NONE', *, *, #11713, .F. ) ;
#14392=CARTESIAN_POINT ( 'NONE',  ( 27.85662501549087366, -2.162596695673018043, -5.113484796970851676 ) ) ;
#14395=DIRECTION ( 'NONE',  ( -0.000000000000000000, -0.000000000000000000, -1.000000000000000000 ) ) ;
#14408=VECTOR ( 'NONE', #16965, 1000.000000000000000 ) ;
#14410=EDGE_CURVE ( 'NONE', #11056, #14154, #12233, .T. ) ;
#14413=CARTESIAN_POINT ( 'NONE',  ( -8.632250723006722026, -18.84644399697197770, -16.84735068286508763 ) ) ;
#14416=LINE ( 'NONE', #4439, #14408 ) ;
#14417=CARTESIAN_POINT ( 'NONE',  ( -16.79042544672876858, -17.04069398696883297, -16.02996823657058911 ) ) ;
#14426=CARTESIAN_POINT ( 'NONE',  ( 26.86653773853314320, -2.919050055179571945, -6.861505862736159145 ) ) ;
#14433=CARTESIAN_POINT ( 'NONE',  ( 26.01652455409633902, -4.902371455920928156, -5.783357778048663356 ) ) ;
#14435=CARTESIAN_POINT ( 'NONE',  ( 33.28924367748503244, -4.026152426421394814, -7.939653947423662039 ) ) ;
#14437=CARTESIAN_POINT ( 'NONE',  ( 45.00000000000000711, -19.03270077640483038, -5.537981825772250843 ) ) ;
#14442=CARTESIAN_POINT ( 'NONE',  ( 27.04606801335823718, -3.524390735323771118, -7.939653947423660263 ) ) ;
#14444=CARTESIAN_POINT ( 'NONE',  ( 26.52522735095806894, -6.721994413439005278, -4.705209693361169343 ) ) ;
#14445=EDGE_CURVE ( 'NONE', #16037, #9754, #12805, .T. ) ;
#14446=CARTESIAN_POINT ( 'NONE',  ( 28.99445422935450267, -6.424501337975009996, -6.861505862736166250 ) ) ;
#14449=CARTESIAN_POINT ( 'NONE',  ( 7.499998387031003411, -20.49508120620799900, -12.00000000000000000 ) ) ;
#14454=AXIS2_PLACEMENT_3D ( 'NONE', #2592, #8120, #1241 ) ;
#14460=DIRECTION ( 'NONE',  ( 0.000000000000000000, 0.000000000000000000, 1.000000000000000000 ) ) ;
#14462=DIRECTION ( 'NONE',  ( -1.000000000000000000, 0.000000000000000000, 0.000000000000000000 ) ) ;
#14465=CYLINDRICAL_SURFACE ( 'NONE', #6700, 2.499999999999999112 ) ;
#14469=CARTESIAN_POINT ( 'NONE',  ( 29.62480591732145996, -4.467644809586046151, -3.283357778048664688 ) ) ;
#14472=DIRECTION ( 'NONE',  ( 1.000000000000000000, 0.000000000000000000, -0.000000000000000000 ) ) ;
#14475=DIRECTION ( 'NONE',  ( -0.1196152422706620172, 0.9928203230275510771, 0.000000000000000000 ) ) ;
#14485=EDGE_LOOP ( 'NONE', ( #941, #13630, #3476, #10224 ) ) ;
#14486=CARTESIAN_POINT ( 'NONE',  ( 27.92107091181166467, -2.492190854301117753, -4.533357778048659803 ) ) ;
#14490=CARTESIAN_POINT ( 'NONE',  ( 32.82963640218302004, -5.962437625020304388, -4.705209693361169343 ) ) ;
#14505=EDGE_LOOP ( 'NONE', ( #15913, #15650, #10496, #1092 ) ) ;
#14511=CARTESIAN_POINT ( 'NONE',  ( -22.21647589440744142, -22.43199035874600966, -15.08811024704901094 ) ) ;
#14513=FACE_OUTER_BOUND ( 'NONE', #4192, .T. ) ;
#14520=ORIENTED_EDGE ( 'NONE', *, *, #12586, .T. ) ;
#14522=EDGE_CURVE ( 'NONE', #512, #11172, #17121, .T. ) ;
#14523=CARTESIAN_POINT ( 'NONE',  ( 27.50150540219088313, -5.977401655418042914, -3.627061608673667781 ) ) ;
#14531=FACE_OUTER_BOUND ( 'NONE', #6347, .T. ) ;
#14534=CARTESIAN_POINT ( 'NONE',  ( 30.01874226414561875, -2.539271660970221944, -6.861505862736159145 ) ) ;
#14539=VERTEX_POINT ( 'NONE', #9517 ) ;
#14542=CARTESIAN_POINT ( 'NONE',  ( 27.78610916120306129, -6.570083055755264745, -4.705209693361169343 ) ) ;
#14544=CARTESIAN_POINT ( 'NONE',  ( 25.77727942049545717, -5.625018267156629115, -7.939653947423662039 ) ) ;
#14547=CARTESIAN_POINT ( 'NONE',  ( 27.48088551392658729, -7.244023872874614689, -5.783357778048657138 ) ) ;
#14554=VECTOR ( 'NONE', #14630, 1000.000000000000227 ) ;
#14555=( BOUNDED_CURVE ( )  B_SPLINE_CURVE ( 2, ( #7759, #13291, #14750, #10211, #12755, #5765, #14212, #4682, #4328 ),
 .UNSPECIFIED., .F., .T. ) 
 B_SPLINE_CURVE_WITH_KNOTS ( ( 3, 2, 2, 2, 3 ),
 ( 0.1730769230769231004, 0.1794871794871794879, 0.1923076923076923184, 0.2051282051282051211, 0.2115384615384615641 ),
 .UNSPECIFIED. ) 
 CURVE ( )  GEOMETRIC_REPRESENTATION_ITEM ( )  RATIONAL_B_SPLINE_CURVE ( ( 0.9330127018922194093, 0.9330127018922196314, 1.000000000000000000, 0.8660254037844387076, 1.000000000000000000, 0.8660254037844387076, 1.000000000000000000, 0.9330127018922190762, 0.9330127018922194093 ) ) 
 REPRESENTATION_ITEM ( '' )  );
#14556=EDGE_CURVE ( 'NONE', #1336, #13453, #14970, .T. ) ;
#14560=CYLINDRICAL_SURFACE ( 'NONE', #1419, 14.00000000000000178 ) ;
#14562=APPLICATION_CONTEXT ( 'automotive_design' ) ;
#14563=DIRECTION ( 'NONE',  ( 0.000000000000000000, 1.000000000000000000, 0.000000000000000000 ) ) ;
#14566=CARTESIAN_POINT ( 'NONE',  ( 32.18597209352066812, -4.159074864394664672, -7.939653947423662039 ) ) ;
#14570=CARTESIAN_POINT ( 'NONE',  ( 28.23639288985533824, -7.542548330185622874, -5.783357778048669573 ) ) ;
#14571=CARTESIAN_POINT ( 'NONE',  ( -37.55714628004649569, -12.56174331051002113, -5.783357778048663356 ) ) ;
#14573=CARTESIAN_POINT ( 'NONE',  ( -25.11802603177690330, -16.03270077640482683, -0.5379818257722508434 ) ) ;
#14575=CARTESIAN_POINT ( 'NONE',  ( 26.31284730449749532, -7.327874027665321144, -6.311983372246984914 ) ) ;
#14578=ORIENTED_EDGE ( 'NONE', *, *, #5256, .F. ) ;
#14588=EDGE_CURVE ( 'NONE', #1845, #12756, #1015, .T. ) ;
#14590=DIRECTION ( 'NONE',  ( 0.000000000000000000, 0.000000000000000000, 1.000000000000000000 ) ) ;
#14593=CIRCLE ( 'NONE', #7053, 5.000000000000000888 ) ;
#14594=CARTESIAN_POINT ( 'NONE',  ( 33.30663696749426350, -1.516174747195733863, -5.783357778048658027 ) ) ;
#14606=EDGE_CURVE ( 'NONE', #7303, #7229, #13256, .T. ) ;
#14608=CARTESIAN_POINT ( 'NONE',  ( -20.83887142315839469, -22.08617648736154493, -15.35754594250728999 ) ) ;
#14611=DIRECTION ( 'NONE',  ( -0.000000000000000000, -0.000000000000000000, -1.000000000000000000 ) ) ;
#14614=DIRECTION ( 'NONE',  ( 0.1196152422706587976, -0.9928203230275515212, 1.866876274697368064E-15 ) ) ;
#14615=ADVANCED_FACE ( 'NONE', ( #1025 ), #6547, .F. ) ;
#14617=CARTESIAN_POINT ( 'NONE',  ( 26.47269060886452507, -6.728324053342490174, -6.861505862736166250 ) ) ;
#14622=ORIENTED_EDGE ( 'NONE', *, *, #182, .T. ) ;
#14624=CARTESIAN_POINT ( 'NONE',  ( 32.51858583609114106, -1.611119345748072362, -5.783357778048658915 ) ) ;
#14625=ORIENTED_EDGE ( 'NONE', *, *, #1056, .F. ) ;
#14627=CARTESIAN_POINT ( 'NONE',  ( 29.18947247604338102, -3.066280307211263434, -8.283357778048660691 ) ) ;
#14628=CARTESIAN_POINT ( 'NONE',  ( 26.08205926866327218, -5.446317154234562530, -8.158109112226842541 ) ) ;
#14630=DIRECTION ( 'NONE',  ( 0.9928203230275510771, 0.1196152422706614621, -0.000000000000000000 ) ) ;
#14631=CARTESIAN_POINT ( 'NONE',  ( 33.32864623319426300, -4.021405196597508613, -3.283357778048664688 ) ) ;
#14632=ADVANCED_FACE ( 'NONE', ( #8343, #13875 ), #1462, .T. ) ;
#14633=CARTESIAN_POINT ( 'NONE',  ( 27.09860475545177039, -3.518061095420291995, -3.627061608673662896 ) ) ;
#14642=CARTESIAN_POINT ( 'NONE',  ( 20.00000000000000000, 7.999999999999996447, -12.00000000000000000 ) ) ;
#14647=CARTESIAN_POINT ( 'NONE',  ( 31.54230778485832332, -2.355712103769039611, -4.705209693361160461 ) ) ;
#14649=CARTESIAN_POINT ( 'NONE',  ( 29.42969845347704450, -5.944964990802679594, -8.283357778048662468 ) ) ;
#14651=B_SPLINE_CURVE_WITH_KNOTS ( 'NONE', 3,
 ( #4725, #17559, #1016, #16165, #14628, #2208, #15988, #13071, #5077, #16080, #17176, #3559, #7642, #13247, #10248, #10598, #10332, #656 ),
 .UNSPECIFIED., .F., .F.,
 ( 4, 2, 2, 2, 2, 2, 2, 2, 4 ),
 ( 0.000000000000000000, 0.0005705796246920901435, 0.001141159249384180287, 0.001711738874076270539, 0.002282318498768360574, 0.002852898123460450609, 0.003423477748152541078, 0.003994057372844630679, 0.004564636997536721148 ),
 .UNSPECIFIED. ) ;
#14662=VERTEX_POINT ( 'NONE', #9774 ) ;
#14668=LINE ( 'NONE', #8858, #689 ) ;
#14671=CARTESIAN_POINT ( 'NONE',  ( 32.17274868998081416, -2.279756424927169345, -4.705209693361160461 ) ) ;
#14676=ADVANCED_FACE ( 'NONE', ( #5527 ), #2738, .F. ) ;
#14678=LINE ( 'NONE', #5889, #11805 ) ;
#14688=CARTESIAN_POINT ( 'NONE',  ( 23.47400307746859482, -29.47066586337335892, -14.90105725137469506 ) ) ;
#14692=CARTESIAN_POINT ( 'NONE',  ( -23.00000000000000000, -16.21813761408365195, -13.00000000000000178 ) ) ;
#14699=CARTESIAN_POINT ( 'NONE',  ( 32.17274868998081416, -2.279756424927169345, -4.705209693361160461 ) ) ;
#14709=CARTESIAN_POINT ( 'NONE',  ( 30.67110321781257909, -3.087645581983020637, -7.939653947423660263 ) ) ;
#14710=ORIENTED_EDGE ( 'NONE', *, *, #15074, .F. ) ;
#14711=CARTESIAN_POINT ( 'NONE',  ( 29.46348657678868577, -6.667800981652280967, -7.033357778048666908 ) ) ;
#14714=CARTESIAN_POINT ( 'NONE',  ( 26.31556265977298992, -7.384422263489805793, -5.783357778048663356 ) ) ;
#14715=ORIENTED_EDGE ( 'NONE', *, *, #16237, .F. ) ;
#14716=CARTESIAN_POINT ( 'NONE',  ( 32.19529564017040002, -1.250324391365404741, -5.783357778048658027 ) ) ;
#14717=AXIS2_PLACEMENT_3D ( 'NONE', #14433, #13066, #13243 ) ;
#14718=CARTESIAN_POINT ( 'NONE',  ( 28.12741954877813555, -2.767138697495831856, -6.861505862736159145 ) ) ;
#14727=VECTOR ( 'NONE', #17657, 1000.000000000000000 ) ;
#14729=CARTESIAN_POINT ( 'NONE',  ( -27.17934203385504333, -30.00000000000000355, -13.93658524716016878 ) ) ;
#14730=AXIS2_PLACEMENT_3D ( 'NONE', #1292, #13793, #6816 ) ;
#14731=ORIENTED_EDGE ( 'NONE', *, *, #4285, .T. ) ;
#14736=CARTESIAN_POINT ( 'NONE',  ( 27.41826274939272423, -4.733489685532582314, -8.283357778048662468 ) ) ;
#14748=ADVANCED_FACE ( 'NONE', ( #17905 ), #8178, .F. ) ;
#14750=CARTESIAN_POINT ( 'NONE',  ( 32.22908376348204484, -1.973160382215000785, -7.033357778048658027 ) ) ;
#14757=ORIENTED_EDGE ( 'NONE', *, *, #16135, .T. ) ;
#14758=CARTESIAN_POINT ( 'NONE',  ( -45.50000000000000000, -19.03270077640483038, -2.787981825772258837 ) ) ;
#14759=CARTESIAN_POINT ( 'NONE',  ( 31.87075164095941915, -4.197052703815608687, -3.627061608673664672 ) ) ;
#14763=CARTESIAN_POINT ( 'NONE',  ( 30.06013935859953534, -5.869009311960809328, -8.283357778048664244 ) ) ;
#14765=( BOUNDED_CURVE ( )  B_SPLINE_CURVE ( 2, ( #10464, #13197, #6119, #11647, #15745, #3225, #10367, #15829, #8668 ),
 .UNSPECIFIED., .F., .T. ) 
 B_SPLINE_CURVE_WITH_KNOTS ( ( 3, 2, 2, 2, 3 ),
 ( 0.2884615384615384914, 0.2948717948717948789, 0.3076923076923077094, 0.3205128205128205399, 0.3269230769230769273 ),
 .UNSPECIFIED. ) 
 CURVE ( )  GEOMETRIC_REPRESENTATION_ITEM ( )  RATIONAL_B_SPLINE_CURVE ( ( 0.9330127018922194093, 0.9330127018922196314, 1.000000000000000000, 0.8660254037844387076, 1.000000000000000000, 0.8660254037844387076, 1.000000000000000000, 0.9330127018922194093, 0.9330127018922194093 ) ) 
 REPRESENTATION_ITEM ( '' )  );
#14766=CARTESIAN_POINT ( 'NONE',  ( 29.37220822929407760, -7.016156836349003001, -5.783357778048668685 ) ) ;
#14767=CARTESIAN_POINT ( 'NONE',  ( 32.29295089585318834, -5.599999616269981217, -3.283357778048667797 ) ) ;
#14770=ORIENTED_EDGE ( 'NONE', *, *, #1268, .T. ) ;
#14775=DIRECTION ( 'NONE',  ( -0.000000000000000000, -0.000000000000000000, -1.000000000000000000 ) ) ;
#14780=CARTESIAN_POINT ( 'NONE',  ( -5.499998817156067865, -20.49639288455253450, -13.00000000000000178 ) ) ;
#14781=AXIS2_PLACEMENT_3D ( 'NONE', #11443, #3213, #1870 ) ;
#14786=CARTESIAN_POINT ( 'NONE',  ( 32.18597209352066812, -4.159074864394664672, -7.939653947423662039 ) ) ;
#14789=LINE ( 'NONE', #12048, #15283 ) ;
#14791=ORIENTED_EDGE ( 'NONE', *, *, #7563, .T. ) ;
#14793=CARTESIAN_POINT ( 'NONE',  ( 30.86385689617753059, -5.572304701594727128, -7.939653947423662927 ) ) ;
#14797=EDGE_CURVE ( 'NONE', #16037, #963, #10258, .T. ) ;
#14800=CARTESIAN_POINT ( 'NONE',  ( 31.03206908560819954, -5.751910973953720863, -3.283357778048667797 ) ) ;
#14801=AXIS2_PLACEMENT_3D ( 'NONE', #5882, #6983, #1730 ) ;
#14804=CARTESIAN_POINT ( 'NONE',  ( 33.17094678975809074, -2.159493266760871499, -6.861505862736159145 ) ) ;
#14807=DIRECTION ( 'NONE',  ( 1.000000000000000000, 0.000000000000000000, 0.000000000000000000 ) ) ;
#14816=CARTESIAN_POINT ( 'NONE',  ( 33.46007730730551799, -5.886481946178435010, -4.705209693361169343 ) ) ;
#14819=CARTESIAN_POINT ( 'NONE',  ( 26.63392073224175505, -2.647267031729148012, -7.033357778048658027 ) ) ;
#14831=VECTOR ( 'NONE', #11903, 1000.000000000000000 ) ;
#14836=DIRECTION ( 'NONE',  ( 0.9928203230275510771, 0.1196152422706614205, 0.000000000000000000 ) ) ;
#14839=VERTEX_POINT ( 'NONE', #17422 ) ;
#14841=DIRECTION ( 'NONE',  ( 1.000000000000000000, 0.000000000000000000, 0.000000000000000000 ) ) ;
#14842=CARTESIAN_POINT ( 'NONE',  ( 29.77797860222238313, -3.195249460342344250, -3.627061608673662008 ) ) ;
#14844=CARTESIAN_POINT ( 'NONE',  ( 30.98067518586950442, -1.786210345264705790, -5.783357778048658027 ) ) ;
#14845=EDGE_CURVE ( 'NONE', #15676, #947, #14082, .T. ) ;
#14846=CARTESIAN_POINT ( 'NONE',  ( -20.00000000000000000, 7.999999999999996447, -12.00000000000000000 ) ) ;
#14848=CARTESIAN_POINT ( 'NONE',  ( 26.39379627684682106, -4.856917663858078882, -3.283357778048664688 ) ) ;
#14850=EDGE_LOOP ( 'NONE', ( #5890, #3904, #9970, #23, #11322, #10829 ) ) ;
#14851=EDGE_LOOP ( 'NONE', ( #12103, #12116, #15677, #3905 ) ) ;
#14859=FACE_BOUND ( 'NONE', #13882, .T. ) ;
#14861=DIRECTION ( 'NONE',  ( 0.000000000000000000, 0.000000000000000000, 1.000000000000000000 ) ) ;
#14865=CARTESIAN_POINT ( 'NONE',  ( 27.25621498173240198, -3.499072175709823984, -3.627061608673662008 ) ) ;
#14868=CARTESIAN_POINT ( 'NONE',  ( 30.39102621733566423, -5.629271460726126719, -7.939653947423664704 ) ) ;
#14869=VECTOR ( 'NONE', #14395, 1000.000000000000000 ) ;
#14870=VERTEX_POINT ( 'NONE', #6417 ) ;
#14872=AXIS2_PLACEMENT_3D ( 'NONE', #10139, #10313, #1478 ) ;
#14873=ADVANCED_FACE ( 'NONE', ( #12786 ), #3616, .T. ) ;
#14876=ORIENTED_EDGE ( 'NONE', *, *, #16280, .F. ) ;
#14878=CARTESIAN_POINT ( 'NONE',  ( 30.15026255541241440, -6.285249260098253465, -4.705209693361168455 ) ) ;
#14879=EDGE_CURVE ( 'NONE', #4281, #14662, #5974, .T. ) ;
#14881=CARTESIAN_POINT ( 'NONE',  ( 33.95908713831674675, -3.945449517755636126, -5.783357778048663356 ) ) ;
#14882=CARTESIAN_POINT ( 'NONE',  ( 28.58911057998038885, -6.046239229258517867, -3.283357778048667797 ) ) ;
#14884=CARTESIAN_POINT ( 'NONE',  ( 32.57067411085063924, -7.020353038355215070, -5.783357778048669573 ) ) ;
#14886=CARTESIAN_POINT ( 'NONE',  ( 33.42946061375642586, -6.517141185936593750, -5.783357778048668685 ) ) ;
#14888=CARTESIAN_POINT ( 'NONE',  ( 30.35023428074701002, -1.862166024106576057, -5.783357778048664244 ) ) ;
#14891=EDGE_CURVE ( 'NONE', #9479, #5360, #7605, .T. ) ;
#14893=EDGE_CURVE ( 'NONE', #7696, #6789, #7159, .T. ) ;
#14894=ORIENTED_EDGE ( 'NONE', *, *, #16135, .F. ) ;
#14898=CARTESIAN_POINT ( 'NONE',  ( -27.54501800341186168, -11.92321325334030568, -13.84074570522889047 ) ) ;
#14901=CARTESIAN_POINT ( 'NONE',  ( 33.32855701603872234, -2.140504347050403045, -6.861505862736158257 ) ) ;
#14903=CARTESIAN_POINT ( 'NONE',  ( 26.94172295629870462, -6.971623697019761146, -7.033357778048666908 ) ) ;
#14908=CARTESIAN_POINT ( 'NONE',  ( 29.03578327489625011, -17.85349083735938081, -13.43326801114178615 ) ) ;
#14916=EDGE_CURVE ( 'NONE', #10596, #12847, #16131, .T. ) ;
#14917=EDGE_LOOP ( 'NONE', ( #10108, #669, #2415, #15715 ) ) ;
#14919=EDGE_LOOP ( 'NONE', ( #12432, #15850, #9168, #708 ) ) ;
#14922=ORIENTED_EDGE ( 'NONE', *, *, #14845, .F. ) ;
#14924=CARTESIAN_POINT ( 'NONE',  ( 29.78250536075762867, -6.329556739422670830, -6.861505862736167138 ) ) ;
#14926=CARTESIAN_POINT ( 'NONE',  ( 30.57046727500519978, -4.353711291323232757, -8.283357778048662468 ) ) ;
#14936=ORIENTED_EDGE ( 'NONE', *, *, #11713, .T. ) ;
#14937=ORIENTED_EDGE ( 'NONE', *, *, #11055, .T. ) ;
#14940=EDGE_CURVE ( 'NONE', #7031, #12145, #8615, .T. ) ;
#14945=CARTESIAN_POINT ( 'NONE',  ( 29.71979337562451207, -1.938121702948446323, -5.783357778048664244 ) ) ;
#14947=DIRECTION ( 'NONE',  ( 0.7999999999999999334, -0.6000000000000001998, 0.000000000000000000 ) ) ;
#14950=CARTESIAN_POINT ( 'NONE',  ( 28.68570264635560463, -13.61469575198669624, -13.53129406029897730 ) ) ;
#14952=CARTESIAN_POINT ( 'NONE',  ( 31.67382807612511542, -6.101689702897060030, -6.861505862736167138 ) ) ;
#14956=DIRECTION ( 'NONE',  ( -1.000000000000000000, 0.000000000000000000, 0.000000000000000000 ) ) ;
#14959=CARTESIAN_POINT ( 'NONE',  ( 28.73594040535617467, -2.066853418799292630, -5.783357778048658915 ) ) ;
#14964=PLANE ( 'NONE',  #4679 ) ;
#14966=CARTESIAN_POINT ( 'NONE',  ( 33.16732689266149237, -6.221561368663743430, -7.033357778048666908 ) ) ;
#14968=CARTESIAN_POINT ( 'NONE',  ( 31.91006497951310550, -2.311404624444611589, -6.861505862736159145 ) ) ;
#14970=LINE ( 'NONE', #3736, #12936 ) ;
#14979=CARTESIAN_POINT ( 'NONE',  ( 13.00000000000000178, 0.000000000000000000, -8.700000000000001066 ) ) ;
#14981=AXIS2_PLACEMENT_3D ( 'NONE', #17533, #15955, #2090 ) ;
#14982=CARTESIAN_POINT ( 'NONE',  ( 29.97942892559193950, -4.424919740341219487, -3.627061608673664672 ) ) ;
#14986=CARTESIAN_POINT ( 'NONE',  ( 32.65880277236253448, -4.102108105263264193, -7.939653947423662039 ) ) ;
#14999=ORIENTED_EDGE ( 'NONE', *, *, #2122, .F. ) ;
#15001=ADVANCED_FACE ( 'NONE', ( #9389 ), #8218, .F. ) ;
#15005=CARTESIAN_POINT ( 'NONE',  ( 28.39010325924584421, -2.735490497978389612, -4.705209693361160461 ) ) ;
#15006=CARTESIAN_POINT ( 'NONE',  ( 30.72436838703367812, -6.515889623968540434, -7.033357778048666908 ) ) ;
#15012=CARTESIAN_POINT ( 'NONE',  ( 27.30498922523054617, -2.229057914452205136, -5.113484796970851676 ) ) ;
#15034=CARTESIAN_POINT ( 'NONE',  ( 20.84129949943806537, -10.34926000617958231, -15.35708546568073984 ) ) ;
#15037=CARTESIAN_POINT ( 'NONE',  ( 30.15443244188179150, -1.895953141405084086, -5.783357778048658027 ) ) ;
#15038=EDGE_CURVE ( 'NONE', #11629, #8286, #15195, .T. ) ;
#15048=CARTESIAN_POINT ( 'NONE',  ( 28.99445422935450267, -6.424501337975009996, -6.861505862736166250 ) ) ;
#15050=CARTESIAN_POINT ( 'NONE',  ( 25.94006848055682113, -4.267777217026356595, -3.719179227265282162 ) ) ;
#15055=EDGE_CURVE ( 'NONE', #15308, #1845, #8298, .T. ) ;
#15058=CARTESIAN_POINT ( 'NONE',  ( 28.60033944477555323, -4.591072787911525843, -8.283357778048662468 ) ) ;
#15059=CARTESIAN_POINT ( 'NONE',  ( 32.77257290155422709, -2.834459985843461816, -3.627061608673662896 ) ) ;
#15062=CARTESIAN_POINT ( 'NONE',  ( 26.56758885001203652, -2.317900097157796324, -5.783357778048670461 ) ) ;
#15064=DIRECTION ( 'NONE',  ( 0.9928203230275510771, 0.1196152422706614621, -0.000000000000000000 ) ) ;
#15074=EDGE_CURVE ( 'NONE', #9208, #16590, #9307, .T. ) ;
#15075=CARTESIAN_POINT ( 'NONE',  ( 28.40332666278570173, -4.614808937445885384, -7.939653947423662039 ) ) ;
#15078=PLANE ( 'NONE',  #4678 ) ;
#15080=CARTESIAN_POINT ( 'NONE',  ( 33.38562051666750818, -5.268481986227246061, -7.939653947423664704 ) ) ;
#15084=CIRCLE ( 'NONE', #7573, 2.499999999999998668 ) ;
#15087=CARTESIAN_POINT ( 'NONE',  ( 19.23308179030308551, -21.22208063239337505, -15.64628783324453387 ) ) ;
#15091=CARTESIAN_POINT ( 'NONE',  ( -20.25000000000001066, -16.21813761408365195, -13.00000000000000355 ) ) ;
#15093=VECTOR ( 'NONE', #11268, 1000.000000000000227 ) ;
#15095=DIRECTION ( 'NONE',  ( -0.1196152422706611984, 0.9928203230275510771, 0.000000000000000000 ) ) ;
#15097=CARTESIAN_POINT ( 'NONE',  ( 28.28502977505876359, -2.748149777785362957, -6.861505862736158257 ) ) ;
#15114=CYLINDRICAL_SURFACE ( 'NONE', #3259, 2.749999999999992006 ) ;
#15117=( BOUNDED_CURVE ( )  B_SPLINE_CURVE ( 2, ( #15853, #3787, #7957, #14767, #3425, #17423, #10569, #13218, #2175 ),
 .UNSPECIFIED., .F., .T. ) 
 B_SPLINE_CURVE_WITH_KNOTS ( ( 3, 2, 2, 2, 3 ),
 ( 0.2115384615384615641, 0.2179487179487179516, 0.2307692307692307820, 0.2435897435897435848, 0.2500000000000000000 ),
 .UNSPECIFIED. ) 
 CURVE ( )  GEOMETRIC_REPRESENTATION_ITEM ( )  RATIONAL_B_SPLINE_CURVE ( ( 0.9330127018922194093, 0.9330127018922196314, 1.000000000000000000, 0.8660254037844387076, 1.000000000000000000, 0.8660254037844387076, 1.000000000000000000, 0.9330127018922191873, 0.9330127018922194093 ) ) 
 REPRESENTATION_ITEM ( '' )  );
#15120=CARTESIAN_POINT ( 'NONE',  ( 33.73390066541284682, -2.518766455766908940, -3.283357778048662023 ) ) ;
#15122=LINE ( 'NONE', #8231, #5242 ) ;
#15123=ORIENTED_EDGE ( 'NONE', *, *, #5209, .F. ) ;
#15126=CARTESIAN_POINT ( 'NONE',  ( 20.27684169284606241, -10.57794632788464995, -15.46227570229628689 ) ) ;
#15131=VECTOR ( 'NONE', #1463, 1000.000000000000000 ) ;
#15132=CARTESIAN_POINT ( 'NONE',  ( 27.67650891848073158, -3.448435056481901295, -7.939653947423660263 ) ) ;
#15137=AXIS2_PLACEMENT_3D ( 'NONE', #10107, #4412, #9925 ) ;
#15138=EDGE_CURVE ( 'NONE', #12549, #3497, #2955, .T. ) ;
#15142=CARTESIAN_POINT ( 'NONE',  ( 29.62036837594175154, -3.214238380052812261, -3.627061608673662896 ) ) ;
#15148=ADVANCED_FACE ( 'NONE', ( #14104 ), #10005, .F. ) ;
#15149=CARTESIAN_POINT ( 'NONE',  ( 13.00000000000000178, 0.000000000000000000, -12.00000000000000000 ) ) ;
#15152=CARTESIAN_POINT ( 'NONE',  ( 29.38468146192651886, -6.677295441714964142, -7.033357778048666908 ) ) ;
#15155=CARTESIAN_POINT ( 'NONE',  ( 33.40301380667672504, -2.758504307001591549, -3.627061608673662896 ) ) ;
#15157=CARTESIAN_POINT ( 'NONE',  ( -25.11802603177690330, -19.03270077640483038, -0.5379818257722508434 ) ) ;
#15162=ORIENTED_EDGE ( 'NONE', *, *, #14289, .T. ) ;
#15168=ORIENTED_EDGE ( 'NONE', *, *, #7915, .F. ) ;
#15170=CARTESIAN_POINT ( 'NONE',  ( 31.43723430067123914, -2.368371383576012956, -6.861505862736158257 ) ) ;
#15173=CARTESIAN_POINT ( 'NONE',  ( 32.01513846370018967, -2.298745344637636912, -4.705209693361161349 ) ) ;
#15181=CARTESIAN_POINT ( 'NONE',  ( -2.016448651773435938E-27, -20.49999999999999645, -13.00000000000000355 ) ) ;
#15187=CARTESIAN_POINT ( 'NONE',  ( 31.56875459193803124, -6.114348982704044921, -4.705209693361169343 ) ) ;
#15195=LINE ( 'NONE', #10824, #10186 ) ;
#15196=DIRECTION ( 'NONE',  ( -1.000000000000000000, 0.000000000000000000, 0.000000000000000000 ) ) ;
#15205=DIRECTION ( 'NONE',  ( -0.000000000000000000, -0.000000000000000000, -1.000000000000000000 ) ) ;
#15215=CARTESIAN_POINT ( 'NONE',  ( 29.14753769709988518, -3.271205139184214516, -3.627061608673662008 ) ) ;
#15217=DIRECTION ( 'NONE',  ( 0.000000000000000000, 1.000000000000000000, 0.000000000000000000 ) ) ;
#15222=( BOUNDED_CURVE ( )  B_SPLINE_CURVE ( 2, ( #2435, #17693, #10735, #16309, #2510, #144, #2956, #7225, #9823 ),
 .UNSPECIFIED., .F., .T. ) 
 B_SPLINE_CURVE_WITH_KNOTS ( ( 3, 2, 2, 2, 3 ),
 ( 0.2884615384615384914, 0.2948717948717948789, 0.3076923076923077094, 0.3205128205128205399, 0.3269230769230769273 ),
 .UNSPECIFIED. ) 
 CURVE ( )  GEOMETRIC_REPRESENTATION_ITEM ( )  RATIONAL_B_SPLINE_CURVE ( ( 0.9330127018922194093, 0.9330127018922196314, 1.000000000000000000, 0.8660254037844387076, 1.000000000000000000, 0.8660254037844387076, 1.000000000000000000, 0.9330127018922194093, 0.9330127018922194093 ) ) 
 REPRESENTATION_ITEM ( '' )  );
#15227=CARTESIAN_POINT ( 'NONE',  ( -15.92260893619738837, -28.39189527176317540, -6.000000000000000000 ) ) ;
#15233=CARTESIAN_POINT ( 'NONE',  ( 27.17934203385504333, -30.00000000000000355, -13.93658524716016878 ) ) ;
#15234=CARTESIAN_POINT ( 'NONE',  ( 26.66018910156667232, -2.644102211984857842, -4.533357778048659803 ) ) ;
#15236=CARTESIAN_POINT ( 'NONE',  ( 31.27962407439061110, -2.387360303286481855, -6.861505862736159145 ) ) ;
#15238=CARTESIAN_POINT ( 'NONE',  ( -23.00000000000000000, -16.21813761408365195, -13.00000000000000355 ) ) ;
#15242=ORIENTED_EDGE ( 'NONE', *, *, #7066, .T. ) ;
#15248=CARTESIAN_POINT ( 'NONE',  ( 31.55553118839817728, -4.235030543236534939, -7.939653947423662039 ) ) ;
#15249=CARTESIAN_POINT ( 'NONE',  ( -8.632250723006722026, -18.84644399697197770, -16.84735068286508763 ) ) ;
#15253=CARTESIAN_POINT ( 'NONE',  ( 30.75425665345519732, -2.450656702321377001, -4.705209693361161349 ) ) ;
#15254=CARTESIAN_POINT ( 'NONE',  ( 45.00000000000000711, -16.03270077640482683, -5.537981825772250843 ) ) ;
#15258=ORIENTED_EDGE ( 'NONE', *, *, #8527, .F. ) ;
#15261=AXIS2_PLACEMENT_3D ( 'NONE', #487, #4470, #17000 ) ;
#15270=CARTESIAN_POINT ( 'NONE',  ( 25.96860978910007844, -6.167287525404733017, -7.540302725459484989 ) ) ;
#15271=ADVANCED_FACE ( 'NONE', ( #11259 ), #9822, .F. ) ;
#15283=VECTOR ( 'NONE', #12322, 1000.000000000000227 ) ;
#15285=EDGE_CURVE ( 'NONE', #17574, #11056, #6663, .T. ) ;
#15287=DIRECTION ( 'NONE',  ( -1.000000000000000000, 0.000000000000000000, 0.000000000000000000 ) ) ;
#15300=CARTESIAN_POINT ( 'NONE',  ( 28.40059689994085801, -13.06564623954105464, -13.61006631438115200 ) ) ;
#15304=AXIS2_PLACEMENT_3D ( 'NONE', #5241, #10762, #16340 ) ;
#15307=VECTOR ( 'NONE', #1322, 1000.000000000000000 ) ;
#15308=VERTEX_POINT ( 'NONE', #11822 ) ;
#15315=CARTESIAN_POINT ( 'NONE',  ( -3.248936832696171617, 17.78798921770683350, -17.00000000000000000 ) ) ;
#15316=DIRECTION ( 'NONE',  ( 1.000000000000000000, 0.000000000000000000, 0.000000000000000000 ) ) ;
#15318=LINE ( 'NONE', #11206, #2934 ) ;
#15319=LINE ( 'NONE', #15149, #13 ) ;
#15321=DIRECTION ( 'NONE',  ( -0.7681011886108269904, -0.5760758914581204371, -0.2795659695588260107 ) ) ;
#15323=CARTESIAN_POINT ( 'NONE',  ( 27.52714686987067694, -7.627998469090175426, -5.783357778048669573 ) ) ;
#15324=CARTESIAN_POINT ( 'NONE',  ( 30.12381574833269937, -2.526612381163247267, -4.705209693361161349 ) ) ;
#15325=CARTESIAN_POINT ( 'NONE',  ( 23.00000000000000000, -16.21813761408365195, -13.00000000000000355 ) ) ;
#15328=( BOUNDED_CURVE ( )  B_SPLINE_CURVE ( 2, ( #5635, #10976, #1669, #13727, #9895, #13998, #17926, #3028, #5458 ),
 .UNSPECIFIED., .F., .T. ) 
 B_SPLINE_CURVE_WITH_KNOTS ( ( 3, 2, 2, 2, 3 ),
 ( 0.5192307692307692735, 0.5256410256410256610, 0.5384615384615384359, 0.5512820512820513219, 0.5576923076923077094 ),
 .UNSPECIFIED. ) 
 CURVE ( )  GEOMETRIC_REPRESENTATION_ITEM ( )  RATIONAL_B_SPLINE_CURVE ( ( 0.9330127018922192983, 0.9330127018922198534, 1.000000000000000000, 0.8660254037844387076, 1.000000000000000000, 0.8660254037844387076, 1.000000000000000000, 0.9330127018922194093, 0.9330127018922194093 ) ) 
 REPRESENTATION_ITEM ( '' )  );
#15329=CARTESIAN_POINT ( 'NONE',  ( 16.75000000000000000, -16.21813761408365195, -13.00000000000000178 ) ) ;
#15333=EDGE_LOOP ( 'NONE', ( #15986, #7836, #6333, #1753 ) ) ;
#15335=VERTEX_POINT ( 'NONE', #6118 ) ;
#15338=CARTESIAN_POINT ( 'NONE',  ( -34.91377932259078420, -11.86950488720510322, -11.57182824616228878 ) ) ;
#15341=CARTESIAN_POINT ( 'NONE',  ( 30.93831368681553684, -6.190304661545915188, -4.705209693361169343 ) ) ;
#15344=VERTEX_POINT ( 'NONE', #7581 ) ;
#15345=CARTESIAN_POINT ( 'NONE',  ( 29.62489513447700062, -6.348545659133139729, -6.861505862736166250 ) ) ;
#15347=CYLINDRICAL_SURFACE ( 'NONE', #16159, 5.000000000000000000 ) ;
#15348=VERTEX_POINT ( 'NONE', #14575 ) ;
#15351=ORIENTED_EDGE ( 'NONE', *, *, #8540, .F. ) ;
#15352=CARTESIAN_POINT ( 'NONE',  ( 21.62682814333776804, -22.31876753225984800, -15.20565444446567227 ) ) ;
#15353=ORIENTED_EDGE ( 'NONE', *, *, #3672, .F. ) ;
#15363=ORIENTED_EDGE ( 'NONE', *, *, #3123, .T. ) ;
#15365=AXIS2_PLACEMENT_3D ( 'NONE', #7378, #9785, #13885 ) ;
#15366=AXIS2_PLACEMENT_3D ( 'NONE', #14571, #2149, #9193 ) ;
#15367=CARTESIAN_POINT ( 'NONE',  ( 27.23882169172318513, -6.009049854935478052, -7.939653947423664704 ) ) ;
#15372=VECTOR ( 'NONE', #4613, 1000.000000000000000 ) ;
#15386=VECTOR ( 'NONE', #17010, 1000.000000000000227 ) ;
#15390=CARTESIAN_POINT ( 'NONE',  ( 27.38828526237195504, -6.917821758047558056, -4.533357778048668685 ) ) ;
#15403=VECTOR ( 'NONE', #3753, 1000.000000000000227 ) ;
#15404=ORIENTED_EDGE ( 'NONE', *, *, #2607, .F. ) ;
#15409=CARTESIAN_POINT ( 'NONE',  ( 26.24062359194589433, -6.129313013101782559, -3.627061608673667781 ) ) ;
#15414=CARTESIAN_POINT ( 'NONE',  ( 32.00093131988006689, -6.699447617117800569, -6.453230759126470595 ) ) ;
#15419=CARTESIAN_POINT ( 'NONE',  ( 27.29063000668916672, -2.568146533142987575, -4.533357778048659803 ) ) ;
#15421=CARTESIAN_POINT ( 'NONE',  ( 28.77978050244509944, -3.315512618508630993, -7.939653947423660263 ) ) ;
#15425=CARTESIAN_POINT ( 'NONE',  ( -34.91600907648203389, -11.88801210197604341, 0.000000000000000000 ) ) ;
#15426=AXIS2_PLACEMENT_3D ( 'NONE', #17854, #10893, #16462 ) ;
#15430=ORIENTED_EDGE ( 'NONE', *, *, #14797, .F. ) ;
#15432=LINE ( 'NONE', #4457, #9628 ) ;
#15434=ORIENTED_EDGE ( 'NONE', *, *, #3039, .T. ) ;
#15435=CARTESIAN_POINT ( 'NONE',  ( -17.71052479140136526, -12.88256812061772116, -15.89289657457836746 ) ) ;
#15437=ORIENTED_EDGE ( 'NONE', *, *, #2717, .F. ) ;
#15438=CARTESIAN_POINT ( 'NONE',  ( 28.08810621022444920, -4.652786776866828511, -3.627061608673664672 ) ) ;
#15440=EDGE_CURVE ( 'NONE', #17849, #11176, #11730, .T. ) ;
#15441=CARTESIAN_POINT ( 'NONE',  ( 29.99682221560115991, -1.914942061115552541, -5.783357778048658027 ) ) ;
#15455=CARTESIAN_POINT ( 'NONE',  ( 8.968924017731504605, -19.12031538047531853, -16.82773324567541451 ) ) ;
#15457=CARTESIAN_POINT ( 'NONE',  ( 26.94172295629870462, -6.971623697019761146, -7.033357778048666908 ) ) ;
#15458=CARTESIAN_POINT ( 'NONE',  ( 33.79776779778399032, -6.145605689821873163, -7.033357778048666908 ) ) ;
#15460=CARTESIAN_POINT ( 'NONE',  ( 31.35480929215617252, -6.439933945126671055, -7.033357778048666908 ) ) ;
#15468=CARTESIAN_POINT ( 'NONE',  ( 26.47260139170898441, -4.847423203795396596, -3.283357778048664688 ) ) ;
#15472=ORIENTED_EDGE ( 'NONE', *, *, #10585, .T. ) ;
#15483=DIRECTION ( 'NONE',  ( 1.000000000000000000, 0.000000000000000000, 0.000000000000000000 ) ) ;
#15494=ADVANCED_FACE ( 'NONE', ( #5318, #10841 ), #16407, .T. ) ;
#15499=CARTESIAN_POINT ( 'NONE',  ( 29.27960797773944179, -6.689954721521948144, -4.533357778048668685 ) ) ;
#15501=CARTESIAN_POINT ( 'NONE',  ( -18.96667930129623514, 9.308258642545592210, -15.69246997591053017 ) ) ;
#15504=CARTESIAN_POINT ( 'NONE',  ( 20.25000000000000711, -16.21813761408365195, -13.00000000000000178 ) ) ;
#15507=UNCERTAINTY_MEASURE_WITH_UNIT (LENGTH_MEASURE( 1.000000000000000082E-05 ), #16275, 'distance_accuracy_value', 'NONE');
#15509=CARTESIAN_POINT ( 'NONE',  ( 30.65370992780335868, -5.597623261208691581, -3.627061608673667781 ) ) ;
#15512=CARTESIAN_POINT ( 'NONE',  ( 26.27285561281999193, -7.029948842322393254, -4.710679390969556124 ) ) ;
#15514=DIRECTION ( 'NONE',  ( -0.000000000000000000, -0.000000000000000000, -1.000000000000000000 ) ) ;
#15522=VERTEX_POINT ( 'NONE', #15661 ) ;
#15523=CARTESIAN_POINT ( 'NONE',  ( 25.78291734803729796, -2.627872734613073913, -5.430426774474530482 ) ) ;
#15525=CARTESIAN_POINT ( 'NONE',  ( 28.87615734162756453, -4.557842178314484016, -7.939653947423662039 ) ) ;
#15526=CARTESIAN_POINT ( 'NONE',  ( 45.50000000000000000, -16.03270077640482683, -5.537981825772250843 ) ) ;
#15527=FACE_BOUND ( 'NONE', #10330, .T. ) ;
#15528=CARTESIAN_POINT ( 'NONE',  ( -45.00000000000000711, -16.03270077640482683, -5.537981825772250843 ) ) ;
#15530=CARTESIAN_POINT ( 'NONE',  ( -20.00000000000000000, 7.999999999999996447, -12.00000000000000000 ) ) ;
#15536=VERTEX_POINT ( 'NONE', #17034 ) ;
#15537=DIRECTION ( 'NONE',  ( 0.000000000000000000, 0.000000000000000000, 1.000000000000000000 ) ) ;
#15538=ORIENTED_EDGE ( 'NONE', *, *, #3003, .F. ) ;
#15540=VERTEX_POINT ( 'NONE', #3333 ) ;
#15542=CARTESIAN_POINT ( 'NONE',  ( 26.65222088368961195, -7.333664733486695120, -5.783357778048669573 ) ) ;
#15543=CARTESIAN_POINT ( 'NONE',  ( 30.88568772756644520, -4.315733451902305617, -3.283357778048664688 ) ) ;
#15547=FACE_OUTER_BOUND ( 'NONE', #17684, .T. ) ;
#15549=CARTESIAN_POINT ( 'NONE',  ( 29.52399153675929355, -1.971908820246954130, -5.783357778048658027 ) ) ;
#15550=LINE ( 'NONE', #8483, #15995 ) ;
#15560=DIRECTION ( 'NONE',  ( -1.000000000000000000, 0.000000000000000000, 0.000000000000000000 ) ) ;
#15569=ORIENTED_EDGE ( 'NONE', *, *, #11669, .T. ) ;
#15579=ORIENTED_EDGE ( 'NONE', *, *, #7902, .F. ) ;
#15585=CARTESIAN_POINT ( 'NONE',  ( 33.60446413004628141, -3.988174587000466342, -3.627061608673664672 ) ) ;
#15587=CARTESIAN_POINT ( 'NONE',  ( -11.90182750357594621, 14.98910623166845646, -16.60584412753037853 ) ) ;
#15588=CARTESIAN_POINT ( 'NONE',  ( -28.39989834181360706, -19.37183319909320645, -13.61025820885934223 ) ) ;
#15593=DIRECTION ( 'NONE',  ( -0.000000000000000000, -0.000000000000000000, -1.000000000000000000 ) ) ;
#15594=CARTESIAN_POINT ( 'NONE',  ( -23.02601376483258022, 3.965314980223224151, -6.000000000000000000 ) ) ;
#15598=CARTESIAN_POINT ( 'NONE',  ( 29.49337484321020497, -2.602568060005117090, -4.705209693361161349 ) ) ;
#15600=CARTESIAN_POINT ( 'NONE',  ( -2.016448651773435938E-27, -20.49999999999999645, -13.00000000000000178 ) ) ;
#15601=CARTESIAN_POINT ( 'NONE',  ( 26.00079723459025871, -4.771832887959356562, -3.592817407220987747 ) ) ;
#15603=( BOUNDED_CURVE ( )  B_SPLINE_CURVE ( 3, ( #17441, #16062, #8626, #12435 ),
 .UNSPECIFIED., .F., .T. ) 
 B_SPLINE_CURVE_WITH_KNOTS ( ( 4, 4 ),
 ( 1.221730476396036824, 1.230954889131919305 ),
 .UNSPECIFIED. ) 
 CURVE ( )  GEOMETRIC_REPRESENTATION_ITEM ( )  RATIONAL_B_SPLINE_CURVE ( ( 1.000000000000000000, 0.9999929091967096895, 0.9999929091967096895, 1.000000000000000000 ) ) 
 REPRESENTATION_ITEM ( '' )  );
#15605=PLANE ( 'NONE',  #1375 ) ;
#15606=VERTEX_POINT ( 'NONE', #4591 ) ;
#15608=EDGE_LOOP ( 'NONE', ( #8823, #16680, #9684, #10321 ) ) ;
#15611=CARTESIAN_POINT ( 'NONE',  ( -16.75000000000000355, -15.80559819018441381, -16.03574476417185934 ) ) ;
#15612=VERTEX_POINT ( 'NONE', #349 ) ;
#15613=CARTESIAN_POINT ( 'NONE',  ( -45.00000000000000711, -16.03270077640482683, -0.5379818257722508434 ) ) ;
#15617=CARTESIAN_POINT ( 'NONE',  ( 30.02326902268086428, -5.673578940050561847, -3.627061608673667781 ) ) ;
#15618=CARTESIAN_POINT ( 'NONE',  ( 27.96989853965305528, -4.667028466753395222, -8.283357778048662468 ) ) ;
#15622=AXIS2_PLACEMENT_3D ( 'NONE', #6244, #10406, #2271 ) ;
#15634=ORIENTED_EDGE ( 'NONE', *, *, #6450, .F. ) ;
#15638=ORIENTED_EDGE ( 'NONE', *, *, #13658, .T. ) ;
#15640=CARTESIAN_POINT ( 'NONE',  ( 32.34167700165585302, -2.686501913001913433, -8.283357778048658915 ) ) ;
#15641=CARTESIAN_POINT ( 'NONE',  ( 26.64639396487419987, -2.308405637095112706, -5.783357778048658027 ) ) ;
#15649=AXIS2_PLACEMENT_3D ( 'NONE', #9341, #6621, #9424 ) ;
#15650=ORIENTED_EDGE ( 'NONE', *, *, #9344, .T. ) ;
#15656=CARTESIAN_POINT ( 'NONE',  ( 26.15738093914773543, -4.885401043216321959, -8.283357778048662468 ) ) ;
#15661=CARTESIAN_POINT ( 'NONE',  ( 3.538288549924106796, -15.34800872113743431, -13.00000000000000178 ) ) ;
#15662=CARTESIAN_POINT ( 'NONE',  ( 25.90899358965569022, -2.397247819800704782, -6.453230759126464378 ) ) ;
#15674=AXIS2_PLACEMENT_3D ( 'NONE', #10852, #6972, #6876 ) ;
#15676=VERTEX_POINT ( 'NONE', #3685 ) ;
#15677=ORIENTED_EDGE ( 'NONE', *, *, #17640, .F. ) ;
#15678=VERTEX_POINT ( 'NONE', #13391 ) ;
#15681=DIRECTION ( 'NONE',  ( 0.6000000000000001998, -0.7999999999999999334, 0.000000000000000000 ) ) ;
#15683=CARTESIAN_POINT ( 'NONE',  ( -24.42841412577760352, -22.30604244805903136, -14.60923613736931514 ) ) ;
#15685=CARTESIAN_POINT ( 'NONE',  ( 31.98525019727866692, -6.363978266284800789, -7.033357778048666908 ) ) ;
#15691=CARTESIAN_POINT ( 'NONE',  ( 25.92467471225709374, -2.732717170633701453, -7.033357778048658027 ) ) ;
#15694=CARTESIAN_POINT ( 'NONE',  ( 28.34209327568754233, -5.876127416962207306, -7.939653947423664704 ) ) ;
#15695=CARTESIAN_POINT ( 'NONE',  ( 5.499998817156068753, -20.49639288455253450, -12.00000000000000000 ) ) ;
#15696=CARTESIAN_POINT ( 'NONE',  ( 32.33415724766913257, -1.960501102408027219, -4.533357778048659803 ) ) ;
#15697=CARTESIAN_POINT ( 'NONE',  ( 26.13631296615022137, -5.896629108145342357, -3.732065232213778394 ) ) ;
#15702=CIRCLE ( 'NONE', #16559, 5.500000000000000000 ) ;
#15703=ORIENTED_EDGE ( 'NONE', *, *, #6215, .T. ) ;
#15706=ORIENTED_EDGE ( 'NONE', *, *, #3300, .F. ) ;
#15707=VECTOR ( 'NONE', #4226, 1000.000000000000227 ) ;
#15708=CARTESIAN_POINT ( 'NONE',  ( 23.00000000000000000, -16.21813761408365195, 0.000000000000000000 ) ) ;
#15709=ORIENTED_EDGE ( 'NONE', *, *, #5828, .T. ) ;
#15711=CARTESIAN_POINT ( 'NONE',  ( 26.39370705969127684, -2.976016814310973313, -6.861505862736158257 ) ) ;
#15713=CARTESIAN_POINT ( 'NONE',  ( 27.78610916120306129, -6.570083055755264745, -4.705209693361169343 ) ) ;
#15715=ORIENTED_EDGE ( 'NONE', *, *, #12586, .F. ) ;
#15716=( BOUNDED_CURVE ( )  B_SPLINE_CURVE ( 3, ( #10249, #11702, #6360, #3373 ),
 .UNSPECIFIED., .F., .T. ) 
 B_SPLINE_CURVE_WITH_KNOTS ( ( 4, 4 ),
 ( 5.052230418047667371, 5.061454830783549852 ),
 .UNSPECIFIED. ) 
 CURVE ( )  GEOMETRIC_REPRESENTATION_ITEM ( )  RATIONAL_B_SPLINE_CURVE ( ( 1.000000000000000000, 0.9999929091967096895, 0.9999929091967096895, 1.000000000000000000 ) ) 
 REPRESENTATION_ITEM ( '' )  );
#15717=EDGE_LOOP ( 'NONE', ( #1293, #15353, #10874, #13898 ) ) ;
#15718=CARTESIAN_POINT ( 'NONE',  ( 26.21417678486618641, -2.370676134166772808, -5.783357778048658027 ) ) ;
#15722=ORIENTED_EDGE ( 'NONE', *, *, #5037, .T. ) ;
#15730=DIRECTION ( 'NONE',  ( -1.000000000000000000, 0.000000000000000000, 0.000000000000000000 ) ) ;
#15734=CYLINDRICAL_SURFACE ( 'NONE', #2335, 2.749999999999992006 ) ;
#15738=CARTESIAN_POINT ( 'NONE',  ( 31.98525019727866692, -6.363978266284800789, -7.033357778048666908 ) ) ;
#15741=DIRECTION ( 'NONE',  ( 0.9928203230275510771, 0.1196152422706614621, -0.000000000000000000 ) ) ;
#15742=DIRECTION ( 'NONE',  ( -1.000000000000000000, 0.000000000000000000, 0.000000000000000000 ) ) ;
#15745=CARTESIAN_POINT ( 'NONE',  ( 31.43732351782677625, -4.249272233123119413, -3.283357778048664688 ) ) ;
#15746=AXIS2_PLACEMENT_3D ( 'NONE', #474, #10155, #7101 ) ;
#15752=FACE_OUTER_BOUND ( 'NONE', #15333, .T. ) ;
#15755=CARTESIAN_POINT ( 'NONE',  ( 25.90934487712387480, 0.1208734971681818676, 4.216642221951339309 ) ) ;
#15758=EDGE_CURVE ( 'NONE', #15540, #11613, #1829, .T. ) ;
#15760=CARTESIAN_POINT ( 'NONE',  ( 27.48088551392658729, -7.244023872874614689, -5.783357778048657138 ) ) ;
#15762=CARTESIAN_POINT ( 'NONE',  ( -2.016448651773435938E-27, -20.49999999999999645, -12.00000000000000000 ) ) ;
#15768=ORIENTED_EDGE ( 'NONE', *, *, #2717, .T. ) ;
#15773=CARTESIAN_POINT ( 'NONE',  ( 27.17934203385504333, -30.00000000000000355, -13.93658524716016878 ) ) ;
#15779=DIRECTION ( 'NONE',  ( 0.1414213562373112243, -0.9899494936611663576, 0.000000000000000000 ) ) ;
#15780=CARTESIAN_POINT ( 'NONE',  ( 29.42285898892238549, -7.010054420087358018, -5.113484796970856117 ) ) ;
#15783=VERTEX_POINT ( 'NONE', #14758 ) ;
#15784=CARTESIAN_POINT ( 'NONE',  ( 27.10313151398701947, -6.652368374500619908, -6.861505862736166250 ) ) ;
#15793=CARTESIAN_POINT ( 'NONE',  ( 31.08270050955629671, -4.291997302367946077, -3.627061608673664672 ) ) ;
#15794=ORIENTED_EDGE ( 'NONE', *, *, #12326, .T. ) ;
#15799=ORIENTED_EDGE ( 'NONE', *, *, #218, .F. ) ;
#15800=CARTESIAN_POINT ( 'NONE',  ( 27.65458886993626564, -2.824105456627233224, -6.861505862736158257 ) ) ;
#15802=CARTESIAN_POINT ( 'NONE',  ( 26.24062359194589078, -6.129313013101781671, -3.627061608673667781 ) ) ;
#15822=CARTESIAN_POINT ( 'NONE',  ( 30.41656616297672500, -2.191532958677927745, -7.033357778048658027 ) ) ;
#15825=CARTESIAN_POINT ( 'NONE',  ( -8.632250723006722026, -18.84644399697197770, -16.84735068286508763 ) ) ;
#15829=CARTESIAN_POINT ( 'NONE',  ( 31.00882954110335632, -1.782818301463667598, -5.113484796970851676 ) ) ;
#15832=B_SPLINE_CURVE_WITH_KNOTS ( 'NONE', 1,
 ( #13599, #5153 ),
 .UNSPECIFIED., .F., .F.,
 ( 2, 2 ),
 ( 0.000000000000000000, 1.000000000000000000 ),
 .UNSPECIFIED. ) ;
#15835=ORIENTED_EDGE ( 'NONE', *, *, #17477, .F. ) ;
#15838=CARTESIAN_POINT ( 'NONE',  ( 50.00000000000000000, -19.03270077640483038, -5.537981825772250843 ) ) ;
#15840=CARTESIAN_POINT ( 'NONE',  ( 28.28511899221430070, -4.629050627332469858, -3.283357778048664688 ) ) ;
#15844=CARTESIAN_POINT ( 'NONE',  ( 32.93018312783485158, -2.815471066132994249, -3.627061608673662008 ) ) ;
#15850=ORIENTED_EDGE ( 'NONE', *, *, #17551, .T. ) ;
#15851=( BOUNDED_CURVE ( )  B_SPLINE_CURVE ( 2, ( #15760, #5946, #15390, #7239, #11279, #521, #11566, #2978, #7151 ),
 .UNSPECIFIED., .F., .T. ) 
 B_SPLINE_CURVE_WITH_KNOTS ( ( 3, 2, 2, 2, 3 ),
 ( 0.8269230769230769829, 0.8333333333333333703, 0.8461538461538461453, 0.8589743589743589203, 0.8653846153846154188 ),
 .UNSPECIFIED. ) 
 CURVE ( )  GEOMETRIC_REPRESENTATION_ITEM ( )  RATIONAL_B_SPLINE_CURVE ( ( 0.9330127018922192983, 0.9330127018922198534, 1.000000000000000000, 0.8660254037844387076, 1.000000000000000000, 0.8660254037844387076, 1.000000000000000000, 0.9330127018922187432, 0.9330127018922192983 ) ) 
 REPRESENTATION_ITEM ( '' )  );
#15853=CARTESIAN_POINT ( 'NONE',  ( 32.52441275490655670, -6.636378442139655220, -5.783357778048663356 ) ) ;
#15855=EDGE_CURVE ( 'NONE', #6589, #9029, #15949, .T. ) ;
#15856=VERTEX_POINT ( 'NONE', #13738 ) ;
#15859=ORIENTED_EDGE ( 'NONE', *, *, #10085, .F. ) ;
#15866=CARTESIAN_POINT ( 'NONE',  ( -26.79284261260708178, -21.20213040957736794, -14.03697675243215848 ) ) ;
#15868=CARTESIAN_POINT ( 'NONE',  ( 31.04700706809921940, -2.115577279836057922, -7.033357778048658027 ) ) ;
#15875=CARTESIAN_POINT ( 'NONE',  ( 33.76207435632690590, -3.969185667289998332, -3.627061608673664672 ) ) ;
#15878=AXIS2_PLACEMENT_3D ( 'NONE', #12871, #11485, #5781 ) ;
#15884=CARTESIAN_POINT ( 'NONE',  ( 30.75425665345519732, -2.450656702321377001, -4.705209693361161349 ) ) ;
#15886=ADVANCED_FACE ( 'NONE', ( #6929 ), #10201, .T. ) ;
#15889=DIRECTION ( 'NONE',  ( 4.179998415399335043E-17, -3.469446951953615175E-16, 1.000000000000000000 ) ) ;
#15893=CARTESIAN_POINT ( 'NONE',  ( 28.41655006632555569, -6.494127376913395366, -4.705209693361169343 ) ) ;
#15894=CARTESIAN_POINT ( 'NONE',  ( 26.25801688195511474, -3.619335333876111171, -7.939653947423660263 ) ) ;
#15895=CARTESIAN_POINT ( 'NONE',  ( 35.74085044863416982, 7.999999999999934275, -11.27079897466147429 ) ) ;
#15897=CARTESIAN_POINT ( 'NONE',  ( 16.03720890403358013, 12.19600435288735341, -16.13737481314213440 ) ) ;
#15903=EDGE_LOOP ( 'NONE', ( #5801, #12841, #6772, #7954 ) ) ;
#15908=CYLINDRICAL_SURFACE ( 'NONE', #10199, 2.000000000000001776 ) ;
#15911=CARTESIAN_POINT ( 'NONE',  ( 32.06767520579373354, -2.292415704734142690, -6.861505862736158257 ) ) ;
#15913=ORIENTED_EDGE ( 'NONE', *, *, #14410, .T. ) ;
#15915=CARTESIAN_POINT ( 'NONE',  ( 28.36392410707646761, -4.619556167269785796, -3.283357778048664688 ) ) ;
#15920=CARTESIAN_POINT ( 'NONE',  ( 19.43845002722867221, 2.988003976273734263, -6.000000000000000000 ) ) ;
#15924=( BOUNDED_CURVE ( )  B_SPLINE_CURVE ( 3, ( #2092, #13139, #14688, #15773 ),
 .UNSPECIFIED., .F., .T. ) 
 B_SPLINE_CURVE_WITH_KNOTS ( ( 4, 4 ),
 ( 4.846194975958193929, 4.967031014587541371 ),
 .UNSPECIFIED. ) 
 CURVE ( )  GEOMETRIC_REPRESENTATION_ITEM ( )  RATIONAL_B_SPLINE_CURVE ( ( 1.000000000000000000, 0.9987835910734579326, 0.9987835910734579326, 1.000000000000000000 ) ) 
 REPRESENTATION_ITEM ( '' )  );
#15929=ORIENTED_EDGE ( 'NONE', *, *, #13003, .T. ) ;
#15946=CARTESIAN_POINT ( 'NONE',  ( 26.02974819644417792, -2.720057890826728109, -4.533357778048659803 ) ) ;
#15949=( BOUNDED_CURVE ( )  B_SPLINE_CURVE ( 2, ( #2771, #13819, #8378, #49, #3949, #5560, #9379, #1406, #1140 ),
 .UNSPECIFIED., .F., .T. ) 
 B_SPLINE_CURVE_WITH_KNOTS ( ( 3, 2, 2, 2, 3 ),
 ( 0.05769230769230771633, 0.06410256410256409687, 0.07692307692307692735, 0.08974358974358974395, 0.09615384615384617306 ),
 .UNSPECIFIED. ) 
 CURVE ( )  GEOMETRIC_REPRESENTATION_ITEM ( )  RATIONAL_B_SPLINE_CURVE ( ( 0.9330127018922194093, 0.9330127018922196314, 1.000000000000000000, 0.8660254037844387076, 1.000000000000000000, 0.8660254037844387076, 1.000000000000000000, 0.9330127018922191873, 0.9330127018922194093 ) ) 
 REPRESENTATION_ITEM ( '' )  );
#15950=VECTOR ( 'NONE', #9009, 1000.000000000000000 ) ;
#15954=EDGE_LOOP ( 'NONE', ( #1114, #8862 ) ) ;
#15955=DIRECTION ( 'NONE',  ( 0.9928203230275512992, 0.1196152422706614898, -0.000000000000000000 ) ) ;
#15962=CARTESIAN_POINT ( 'NONE',  ( -20.27016866188220945, -21.85533094420792466, -15.46350303853101593 ) ) ;
#15964=CYLINDRICAL_SURFACE ( 'NONE', #11897, 6.249999999999998224 ) ;
#15968=CIRCLE ( 'NONE', #7559, 13.00000000000000178 ) ;
#15974=CARTESIAN_POINT ( 'NONE',  ( 26.45077056032005913, -6.103994453487816330, -7.939653947423664704 ) ) ;
#15978=PLANE ( 'NONE',  #6607 ) ;
#15982=CARTESIAN_POINT ( 'NONE',  ( 29.23078034989804763, -4.515117109069654688, -8.283357778048662468 ) ) ;
#15984=VECTOR ( 'NONE', #10526, 1000.000000000000227 ) ;
#15985=CARTESIAN_POINT ( 'NONE',  ( 32.65880277236253448, -4.102108105263264193, -7.939653947423662039 ) ) ;
#15986=ORIENTED_EDGE ( 'NONE', *, *, #15055, .F. ) ;
#15988=CARTESIAN_POINT ( 'NONE',  ( 26.01345249736710841, -4.876873030332669501, -8.181274557237335543 ) ) ;
#15989=FACE_OUTER_BOUND ( 'NONE', #1908, .T. ) ;
#15991=CARTESIAN_POINT ( 'NONE',  ( -2.016448651773435938E-27, -20.49999999999999645, -6.000000000000000000 ) ) ;
#15992=EDGE_CURVE ( 'NONE', #5342, #15678, #11350, .T. ) ;
#15993=CARTESIAN_POINT ( 'NONE',  ( 29.81239362717914787, -2.264323817775507397, -4.533357778048659803 ) ) ;
#15994=CARTESIAN_POINT ( 'NONE',  ( 26.84461768998868436, -2.294720455324902542, -5.783357778048658027 ) ) ;
#15995=VECTOR ( 'NONE', #11544, 1000.000000000000227 ) ;
#15996=CARTESIAN_POINT ( 'NONE',  ( -32.93004296264518160, -25.68697430340739629, -12.29384923381406658 ) ) ;
#15998=CARTESIAN_POINT ( 'NONE',  ( 4.081988505578530102, 17.67880197223097127, -16.99999999999999645 ) ) ;
#16003=CARTESIAN_POINT ( 'NONE',  ( -20.00000000000000000, 7.999999999999996447, 0.000000000000000000 ) ) ;
#16006=ORIENTED_EDGE ( 'NONE', *, *, #10483, .T. ) ;
#16010=CARTESIAN_POINT ( 'NONE',  ( 32.30426898124760982, -6.025734024055190652, -6.861505862736167138 ) ) ;
#16011=EDGE_CURVE ( 'NONE', #6049, #10596, #8116, .T. ) ;
#16015=CARTESIAN_POINT ( 'NONE',  ( 27.73348320195396965, -4.695511846111656062, -3.283357778048664688 ) ) ;
#16016=DIRECTION ( 'NONE',  ( 0.000000000000000000, -1.000000000000000000, -3.469446951953614189E-16 ) ) ;
#16018=DIRECTION ( 'NONE',  ( 0.000000000000000000, 0.000000000000000000, 1.000000000000000000 ) ) ;
#16024=CARTESIAN_POINT ( 'NONE',  ( 28.29630561643014275, -19.54286113573893502, -13.63865706309495884 ) ) ;
#16025=AXIS2_PLACEMENT_3D ( 'NONE', #11381, #11184, #15483 ) ;
#16027=VECTOR ( 'NONE', #7858, 1000.000000000000000 ) ;
#16037=VERTEX_POINT ( 'NONE', #13650 ) ;
#16040=CARTESIAN_POINT ( 'NONE',  ( 33.44685390376565692, -4.007163506710925027, -7.939653947423662039 ) ) ;
#16041=VERTEX_POINT ( 'NONE', #1238 ) ;
#16043=CARTESIAN_POINT ( 'NONE',  ( 28.74176732417158320, -7.092112515190875044, -5.783357778048657138 ) ) ;
#16047=CARTESIAN_POINT ( 'NONE',  ( 32.92339180097568629, -5.524043937428110063, -3.283357778048667797 ) ) ;
#16049=DIRECTION ( 'NONE',  ( 0.000000000000000000, 0.000000000000000000, 1.000000000000000000 ) ) ;
#16053=EDGE_LOOP ( 'NONE', ( #12457, #16951, #2206, #7453 ) ) ;
#16056=EDGE_LOOP ( 'NONE', ( #12360, #4937, #9053, #9976 ) ) ;
#16062=CARTESIAN_POINT ( 'NONE',  ( 35.46635924378174565, -16.45598204045931823, -11.37070560279563480 ) ) ;
#16069=CARTESIAN_POINT ( 'NONE',  ( 26.97161122272022382, -2.906390775372597712, -4.705209693361161349 ) ) ;
#16072=EDGE_CURVE ( 'NONE', #16640, #9754, #9003, .T. ) ;
#16073=LINE ( 'NONE', #913, #16463 ) ;
#16075=ORIENTED_EDGE ( 'NONE', *, *, #3369, .T. ) ;
#16077=CARTESIAN_POINT ( 'NONE',  ( 31.28415083292585663, -5.521667582366822202, -3.627061608673667781 ) ) ;
#16078=ORIENTED_EDGE ( 'NONE', *, *, #182, .F. ) ;
#16080=CARTESIAN_POINT ( 'NONE',  ( 25.90419076669538256, -3.969988049114259177, -7.913474645583921330 ) ) ;
#16081=LINE ( 'NONE', #7455, #17117 ) ;
#16084=CARTESIAN_POINT ( 'NONE',  ( 31.84257795004535652, -2.746633492292519296, -3.283357778048662023 ) ) ;
#16086=CARTESIAN_POINT ( 'NONE',  ( 25.71072941247523502, -3.058302133056337357, -4.705209693361161349 ) ) ;
#16087=DIRECTION ( 'NONE',  ( 0.000000000000000000, 0.000000000000000000, 1.000000000000000000 ) ) ;
#16089=DIRECTION ( 'NONE',  ( 0.000000000000000000, 0.000000000000000000, 1.000000000000000000 ) ) ;
#16102=CARTESIAN_POINT ( 'NONE',  ( 15.92260893619738837, -28.39189527176317540, -12.00000000000000000 ) ) ;
#16103=CARTESIAN_POINT ( 'NONE',  ( 27.17934203385504333, -30.00000000000000355, -12.00000000000000000 ) ) ;
#16105=CARTESIAN_POINT ( 'NONE',  ( 28.79925754835455010, -6.020920669644549861, -8.283357778048662468 ) ) ;
#16108=LINE ( 'NONE', #6488, #9746 ) ;
#16117=VERTEX_POINT ( 'NONE', #6010 ) ;
#16124=EDGE_CURVE ( 'NONE', #16117, #4517, #11251, .T. ) ;
#16126=CARTESIAN_POINT ( 'NONE',  ( 32.32618902979206865, -6.650063623909865385, -5.783357778048669573 ) ) ;
#16128=CARTESIAN_POINT ( 'NONE',  ( 28.43075721014566781, -2.093425104433228157, -6.453230759126469707 ) ) ;
#16129=FACE_OUTER_BOUND ( 'NONE', #13883, .T. ) ;
#16131=LINE ( 'NONE', #9961, #2678 ) ;
#16133=CARTESIAN_POINT ( 'NONE',  ( 25.71748644841968456, -2.420320648352051851, -5.783357778048663356 ) ) ;
#16135=EDGE_CURVE ( 'NONE', #9754, #1502, #12698, .T. ) ;
#16138=ORIENTED_EDGE ( 'NONE', *, *, #1767, .F. ) ;
#16139=ORIENTED_EDGE ( 'NONE', *, *, #2895, .F. ) ;
#16143=CARTESIAN_POINT ( 'NONE',  ( -2.016448651773435938E-27, -20.49999999999999645, -13.00000000000000355 ) ) ;
#16145=CARTESIAN_POINT ( 'NONE',  ( 27.29814976067589072, -3.294147343736874234, -8.283357778048660691 ) ) ;
#16149=DIRECTION ( 'NONE',  ( 0.9928203230275510771, 0.1196152422706614621, -0.000000000000000000 ) ) ;
#16150=CARTESIAN_POINT ( 'NONE',  ( 26.60838078660069428, -6.085005533777348319, -7.939653947423664704 ) ) ;
#16153=CARTESIAN_POINT ( 'NONE',  ( 32.72003615946069743, -2.840789625746940938, -7.939653947423660263 ) ) ;
#16156=AXIS2_PLACEMENT_3D ( 'NONE', #8530, #12520, #10 ) ;
#16159=AXIS2_PLACEMENT_3D ( 'NONE', #13723, #2756, #2926 ) ;
#16162=CARTESIAN_POINT ( 'NONE',  ( 31.88814493096864311, -1.687075024589942407, -5.783357778048658915 ) ) ;
#16165=CARTESIAN_POINT ( 'NONE',  ( 26.10492286888475633, -5.636087676172646610, -8.120510362352304057 ) ) ;
#16169=CARTESIAN_POINT ( 'NONE',  ( 31.21213704492286212, -2.822589171134389563, -3.283357778048662023 ) ) ;
#16172=CARTESIAN_POINT ( 'NONE',  ( 32.79901970863393501, -6.593096864778464017, -5.783357778048668685 ) ) ;
#16180=AXIS2_PLACEMENT_3D ( 'NONE', #16774, #10131, #3261 ) ;
#16181=ORIENTED_EDGE ( 'NONE', *, *, #11344, .T. ) ;
#16190=CARTESIAN_POINT ( 'NONE',  ( 33.30663696749426350, -1.516174747195734085, -5.783357778048658915 ) ) ;
#16193=CARTESIAN_POINT ( 'NONE',  ( 28.83304567166618781, -6.743756660494150346, -7.033357778048666908 ) ) ;
#16200=CARTESIAN_POINT ( 'NONE',  ( 26.12396475346091052, -21.64644127732803014, -14.20549555447399470 ) ) ;
#16203=VERTEX_POINT ( 'NONE', #10358 ) ;
#16207=CARTESIAN_POINT ( 'NONE',  ( 26.31556265977298992, -7.384422263489805793, -5.783357778048663356 ) ) ;
#16210=LINE ( 'NONE', #3413, #16810 ) ;
#16212=CARTESIAN_POINT ( 'NONE',  ( 29.17398450417959310, -7.029842018119214941, -5.783357778048669573 ) ) ;
#16215=DIRECTION ( 'NONE',  ( -0.1196152422706614343, 0.9928203230275510771, 0.000000000000000000 ) ) ;
#16229=CARTESIAN_POINT ( 'NONE',  ( 50.00000000000000000, -16.03270077640482683, -5.537981825772250843 ) ) ;
#16233=DIRECTION ( 'NONE',  ( 1.000000000000000000, 0.000000000000000000, 0.000000000000000000 ) ) ;
#16237=EDGE_CURVE ( 'NONE', #2633, #2890, #10452, .T. ) ;
#16238=CARTESIAN_POINT ( 'NONE',  ( 27.77288575766320378, -4.690764616287755651, -7.939653947423662039 ) ) ;
#16242=CARTESIAN_POINT ( 'NONE',  ( 30.28142597461332741, -2.507623461452779701, -4.705209693361160461 ) ) ;
#16243=AXIS2_PLACEMENT_3D ( 'NONE', #4917, #943, #11804 ) ;
#16247=CARTESIAN_POINT ( 'NONE',  ( -45.00000000000000711, -16.03270077640482683, -5.537981825772250843 ) ) ;
#16250=CARTESIAN_POINT ( 'NONE',  ( 28.23249303296521617, -2.754479417688857179, -4.705209693361161349 ) ) ;
#16258=CARTESIAN_POINT ( 'NONE',  ( 32.82573654529290508, -1.174368712523534475, -5.783357778048658027 ) ) ;
#16262=CARTESIAN_POINT ( 'NONE',  ( 32.67202617590239555, -5.981426544730773287, -4.705209693361168455 ) ) ;
#16273=CARTESIAN_POINT ( 'NONE',  ( 33.60446413004628141, -3.988174587000466342, -3.627061608673664672 ) ) ;
#16275=( LENGTH_UNIT ( ) NAMED_UNIT ( * ) SI_UNIT ( .MILLI., .METRE. ) );
#16278=FACE_OUTER_BOUND ( 'NONE', #10688, .T. ) ;
#16280=EDGE_CURVE ( 'NONE', #11429, #1653, #2145, .T. ) ;
#16281=CARTESIAN_POINT ( 'NONE',  ( 26.69778786461289855, -6.274106265784127778, -3.283357778048667797 ) ) ;
#16286=VECTOR ( 'NONE', #7990, 1000.000000000000000 ) ;
#16299=CARTESIAN_POINT ( 'NONE',  ( 31.65190802758064592, -5.477360103042387074, -7.939653947423664704 ) ) ;
#16300=( BOUNDED_SURFACE ( )  B_SPLINE_SURFACE ( 1, 2, ( 
 ( #2344, #11838, #17415, #14594, #11663, #10561, #16040, #974, #10476, #3334, #615, #4769, #10294, #15844, #3416, #6501, #3610, #877, #11747, #9131, #8949, #7862, #14490, #8864, #2169, #7769, #14671, #17316, #2251, #6410, #11929, #2074, #17517, #16126, #3686, #9210, #14759, #13393, #12017, #10897, #13482, #13820, #16466, #16299, #1407, #2426, #15187, #13739, #5207, #8290, #12102, #16388, #1320, #5470, #3869, #3950, #10991, #6930, #13563, #9301, #10727, #8211, #17937, #9638, #4035, #9552, #3778, #16549, #8119, #13651, #1058, #5294, #50, #14842, #6579, #9381, #5381, #12462, #2591, #5561, #14924, #17686, #12291, #2502, #1239, #1142, #8026, #6761, #6668, #6843, #12196, #17777, #2682, #16212, #10815, #2772, #7950, #9465, #15005, #17860, #15097, #12371, #4133, #3126, #4304, #8659, #15893, #7129, #3465, #17015, #14014, #13169, #4568, #5739, #9719, #9816, #7039, #2851, #14542, #745, #14187, #13911, #9910, #8478, #8997, #2124, #12554, #15367, #1504, #325, #7646, #138, #4483, #11080, #1597, #7308, #5650, #3043, #16644, #1780, #9998, #15542, #5831, #12829, #8379, #4219, #12640, #11252, #420, #11161, #4395, #229, #15270, #16732, #2948 ),
 ( #5924, #10337, #11356, #16926, #16831, #11448, #8564, #14097, #15458, #1683, #7217, #12729, #14631, #13250, #13440, #16258, #13613, #2470, #9345, #1020, #14966, #7907, #17562, #3832, #11979, #835, #3563, #14716, #2299, #9255, #3732, #10524, #3652, #14884, #5081, #6362, #9090, #16084, #11886, #10601, #2550, #5166, #17645, #10774, #7992, #17465, #7726, #17371, #8077, #16169, #9173, #12058, #6270, #2212, #4905, #16355, #7817, #13347, #4997, #14800, #927, #6461, #11792, #13526, #10431, #5254, #2391, #6543, #10682, #1100, #6624, #12152, #3915, #17734, #15993, #9426, #3997, #8173, #13704, #9513, #16785, #1456, #16692, #4086, #6987, #1287, #186, #2644, #1196, #6891, #5608, #9683, #15152, #16606, #10950, #12516, #5340, #9595, #3005, #10862, #13789, #4184, #15058, #6810, #13872, #16431, #4353, #101, #12336, #9864, #17900, #5695, #4268, #5431, #11210, #16513, #1367, #9770, #8430, #2734, #12420, #13968, #15419, #8256, #12254, #7, #11125, #2901, #12606, #15323, #1554, #6713, #7088, #11042, #15234, #5523, #2812, #8525, #17822, #8337, #3090, #3272, #6064, #3446, #10234, #17161, #8805, #4794, #15691, #7362, #11591, #1831, #8611, #11307, #4528 ) ),
 .UNSPECIFIED., .F., .F., .T. ) 
 B_SPLINE_SURFACE_WITH_KNOTS ( ( 2, 2 ),
 ( 3, 2, 2, 2, 2, 2, 2, 2, 2, 2, 2, 2, 2, 2, 2, 2, 2, 2, 2, 2, 2, 2, 2, 2, 2, 2, 2, 2, 2, 2, 2, 2, 2, 2, 2, 2, 2, 2, 2, 2, 2, 2, 2, 2, 2, 2, 2, 2, 2, 2, 2, 2, 2, 2, 2, 2, 2, 2, 2, 2, 2, 2, 2, 2, 2, 2, 2, 2, 2, 2, 2, 2, 2, 2, 2, 2, 2, 3 ),
 ( 0.000000000000000000, 1.000000000000000000 ),
 ( 0.000000000000000000, 0.01282051282051282007, 0.02564102564102564014, 0.03846153846153846367, 0.05128205128205128027, 0.06410256410256409687, 0.07692307692307692735, 0.08974358974358974395, 0.1025641025641025605, 0.1153846153846153910, 0.1282051282051281937, 0.1410256410256410242, 0.1538461538461538547, 0.1666666666666666574, 0.1794871794871794879, 0.1923076923076923184, 0.2051282051282051211, 0.2179487179487179516, 0.2307692307692307820, 0.2435897435897435848, 0.2564102564102563875, 0.2692307692307692180, 0.2820512820512820484, 0.2948717948717948789, 0.3076923076923077094, 0.3205128205128205399, 0.3333333333333333148, 0.3461538461538461453, 0.3589743589743589758, 0.3717948717948718063, 0.3846153846153846367, 0.3974358974358974117, 0.4102564102564102422, 0.4230769230769230727, 0.4358974358974359031, 0.4487179487179487336, 0.4615384615384615641, 0.4743589743589743390, 0.4871794871794871695, 0.5000000000000000000, 0.5128205128205127750, 0.5256410256410256610, 0.5384615384615384359, 0.5512820512820513219, 0.5641025641025640969, 0.5769230769230768718, 0.5897435897435897578, 0.6025641025641025328, 0.6153846153846154188, 0.6282051282051281937, 0.6410256410256410797, 0.6538461538461538547, 0.6666666666666666297, 0.6794871794871795156, 0.6923076923076922906, 0.7051282051282051766, 0.7179487179487179516, 0.7307692307692307265, 0.7435897435897436125, 0.7564102564102563875, 0.7692307692307692735, 0.7820512820512820484, 0.7948717948717948234, 0.8076923076923077094, 0.8205128205128204844, 0.8333333333333333703, 0.8461538461538461453, 0.8589743589743589203, 0.8717948717948718063, 0.8846153846153845812, 0.8974358974358974672, 0.9102564102564102422, 0.9230769230769231282, 0.9358974358974359031, 0.9487179487179486781, 0.9615384615384615641, 0.9690837477411259338, 0.9787745852185372186 ),
 .UNSPECIFIED. ) 
 GEOMETRIC_REPRESENTATION_ITEM ( )  RATIONAL_B_SPLINE_SURFACE ( (
 ( 1.000000000000000000, 0.8660254037844387076, 1.000000000000000000, 0.8660254037844387076, 1.000000000000000000, 0.8660254037844387076, 1.000000000000000000, 0.8660254037844387076, 1.000000000000000000, 0.8660254037844387076, 1.000000000000000000, 0.8660254037844387076, 1.000000000000000000, 0.8660254037844387076, 1.000000000000000000, 0.8660254037844387076, 1.000000000000000000, 0.8660254037844387076, 1.000000000000000000, 0.8660254037844387076, 1.000000000000000000, 0.8660254037844387076, 1.000000000000000000, 0.8660254037844387076, 1.000000000000000000, 0.8660254037844387076, 1.000000000000000000, 0.8660254037844387076, 1.000000000000000000, 0.8660254037844387076, 1.000000000000000000, 0.8660254037844387076, 1.000000000000000000, 0.8660254037844387076, 1.000000000000000000, 0.8660254037844387076, 1.000000000000000000, 0.8660254037844387076, 1.000000000000000000, 0.8660254037844387076, 1.000000000000000000, 0.8660254037844387076, 1.000000000000000000, 0.8660254037844387076, 1.000000000000000000, 0.8660254037844387076, 1.000000000000000000, 0.8660254037844387076, 1.000000000000000000, 0.8660254037844387076, 1.000000000000000000, 0.8660254037844387076, 1.000000000000000000, 0.8660254037844387076, 1.000000000000000000, 0.8660254037844387076, 1.000000000000000000, 0.8660254037844387076, 1.000000000000000000, 0.8660254037844387076, 1.000000000000000000, 0.8660254037844387076, 1.000000000000000000, 0.8660254037844387076, 1.000000000000000000, 0.8660254037844387076, 1.000000000000000000, 0.8660254037844387076, 1.000000000000000000, 0.8660254037844387076, 1.000000000000000000, 0.8660254037844387076, 1.000000000000000000, 0.8660254037844387076, 1.000000000000000000, 0.8660254037844387076, 1.000000000000000000, 0.8660254037844387076, 1.000000000000000000, 0.8660254037844387076, 1.000000000000000000, 0.8660254037844387076, 1.000000000000000000, 0.8660254037844387076, 1.000000000000000000, 0.8660254037844387076, 1.000000000000000000, 0.8660254037844387076, 1.000000000000000000, 0.8660254037844387076, 1.000000000000000000, 0.8660254037844387076, 1.000000000000000000, 0.8660254037844387076, 1.000000000000000000, 0.8660254037844387076, 1.000000000000000000, 0.8660254037844387076, 1.000000000000000000, 0.8660254037844387076, 1.000000000000000000, 0.8660254037844387076, 1.000000000000000000, 0.8660254037844387076, 1.000000000000000000, 0.8660254037844387076, 1.000000000000000000, 0.8660254037844387076, 1.000000000000000000, 0.8660254037844387076, 1.000000000000000000, 0.8660254037844387076, 1.000000000000000000, 0.8660254037844387076, 1.000000000000000000, 0.8660254037844387076, 1.000000000000000000, 0.8660254037844387076, 1.000000000000000000, 0.8660254037844387076, 1.000000000000000000, 0.8660254037844387076, 1.000000000000000000, 0.8660254037844387076, 1.000000000000000000, 0.8660254037844387076, 1.000000000000000000, 0.8660254037844387076, 1.000000000000000000, 0.8660254037844387076, 1.000000000000000000, 0.8660254037844387076, 1.000000000000000000, 0.8660254037844387076, 1.000000000000000000, 0.8660254037844387076, 1.000000000000000000, 0.8660254037844387076, 1.000000000000000000, 0.8660254037844387076, 1.000000000000000000, 0.8660254037844387076, 1.000000000000000000, 0.8660254037844387076, 1.000000000000000000, 0.8660254037844387076, 1.000000000000000000, 0.8660254037844387076, 1.000000000000000000, 0.8660254037844387076, 1.000000000000000000, 0.9211516195580409239, 0.9351128802560608744, 0.9351128802560608744, 0.9351128802560608744),
 ( 1.000000000000000000, 0.8660254037844387076, 1.000000000000000000, 0.8660254037844387076, 1.000000000000000000, 0.8660254037844387076, 1.000000000000000000, 0.8660254037844387076, 1.000000000000000000, 0.8660254037844387076, 1.000000000000000000, 0.8660254037844387076, 1.000000000000000000, 0.8660254037844387076, 1.000000000000000000, 0.8660254037844387076, 1.000000000000000000, 0.8660254037844387076, 1.000000000000000000, 0.8660254037844387076, 1.000000000000000000, 0.8660254037844387076, 1.000000000000000000, 0.8660254037844387076, 1.000000000000000000, 0.8660254037844387076, 1.000000000000000000, 0.8660254037844387076, 1.000000000000000000, 0.8660254037844387076, 1.000000000000000000, 0.8660254037844387076, 1.000000000000000000, 0.8660254037844387076, 1.000000000000000000, 0.8660254037844387076, 1.000000000000000000, 0.8660254037844387076, 1.000000000000000000, 0.8660254037844387076, 1.000000000000000000, 0.8660254037844387076, 1.000000000000000000, 0.8660254037844387076, 1.000000000000000000, 0.8660254037844387076, 1.000000000000000000, 0.8660254037844387076, 1.000000000000000000, 0.8660254037844387076, 1.000000000000000000, 0.8660254037844387076, 1.000000000000000000, 0.8660254037844387076, 1.000000000000000000, 0.8660254037844387076, 1.000000000000000000, 0.8660254037844387076, 1.000000000000000000, 0.8660254037844387076, 1.000000000000000000, 0.8660254037844387076, 1.000000000000000000, 0.8660254037844387076, 1.000000000000000000, 0.8660254037844387076, 1.000000000000000000, 0.8660254037844387076, 1.000000000000000000, 0.8660254037844387076, 1.000000000000000000, 0.8660254037844387076, 1.000000000000000000, 0.8660254037844387076, 1.000000000000000000, 0.8660254037844387076, 1.000000000000000000, 0.8660254037844387076, 1.000000000000000000, 0.8660254037844387076, 1.000000000000000000, 0.8660254037844387076, 1.000000000000000000, 0.8660254037844387076, 1.000000000000000000, 0.8660254037844387076, 1.000000000000000000, 0.8660254037844387076, 1.000000000000000000, 0.8660254037844387076, 1.000000000000000000, 0.8660254037844387076, 1.000000000000000000, 0.8660254037844387076, 1.000000000000000000, 0.8660254037844387076, 1.000000000000000000, 0.8660254037844387076, 1.000000000000000000, 0.8660254037844387076, 1.000000000000000000, 0.8660254037844387076, 1.000000000000000000, 0.8660254037844387076, 1.000000000000000000, 0.8660254037844387076, 1.000000000000000000, 0.8660254037844387076, 1.000000000000000000, 0.8660254037844387076, 1.000000000000000000, 0.8660254037844387076, 1.000000000000000000, 0.8660254037844387076, 1.000000000000000000, 0.8660254037844387076, 1.000000000000000000, 0.8660254037844387076, 1.000000000000000000, 0.8660254037844387076, 1.000000000000000000, 0.8660254037844387076, 1.000000000000000000, 0.8660254037844387076, 1.000000000000000000, 0.8660254037844387076, 1.000000000000000000, 0.8660254037844387076, 1.000000000000000000, 0.8660254037844387076, 1.000000000000000000, 0.8660254037844387076, 1.000000000000000000, 0.8660254037844387076, 1.000000000000000000, 0.8660254037844387076, 1.000000000000000000, 0.8660254037844387076, 1.000000000000000000, 0.8660254037844387076, 1.000000000000000000, 0.8660254037844387076, 1.000000000000000000, 0.8660254037844387076, 1.000000000000000000, 0.8660254037844387076, 1.000000000000000000, 0.8660254037844387076, 1.000000000000000000, 0.8660254037844387076, 1.000000000000000000, 0.9211516195580409239, 0.9351128802560608744, 0.9351128802560608744, 0.9351128802560608744) ) ) 
 REPRESENTATION_ITEM ( '' )  SURFACE ( )  );
#16309=CARTESIAN_POINT ( 'NONE',  ( 31.11087420047036289, -5.742416513891037688, -3.283357778048667797 ) ) ;
#16314=VERTEX_POINT ( 'NONE', #13463 ) ;
#16316=VERTEX_POINT ( 'NONE', #5018 ) ;
#16326=CARTESIAN_POINT ( 'NONE',  ( 25.93714794488954212, -2.393855775999666591, -5.783357778048658027 ) ) ;
#16328=CARTESIAN_POINT ( 'NONE',  ( 28.52524344760924180, -2.419399995203538101, -7.033357778048658027 ) ) ;
#16337=CARTESIAN_POINT ( 'NONE',  ( 30.30787278169304244, -6.266260340387784566, -4.705209693361169343 ) ) ;
#16340=DIRECTION ( 'NONE',  ( -0.1196152422706611984, 0.9928203230275510771, 0.000000000000000000 ) ) ;
#16341=CIRCLE ( 'NONE', #14310, 5.000000000000000000 ) ;
#16342=DIRECTION ( 'NONE',  ( 0.000000000000000000, 0.000000000000000000, 1.000000000000000000 ) ) ;
#16348=CARTESIAN_POINT ( 'NONE',  ( 28.76238721243587548, -5.825490297734302381, -3.627061608673667781 ) ) ;
#16351=LINE ( 'NONE', #7989, #12171 ) ;
#16352=LINE ( 'NONE', #3995, #51 ) ;
#16353=AXIS2_PLACEMENT_3D ( 'NONE', #12932, #14590, #13207 ) ;
#16355=CARTESIAN_POINT ( 'NONE',  ( 31.24221605398236790, -5.726592414339752857, -8.283357778048662468 ) ) ;
#16357=LINE ( 'NONE', #3835, #15984 ) ;
#16359=FACE_OUTER_BOUND ( 'NONE', #13021, .T. ) ;
#16362=EDGE_CURVE ( 'NONE', #14027, #2784, #16424, .T. ) ;
#16364=CARTESIAN_POINT ( 'NONE',  ( -23.00000000000000000, -16.21813761408365195, -13.00000000000000355 ) ) ;
#16366=CARTESIAN_POINT ( 'NONE',  ( -2.016448651773435938E-27, -20.49999999999999645, -6.000000000000000000 ) ) ;
#16367=ORIENTED_EDGE ( 'NONE', *, *, #15285, .T. ) ;
#16368=SURFACE_STYLE_USAGE ( .BOTH. , #5273 ) ;
#16369=CARTESIAN_POINT ( 'NONE',  ( 31.02146712245815507, -5.553315781884258229, -7.939653947423662927 ) ) ;
#16371=CARTESIAN_POINT ( 'NONE',  ( 26.15738093914773543, -4.885401043216321959, -8.283357778048662468 ) ) ;
#16377=ORIENTED_EDGE ( 'NONE', *, *, #14376, .T. ) ;
#16384=DIRECTION ( 'NONE',  ( 0.9928203230275510771, 0.1196152422706614205, 0.000000000000000000 ) ) ;
#16387=CARTESIAN_POINT ( 'NONE',  ( 33.95908713831673964, -3.945449517755637014, -5.783357778048663356 ) ) ;
#16388=CARTESIAN_POINT ( 'NONE',  ( 30.78487334700428590, -1.819997462563214263, -5.783357778048658027 ) ) ;
#16392=DIRECTION ( 'NONE',  ( 0.000000000000000000, 0.000000000000000000, 1.000000000000000000 ) ) ;
#16397=EDGE_CURVE ( 'NONE', #5110, #16590, #2667, .T. ) ;
#16398=ORIENTED_EDGE ( 'NONE', *, *, #12361, .F. ) ;
#16402=ORIENTED_EDGE ( 'NONE', *, *, #6758, .F. ) ;
#16403=( BOUNDED_CURVE ( )  B_SPLINE_CURVE ( 3, ( #8500, #10114, #9841, #1531 ),
 .UNSPECIFIED., .F., .T. ) 
 B_SPLINE_CURVE_WITH_KNOTS ( ( 4, 4 ),
 ( 4.889642689481717319, 5.052230418047667371 ),
 .UNSPECIFIED. ) 
 CURVE ( )  GEOMETRIC_REPRESENTATION_ITEM ( )  RATIONAL_B_SPLINE_CURVE ( ( 1.000000000000000000, 0.9977983154653931042, 0.9977983154653931042, 1.000000000000000000 ) ) 
 REPRESENTATION_ITEM ( '' )  );
#16407=PLANE ( 'NONE',  #951 ) ;
#16412=CARTESIAN_POINT ( 'NONE',  ( 16.75000000000000000, -15.80031936969768935, -16.03574476417183803 ) ) ;
#16413=CARTESIAN_POINT ( 'NONE',  ( 7.499998387031003411, -20.49508120620799900, -17.00000000000000000 ) ) ;
#16416=CARTESIAN_POINT ( 'NONE',  ( 31.54230778485832332, -2.355712103769039611, -4.705209693361160461 ) ) ;
#16418=DIRECTION ( 'NONE',  ( 0.1196152422706605323, -0.9928203230275512992, 0.000000000000000000 ) ) ;
#16419=CARTESIAN_POINT ( 'NONE',  ( 31.63243098167119172, -2.771952051906466430, -8.283357778048660691 ) ) ;
#16420=ORIENTED_EDGE ( 'NONE', *, *, #1761, .T. ) ;
#16423=CARTESIAN_POINT ( 'NONE',  ( 29.19137779418881351, -4.519864338893556877, -3.627061608673664672 ) ) ;
#16424=( BOUNDED_CURVE ( )  B_SPLINE_CURVE ( 3, ( #15249, #17840, #10878, #6645 ),
 .UNSPECIFIED., .F., .T. ) 
 B_SPLINE_CURVE_WITH_KNOTS ( ( 4, 4 ),
 ( 1.514099494053832595, 1.567750514535811712 ),
 .UNSPECIFIED. ) 
 CURVE ( )  GEOMETRIC_REPRESENTATION_ITEM ( )  RATIONAL_B_SPLINE_CURVE ( ( 1.000000000000000000, 0.9997601450507493936, 0.9997601450507493936, 1.000000000000000000 ) ) 
 REPRESENTATION_ITEM ( '' )  );
#16429=CARTESIAN_POINT ( 'NONE',  ( 33.95908713831674675, -3.945449517755636126, -5.783357778048663356 ) ) ;
#16431=CARTESIAN_POINT ( 'NONE',  ( 28.78802868011566929, -7.476087111406434893, -5.783357778048669573 ) ) ;
#16432=VERTEX_POINT ( 'NONE', #12440 ) ;
#16435=CARTESIAN_POINT ( 'NONE',  ( 28.19013153391124860, -7.158573733970061248, -5.783357778048657138 ) ) ;
#16437=CARTESIAN_POINT ( 'NONE',  ( 45.00000000000000711, -16.03270077640482683, -0.5379818257722508434 ) ) ;
#16441=LINE ( 'NONE', #2822, #13449 ) ;
#16442=CARTESIAN_POINT ( 'NONE',  ( 26.01652455409633902, -4.902371455920928156, -5.783357778048663356 ) ) ;
#16444=( NAMED_UNIT ( * ) PLANE_ANGLE_UNIT ( ) SI_UNIT ( $, .RADIAN. ) );
#16446=CARTESIAN_POINT ( 'NONE',  ( 31.24031073583692475, -4.273008382657478954, -3.627061608673664672 ) ) ;
#16448=ORIENTED_EDGE ( 'NONE', *, *, #47, .F. ) ;
#16449=ADVANCED_FACE ( 'NONE', ( #16278 ), #15078, .T. ) ;
#16450=CARTESIAN_POINT ( 'NONE',  ( 26.34507017448785504, -7.770415366711231009, -5.783357778048669573 ) ) ;
#16462=DIRECTION ( 'NONE',  ( 1.000000000000000000, 0.000000000000000000, 0.000000000000000000 ) ) ;
#16463=VECTOR ( 'NONE', #2200, 1000.000000000000000 ) ;
#16466=CARTESIAN_POINT ( 'NONE',  ( 31.55553118839817728, -4.235030543236534939, -7.939653947423662039 ) ) ;
#16470=CARTESIAN_POINT ( 'NONE',  ( 29.94002636988270538, -4.429666970165102136, -8.283357778048662468 ) ) ;
#16474=DIRECTION ( 'NONE',  ( 0.8243186046180107640, 0.5661261679878571984, 0.000000000000000000 ) ) ;
#16476=EDGE_LOOP ( 'NONE', ( #5553, #2506 ) ) ;
#16485=CARTESIAN_POINT ( 'NONE',  ( -50.00000000000000000, -16.03270077640482683, -5.537981825772250843 ) ) ;
#16488=CARTESIAN_POINT ( 'NONE',  ( 28.84872679426759845, -7.079226011327149237, -6.453230759126474148 ) ) ;
#16492=DIRECTION ( 'NONE',  ( 0.000000000000000000, 0.000000000000000000, -1.000000000000000000 ) ) ;
#16495=CARTESIAN_POINT ( 'NONE',  ( 31.69574812466957781, -6.726019302751734763, -5.783357778048669573 ) ) ;
#16499=CIRCLE ( 'NONE', #10966, 5.500000000000000888 ) ;
#16503=ORIENTED_EDGE ( 'NONE', *, *, #11669, .F. ) ;
#16505=CARTESIAN_POINT ( 'NONE',  ( 29.62489513447700062, -6.348545659133139729, -6.861505862736166250 ) ) ;
#16513=CARTESIAN_POINT ( 'NONE',  ( 28.09001152836989235, -6.106370808549102414, -8.283357778048662468 ) ) ;
#16514=ORIENTED_EDGE ( 'NONE', *, *, #985, .T. ) ;
#16524=CARTESIAN_POINT ( 'NONE',  ( 30.60493568430522160, -6.867637522466304212, -5.113484796970860558 ) ) ;
#16527=CARTESIAN_POINT ( 'NONE',  ( -27.94356719068602146, -12.38857420186734970, -13.73436385264702153 ) ) ;
#16529=CARTESIAN_POINT ( 'NONE',  ( 29.03376756790819613, -4.538853258604016006, -7.939653947423662039 ) ) ;
#16532=CARTESIAN_POINT ( 'NONE',  ( 27.57216386142120257, -6.895668018177890879, -7.033357778048666908 ) ) ;
#16549=CARTESIAN_POINT ( 'NONE',  ( 30.39102621733566423, -5.629271460726126719, -7.939653947423664704 ) ) ;
#16555=CARTESIAN_POINT ( 'NONE',  ( -25.11802603177690330, -16.03270077640482683, -0.5379818257722508434 ) ) ;
#16559=AXIS2_PLACEMENT_3D ( 'NONE', #2366, #10840, #2615 ) ;
#16562=ORIENTED_EDGE ( 'NONE', *, *, #17240, .F. ) ;
#16570=ORIENTED_EDGE ( 'NONE', *, *, #8693, .T. ) ;
#16574=CARTESIAN_POINT ( 'NONE',  ( 33.53059316159333036, -1.478995586096186532, -5.113484796970854340 ) ) ;
#16584=ORIENTED_EDGE ( 'NONE', *, *, #826, .F. ) ;
#16586=CARTESIAN_POINT ( 'NONE',  ( 27.65458886993626564, -2.824105456627233224, -6.861505862736158257 ) ) ;
#16590=VERTEX_POINT ( 'NONE', #8454 ) ;
#16593=ORIENTED_EDGE ( 'NONE', *, *, #3942, .F. ) ;
#16596=CARTESIAN_POINT ( 'NONE',  ( 28.24571643650507369, -4.633797857156355171, -7.939653947423662039 ) ) ;
#16606=CARTESIAN_POINT ( 'NONE',  ( 29.41846958523816724, -7.400131432564565515, -5.783357778048669573 ) ) ;
#16608=EDGE_CURVE ( 'NONE', #7736, #10032, #7918, .T. ) ;
#16609=CARTESIAN_POINT ( 'NONE',  ( 29.99682221560115991, -1.914942061115552541, -5.783357778048658027 ) ) ;
#16620=CARTESIAN_POINT ( 'NONE',  ( -20.00000000000000355, 7.999999999999996447, -6.000000000000000000 ) ) ;
#16621=ORIENTED_EDGE ( 'NONE', *, *, #3003, .T. ) ;
#16622=CARTESIAN_POINT ( 'NONE',  ( 28.71854711534694715, -4.576831098024959132, -3.627061608673664672 ) ) ;
#16626=CARTESIAN_POINT ( 'NONE',  ( 29.36638131047866196, -1.990897739957422807, -5.783357778048658027 ) ) ;
#16627=LINE ( 'NONE', #10973, #3466 ) ;
#16632=CARTESIAN_POINT ( 'NONE',  ( 22.22189723075623036, -22.43265299876153662, -15.08700452545048343 ) ) ;
#16637=EDGE_CURVE ( 'NONE', #13069, #5422, #16341, .T. ) ;
#16638=VERTEX_POINT ( 'NONE', #13992 ) ;
#16640=VERTEX_POINT ( 'NONE', #7108 ) ;
#16644=CARTESIAN_POINT ( 'NONE',  ( 26.51200394741821498, -4.842675973971495296, -7.939653947423662039 ) ) ;
#16649=CARTESIAN_POINT ( 'NONE',  ( 31.26353094466156080, -6.788289799823394866, -5.783357778048663356 ) ) ;
#16651=EDGE_CURVE ( 'NONE', #16638, #4798, #2193, .T. ) ;
#16666=DIRECTION ( 'NONE',  ( -0.1196152422706621005, 0.9928203230275509661, -0.000000000000000000 ) ) ;
#16674=CARTESIAN_POINT ( 'NONE',  ( 35.77680296528374271, -19.03270077640482683, -10.53798182577225084 ) ) ;
#16679=DIRECTION ( 'NONE',  ( -0.1196152422706621143, 0.9928203230275509661, 0.000000000000000000 ) ) ;
#16680=ORIENTED_EDGE ( 'NONE', *, *, #14916, .F. ) ;
#16681=VERTEX_POINT ( 'NONE', #3633 ) ;
#16684=CARTESIAN_POINT ( 'NONE',  ( 26.35439372113758694, -4.861664893681965083, -7.939653947423662039 ) ) ;
#16689=CARTESIAN_POINT ( 'NONE',  ( 31.05948030073166066, -1.776715885202022394, -5.783357778048662468 ) ) ;
#16691=CARTESIAN_POINT ( 'NONE',  ( 20.00000000000000000, 7.999999999999996447, -6.000000000000000000 ) ) ;
#16692=CARTESIAN_POINT ( 'NONE',  ( 29.91004888286193619, -6.613999042680076990, -4.533357778048668685 ) ) ;
#16693=CARTESIAN_POINT ( 'NONE',  ( 31.28415083292585663, -5.521667582366822202, -3.627061608673667781 ) ) ;
#16695=CARTESIAN_POINT ( 'NONE',  ( 26.55511561737958814, -2.656761491791831187, -7.033357778048658027 ) ) ;
#16696=DIRECTION ( 'NONE',  ( -1.000000000000000000, 0.000000000000000000, 0.000000000000000000 ) ) ;
#16708=DIRECTION ( 'NONE',  ( 0.000000000000000000, 0.000000000000000000, 1.000000000000000000 ) ) ;
#16710=CARTESIAN_POINT ( 'NONE',  ( 31.41531425212677675, -1.744041783721344219, -5.783357778048658915 ) ) ;
#16711=DIRECTION ( 'NONE',  ( 0.000000000000000000, 0.000000000000000000, 1.000000000000000000 ) ) ;
#16714=CARTESIAN_POINT ( 'NONE',  ( 30.01874226414561875, -2.539271660970221944, -6.861505862736159145 ) ) ;
#16717=ORIENTED_EDGE ( 'NONE', *, *, #16608, .F. ) ;
#16726=FACE_BOUND ( 'NONE', #4477, .T. ) ;
#16728=CARTESIAN_POINT ( 'NONE',  ( 32.58190297908952004, -5.565186596593329149, -8.283357778048664244 ) ) ;
#16732=CARTESIAN_POINT ( 'NONE',  ( 26.01127209431523113, -6.877383572197488526, -7.035051132944705188 ) ) ;
#16739=VECTOR ( 'NONE', #12596, 1000.000000000000000 ) ;
#16741=DIRECTION ( 'NONE',  ( 0.000000000000000000, 0.000000000000000000, 1.000000000000000000 ) ) ;
#16744=CIRCLE ( 'NONE', #7202, 6.249999999999998224 ) ;
#16747=SURFACE_STYLE_FILL_AREA ( #11372 ) ;
#16748=FACE_OUTER_BOUND ( 'NONE', #3037, .T. ) ;
#16755=DIRECTION ( 'NONE',  ( 0.9928203230275510771, 0.1196152422706614621, -0.000000000000000000 ) ) ;
#16759=FACE_OUTER_BOUND ( 'NONE', #14917, .T. ) ;
#16765=CARTESIAN_POINT ( 'NONE',  ( 30.48043329534786849, -5.818372192732907067, -3.283357778048667797 ) ) ;
#16768=ORIENTED_EDGE ( 'NONE', *, *, #10796, .F. ) ;
#16774=CARTESIAN_POINT ( 'NONE',  ( 26.01652455409633902, -4.902371455920928156, -5.783357778048663356 ) ) ;
#16775=DIRECTION ( 'NONE',  ( 0.000000000000000000, 0.000000000000000000, 1.000000000000000000 ) ) ;
#16779=CARTESIAN_POINT ( 'NONE',  ( 31.15208055228630357, -2.102918000029084578, -4.533357778048659803 ) ) ;
#16782=ORIENTED_EDGE ( 'NONE', *, *, #13199, .T. ) ;
#16785=CARTESIAN_POINT ( 'NONE',  ( 30.01512236704901682, -6.601339762873093875, -7.033357778048666908 ) ) ;
#16787=CARTESIAN_POINT ( 'NONE',  ( 28.73594040535616756, -2.066853418799292630, -5.783357778048658027 ) ) ;
#16797=ORIENTED_EDGE ( 'NONE', *, *, #6228, .T. ) ;
#16800=CARTESIAN_POINT ( 'NONE',  ( 29.71979337562451207, -1.938121702948446323, -5.783357778048664244 ) ) ;
#16802=EDGE_LOOP ( 'NONE', ( #5668, #17158, #8462, #4494, #1891, #12367, #546, #5716, #8598 ) ) ;
#16803=CARTESIAN_POINT ( 'NONE',  ( -24.42951923951777005, -10.13045284482685382, -14.60898600760630472 ) ) ;
#16807=CARTESIAN_POINT ( 'NONE',  ( 27.28266178881210280, -7.257709054644825741, -5.783357778048669573 ) ) ;
#16810=VECTOR ( 'NONE', #16384, 1000.000000000000227 ) ;
#16811=CARTESIAN_POINT ( 'NONE',  ( 31.91006497951310550, -2.311404624444611589, -6.861505862736159145 ) ) ;
#16813=DIRECTION ( 'NONE',  ( 0.000000000000000000, 0.000000000000000000, 1.000000000000000000 ) ) ;
#16817=CIRCLE ( 'NONE', #9280, 5.500000000000000000 ) ;
#16822=VERTEX_POINT ( 'NONE', #9609 ) ;
#16823=CARTESIAN_POINT ( 'NONE',  ( 26.24611652476386681, -6.808011323847543927, -7.414850139186299316 ) ) ;
#16825=CARTESIAN_POINT ( 'NONE',  ( -35.74085044863416272, -28.97437970944926988, -11.27079897466147607 ) ) ;
#16831=CARTESIAN_POINT ( 'NONE',  ( 33.48996557372703364, -1.821249024531260696, -7.033357778048658027 ) ) ;
#16832=CARTESIAN_POINT ( 'NONE',  ( 31.04700706809921940, -2.115577279836057922, -7.033357778048658027 ) ) ;
#16836=EDGE_CURVE ( 'NONE', #6589, #11736, #16441, .T. ) ;
#16838=VECTOR ( 'NONE', #8886, 1000.000000000000000 ) ;
#16839=CARTESIAN_POINT ( 'NONE',  ( 28.01872616749444944, -6.841866079205687790, -4.533357778048668685 ) ) ;
#16851=CARTESIAN_POINT ( 'NONE',  ( 34.91600907648203389, -11.88801210197604341, 0.000000000000000000 ) ) ;
#16857=EDGE_LOOP ( 'NONE', ( #859, #15835, #8579, #6256, #9222, #15472 ) ) ;
#16860=VECTOR ( 'NONE', #14210, 999.9999999999998863 ) ;
#16869=ORIENTED_EDGE ( 'NONE', *, *, #17716, .T. ) ;
#16871=ORIENTED_EDGE ( 'NONE', *, *, #1019, .F. ) ;
#16876=DIRECTION ( 'NONE',  ( -0.000000000000000000, -0.000000000000000000, -1.000000000000000000 ) ) ;
#16878=DIRECTION ( 'NONE',  ( 0.000000000000000000, 0.000000000000000000, 1.000000000000000000 ) ) ;
#16884=CARTESIAN_POINT ( 'NONE',  ( -23.02601376483258022, 3.965314980223224151, -6.000000000000000000 ) ) ;
#16886=ORIENTED_EDGE ( 'NONE', *, *, #12382, .F. ) ;
#16887=CARTESIAN_POINT ( 'NONE',  ( 31.51621784984448738, -6.120678622607529817, -6.861505862736166250 ) ) ;
#16890=CARTESIAN_POINT ( 'NONE',  ( 25.74999999999999289, -16.21813761408365195, -13.00000000000000178 ) ) ;
#16891=ORIENTED_EDGE ( 'NONE', *, *, #8915, .T. ) ;
#16893=AXIS2_PLACEMENT_3D ( 'NONE', #6576, #6660, #12191 ) ;
#16902=DIRECTION ( 'NONE',  ( 0.1195020427801297691, 0.9918807541847894926, -0.04349518650597275493 ) ) ;
#16903=ORIENTED_EDGE ( 'NONE', *, *, #15038, .T. ) ;
#16905=CARTESIAN_POINT ( 'NONE',  ( 27.25621498173240198, -3.499072175709823984, -3.627061608673662008 ) ) ;
#16907=( BOUNDED_CURVE ( )  B_SPLINE_CURVE ( 2, ( #11246, #1499, #14007, #11156, #1316, #16728, #2677, #8206, #13733 ),
 .UNSPECIFIED., .F., .T. ) 
 B_SPLINE_CURVE_WITH_KNOTS ( ( 3, 2, 2, 2, 3 ),
 ( 0.09615384615384617306, 0.1025641025641025605, 0.1153846153846153910, 0.1282051282051281937, 0.1346153846153846367 ),
 .UNSPECIFIED. ) 
 CURVE ( )  GEOMETRIC_REPRESENTATION_ITEM ( )  RATIONAL_B_SPLINE_CURVE ( ( 0.9330127018922194093, 0.9330127018922196314, 1.000000000000000000, 0.8660254037844387076, 1.000000000000000000, 0.8660254037844387076, 1.000000000000000000, 0.9330127018922190762, 0.9330127018922194093 ) ) 
 REPRESENTATION_ITEM ( '' )  );
#16908=EDGE_LOOP ( 'NONE', ( #9356, #7923, #8572, #2826 ) ) ;
#16909=CARTESIAN_POINT ( 'NONE',  ( 31.30154412293507349, -3.011689903141150815, -7.939653947423660263 ) ) ;
#16910=DIRECTION ( 'NONE',  ( -0.1196152422706611984, 0.9928203230275510771, 0.000000000000000000 ) ) ;
#16911=DIRECTION ( 'NONE',  ( -0.000000000000000000, 1.000000000000000000, 0.000000000000000000 ) ) ;
#16920=FACE_OUTER_BOUND ( 'NONE', #5137, .T. ) ;
#16922=ORIENTED_EDGE ( 'NONE', *, *, #6655, .T. ) ;
#16923=DIRECTION ( 'NONE',  ( 0.000000000000000000, 0.000000000000000000, 1.000000000000000000 ) ) ;
#16926=CARTESIAN_POINT ( 'NONE',  ( 33.45617745041539592, -1.098413033681664430, -5.783357778048658027 ) ) ;
#16931=CARTESIAN_POINT ( 'NONE',  ( 29.56783163384821833, -3.220568019956291383, -7.939653947423660263 ) ) ;
#16936=EDGE_CURVE ( 'NONE', #14370, #4798, #17405, .T. ) ;
#16951=ORIENTED_EDGE ( 'NONE', *, *, #9983, .F. ) ;
#16965=DIRECTION ( 'NONE',  ( -4.179998415399335043E-17, -3.469446951953615175E-16, 1.000000000000000000 ) ) ;
#16966=DIRECTION ( 'NONE',  ( 0.1113444980252557837, -0.9937818688019538493, 0.000000000000000000 ) ) ;
#16968=CARTESIAN_POINT ( 'NONE',  ( 31.68992120585416217, -1.700760206360153015, -5.783357778048664244 ) ) ;
#16970=CARTESIAN_POINT ( 'NONE',  ( 34.91600907648203389, -11.88801210197604341, -12.00000000000000000 ) ) ;
#16971=EDGE_CURVE ( 'NONE', #3112, #6328, #13978, .T. ) ;
#16972=DIRECTION ( 'NONE',  ( -0.000000000000000000, 0.000000000000000000, -1.000000000000000000 ) ) ;
#16974=CARTESIAN_POINT ( 'NONE',  ( 30.76748005699505129, -4.329975141788874993, -7.939653947423662039 ) ) ;
#16977=DIRECTION ( 'NONE',  ( -0.000000000000000000, -0.000000000000000000, -1.000000000000000000 ) ) ;
#16984=CARTESIAN_POINT ( 'NONE',  ( 33.60446413004628141, -3.988174587000466342, -3.627061608673664672 ) ) ;
#16985=EDGE_LOOP ( 'NONE', ( #4870, #10571, #405, #7384 ) ) ;
#16990=CARTESIAN_POINT ( 'NONE',  ( 26.65222088368961195, -7.333664733486695120, -5.783357778048669573 ) ) ;
#16992=CARTESIAN_POINT ( 'NONE',  ( 31.51621784984448738, -6.120678622607529817, -6.861505862736166250 ) ) ;
#16994=DIRECTION ( 'NONE',  ( 0.000000000000000000, 0.000000000000000000, 1.000000000000000000 ) ) ;
#16995=CARTESIAN_POINT ( 'NONE',  ( 32.89331279191618762, -2.620040694222726785, -8.283357778048660691 ) ) ;
#16999=EDGE_CURVE ( 'NONE', #11418, #7303, #17520, .T. ) ;
#17000=DIRECTION ( 'NONE',  ( -1.000000000000000000, 0.000000000000000000, 0.000000000000000000 ) ) ;
#17001=EDGE_CURVE ( 'NONE', #17122, #5005, #15432, .T. ) ;
#17010=DIRECTION ( 'NONE',  ( 0.9899494936611662466, -0.1414213562373111965, -0.000000000000000000 ) ) ;
#17015=CARTESIAN_POINT ( 'NONE',  ( 27.88665588685489993, -3.423116496867954162, -3.627061608673662008 ) ) ;
#17016=CARTESIAN_POINT ( 'NONE',  ( 32.90454166015506132, -1.164874252460851300, -5.783357778048658027 ) ) ;
#17019=DIRECTION ( 'NONE',  ( 1.000000000000000000, 0.000000000000000000, 0.000000000000000000 ) ) ;
#17020=CARTESIAN_POINT ( 'NONE',  ( 28.26310972651430120, -2.123820177930694442, -5.783357778048658027 ) ) ;
#17034=CARTESIAN_POINT ( 'NONE',  ( -5.500000000000000000, -20.49999999999999645, -6.000000000000000000 ) ) ;
#17035=CARTESIAN_POINT ( 'NONE',  ( 25.93714794488954212, -2.393855775999666591, -5.783357778048658027 ) ) ;
#17047=ORIENTED_EDGE ( 'NONE', *, *, #17001, .T. ) ;
#17048=VERTEX_POINT ( 'NONE', #11135 ) ;
#17051=ORIENTED_EDGE ( 'NONE', *, *, #6111, .F. ) ;
#17053=AXIS2_PLACEMENT_3D ( 'NONE', #1606, #14105, #10006 ) ;
#17055=CYLINDRICAL_SURFACE ( 'NONE', #16180, 2.499999999999999112 ) ;
#17057=CARTESIAN_POINT ( 'NONE',  ( -19.22707546753401786, -21.21757778339487288, -15.64731278403363035 ) ) ;
#17066=VERTEX_POINT ( 'NONE', #14256 ) ;
#17067=CARTESIAN_POINT ( 'NONE',  ( 28.23249303296521617, -2.754479417688857179, -4.705209693361161349 ) ) ;
#17068=LINE ( 'NONE', #15695, #14205 ) ;
#17075=AXIS2_PLACEMENT_3D ( 'NONE', #2630, #4072, #16418 ) ;
#17076=VERTEX_POINT ( 'NONE', #1654 ) ;
#17082=CARTESIAN_POINT ( 'NONE',  ( 25.76466184735054910, -2.811881907026620553, -6.248149982130924762 ) ) ;
#17085=CARTESIAN_POINT ( 'NONE',  ( 27.08121146544255353, -6.028038774645947839, -7.939653947423664704 ) ) ;
#17089=DIRECTION ( 'NONE',  ( 0.000000000000000000, 0.000000000000000000, -1.000000000000000000 ) ) ;
#17090=VERTEX_POINT ( 'NONE', #292 ) ;
#17105=CARTESIAN_POINT ( 'NONE',  ( 8.632250723006720250, -18.84644399697197770, -16.84735068286506987 ) ) ;
#17115=CARTESIAN_POINT ( 'NONE',  ( -29.25000000000000000, -16.21813761408365195, -13.37255996287876947 ) ) ;
#17117=VECTOR ( 'NONE', #15889, 1000.000000000000000 ) ;
#17118=EDGE_CURVE ( 'NONE', #4257, #16316, #11416, .T. ) ;
#17121=( BOUNDED_CURVE ( )  B_SPLINE_CURVE ( 2, ( #14888, #13353, #5345, #6367, #1201, #17739, #9176, #2474, #10780 ),
 .UNSPECIFIED., .F., .T. ) 
 B_SPLINE_CURVE_WITH_KNOTS ( ( 3, 2, 2, 2, 3 ),
 ( 0.4038461538461538547, 0.4102564102564102422, 0.4230769230769230727, 0.4358974358974359031, 0.4423076923076923461 ),
 .UNSPECIFIED. ) 
 CURVE ( )  GEOMETRIC_REPRESENTATION_ITEM ( )  RATIONAL_B_SPLINE_CURVE ( ( 0.9330127018922194093, 0.9330127018922196314, 1.000000000000000000, 0.8660254037844387076, 1.000000000000000000, 0.8660254037844387076, 1.000000000000000000, 0.9330127018922190762, 0.9330127018922194093 ) ) 
 REPRESENTATION_ITEM ( '' )  );
#17122=VERTEX_POINT ( 'NONE', #5959 ) ;
#17124=CYLINDRICAL_SURFACE ( 'NONE', #11022, 2.499999999999999112 ) ;
#17129=CARTESIAN_POINT ( 'NONE',  ( -2.749999999999992895, -20.49999999999999645, -13.00000000000000178 ) ) ;
#17131=ORIENTED_EDGE ( 'NONE', *, *, #3407, .F. ) ;
#17136=DIRECTION ( 'NONE',  ( -0.000000000000000000, -0.000000000000000000, -1.000000000000000000 ) ) ;
#17140=( BOUNDED_CURVE ( )  B_SPLINE_CURVE ( 2, ( #17035, #15662, #8779, #14312, #1895, #12935, #5673 ),
 .UNSPECIFIED., .F., .T. ) 
 B_SPLINE_CURVE_WITH_KNOTS ( ( 3, 2, 2, 3 ),
 ( 0.9423076923076922906, 0.9487179487179486781, 0.9615384615384615641, 0.9690340935984054216 ),
 .UNSPECIFIED. ) 
 CURVE ( )  GEOMETRIC_REPRESENTATION_ITEM ( )  RATIONAL_B_SPLINE_CURVE ( ( 0.9330127018922194093, 0.9330127018922194093, 1.000000000000000000, 0.8660254037844387076, 1.000000000000000000, 0.9216705062683109295, 0.9349331465915117212 ) ) 
 REPRESENTATION_ITEM ( '' )  );
#17151=CARTESIAN_POINT ( 'NONE',  ( -10.78415792467453471, 15.55827129984638901, -16.70145112110344598 ) ) ;
#17152=DIRECTION ( 'NONE',  ( 0.1113444980252557837, 0.9937818688019538493, 0.000000000000000000 ) ) ;
#17155=CARTESIAN_POINT ( 'NONE',  ( 31.05948030073166066, -1.776715885202022394, -5.783357778048662468 ) ) ;
#17158=ORIENTED_EDGE ( 'NONE', *, *, #13024, .F. ) ;
#17160=CYLINDRICAL_SURFACE ( 'NONE', #7296, 6.249999999999996447 ) ;
#17161=CARTESIAN_POINT ( 'NONE',  ( 26.16860980394290692, -3.430234601869349920, -3.283357778048662023 ) ) ;
#17163=CARTESIAN_POINT ( 'NONE',  ( 27.47505859511117521, -2.218764776483033163, -5.783357778048658027 ) ) ;
#17165=CARTESIAN_POINT ( 'NONE',  ( 26.19644603989335963, -6.395740563884607432, -4.006386918492157889 ) ) ;
#17170=CYLINDRICAL_SURFACE ( 'NONE', #14717, 2.499999999999999112 ) ;
#17171=B_SPLINE_CURVE_WITH_KNOTS ( 'NONE', 1,
 ( #5093, #16273 ),
 .UNSPECIFIED., .F., .F.,
 ( 2, 2 ),
 ( 0.000000000000000000, 1.000000000000000000 ),
 .UNSPECIFIED. ) ;
#17172=CARTESIAN_POINT ( 'NONE',  ( 31.91459173804835103, -5.445711903524953712, -3.627061608673667781 ) ) ;
#17175=LINE ( 'NONE', #3648, #5518 ) ;
#17176=CARTESIAN_POINT ( 'NONE',  ( 25.88432464927661769, -3.805096980563277498, -7.814840548041910750 ) ) ;
#17177=ORIENTED_EDGE ( 'NONE', *, *, #12068, .F. ) ;
#17178=EDGE_CURVE ( 'NONE', #3121, #14370, #7948, .T. ) ;
#17180=CARTESIAN_POINT ( 'NONE',  ( 25.76326615456878244, -3.051972493152843580, -6.861505862736158257 ) ) ;
#17181=AXIS2_PLACEMENT_3D ( 'NONE', #14283, #8922, #14462 ) ;
#17182=CARTESIAN_POINT ( 'NONE',  ( 26.45077056032005913, -6.103994453487816330, -7.939653947423664704 ) ) ;
#17183=DIRECTION ( 'NONE',  ( 0.000000000000000000, 1.000000000000000000, 0.000000000000000000 ) ) ;
#17184=CARTESIAN_POINT ( 'NONE',  ( 33.81344892038539740, -6.481075040654872943, -6.453230759126470595 ) ) ;
#17186=DIRECTION ( 'NONE',  ( -0.000000000000000000, -1.000000000000000000, -0.000000000000000000 ) ) ;
#17196=CARTESIAN_POINT ( 'NONE',  ( -15.92260893619738837, -28.39189527176317540, -16.15082599432113142 ) ) ;
#17198=EDGE_CURVE ( 'NONE', #17749, #11286, #1724, .T. ) ;
#17206=CARTESIAN_POINT ( 'NONE',  ( 29.15568435273173264, -2.343444316361667834, -7.033357778048658027 ) ) ;
#17217=( BOUNDED_CURVE ( )  B_SPLINE_CURVE ( 3, ( #12083, #10460, #9451, #10544 ),
 .UNSPECIFIED., .F., .T. ) 
 B_SPLINE_CURVE_WITH_KNOTS ( ( 4, 4 ),
 ( 4.774018107371971631, 4.846194975958193929 ),
 .UNSPECIFIED. ) 
 CURVE ( )  GEOMETRIC_REPRESENTATION_ITEM ( )  RATIONAL_B_SPLINE_CURVE ( ( 1.000000000000000000, 0.9995659220841806025, 0.9995659220841806025, 1.000000000000000000 ) ) 
 REPRESENTATION_ITEM ( '' )  );
#17225=DIRECTION ( 'NONE',  ( -0.000000000000000000, -0.000000000000000000, -1.000000000000000000 ) ) ;
#17227=ADVANCED_BREP_SHAPE_REPRESENTATION ( '', ( #11368, #3575 ), #2991 ) ;
#17228=ORIENTED_EDGE ( 'NONE', *, *, #13511, .F. ) ;
#17240=EDGE_CURVE ( 'NONE', #13718, #14027, #3789, .T. ) ;
#17242=ORIENTED_EDGE ( 'NONE', *, *, #10260, .F. ) ;
#17245=EDGE_LOOP ( 'NONE', ( #13931, #1233, #16562, #15706, #10988, #5558, #15168, #16448, #15351, #5982, #15579 ) ) ;
#17249=CARTESIAN_POINT ( 'NONE',  ( -17.83875296969244673, 10.53491135297441161, -15.87472302800564350 ) ) ;
#17250=CARTESIAN_POINT ( 'NONE',  ( -27.68843801662522353, -20.37088413741627235, -13.80304640004047023 ) ) ;
#17260=CARTESIAN_POINT ( 'NONE',  ( 33.56062403295735663, -2.739515387291124426, -3.627061608673662008 ) ) ;
#17266=CARTESIAN_POINT ( 'NONE',  ( 29.37220822929407760, -7.016156836349003001, -5.783357778048668685 ) ) ;
#17267=CARTESIAN_POINT ( 'NONE',  ( 32.12473870642251939, -5.420393343910986594, -7.939653947423662927 ) ) ;
#17269=CARTESIAN_POINT ( 'NONE',  ( 29.47916769939009285, -7.003270332485284300, -6.453230759126468818 ) ) ;
#17271=CARTESIAN_POINT ( 'NONE',  ( 31.29168529989541270, -6.784897756022354010, -6.453230759126470595 ) ) ;
#17272=CYLINDRICAL_SURFACE ( 'NONE', #10979, 2.749999999999992006 ) ;
#17276=CARTESIAN_POINT ( 'NONE',  ( 27.12505156253147476, -7.276697974355294640, -5.783357778048668685 ) ) ;
#17277=CARTESIAN_POINT ( 'NONE',  ( 28.12379965168153362, -6.829206799398704675, -7.033357778048666908 ) ) ;
#17279=CARTESIAN_POINT ( 'NONE',  ( 7.499998387031003411, -20.49508120620799900, -13.00000000000000178 ) ) ;
#17288=ORIENTED_EDGE ( 'NONE', *, *, #16362, .T. ) ;
#17292=CARTESIAN_POINT ( 'NONE',  ( 3.248936832696173393, 17.78798921770683350, -17.00000000000000000 ) ) ;
#17296=CARTESIAN_POINT ( 'NONE',  ( 30.57046727500519978, -4.353711291323232757, -8.283357778048662468 ) ) ;
#17299=FACE_OUTER_BOUND ( 'NONE', #5295, .T. ) ;
#17302=CARTESIAN_POINT ( 'NONE',  ( 33.95908713831673964, -3.945449517755637014, -5.783357778048663356 ) ) ;
#17316=CARTESIAN_POINT ( 'NONE',  ( 32.04575515724926760, -1.668086104879473730, -5.783357778048658027 ) ) ;
#17329=VECTOR ( 'NONE', #17526, 1000.000000000000000 ) ;
#17331=VERTEX_POINT ( 'NONE', #13022 ) ;
#17332=ADVANCED_FACE ( 'NONE', ( #1892 ), #8580, .T. ) ;
#17338=CARTESIAN_POINT ( 'NONE',  ( 0.000000000000000000, 0.000000000000000000, -10.50000000000000000 ) ) ;
#17339=CARTESIAN_POINT ( 'NONE',  ( -25.76436512043297711, -21.83811057962065405, -14.29411090273705831 ) ) ;
#17341=CARTESIAN_POINT ( 'NONE',  ( 31.20090818012769773, -4.277755612481361602, -8.283357778048662468 ) ) ;
#17346=CARTESIAN_POINT ( 'NONE',  ( 30.03080348965042745, -6.936809113706096319, -6.453230759126468818 ) ) ;
#17349=CARTESIAN_POINT ( 'NONE',  ( 27.73357241910951743, -6.576412695658750529, -6.861505862736166250 ) ) ;
#17351=ORIENTED_EDGE ( 'NONE', *, *, #6273, .T. ) ;
#17354=CARTESIAN_POINT ( 'NONE',  ( -25.74999999999999289, -16.21813761408365195, -13.00000000000000178 ) ) ;
#17355=CIRCLE ( 'NONE', #820, 2.749999999999991118 ) ;
#17359=B_SPLINE_CURVE_WITH_KNOTS ( 'NONE', 3,
 ( #2325, #13370, #6485, #1961 ),
 .UNSPECIFIED., .F., .F.,
 ( 4, 4 ),
 ( 0.000000000000000000, 0.0003446252387907819490 ),
 .UNSPECIFIED. ) ;
#17360=CARTESIAN_POINT ( 'NONE',  ( 29.11066736118121767, -3.075774767273946608, -8.283357778048660691 ) ) ;
#17363=CARTESIAN_POINT ( 'NONE',  ( 31.91006497951310550, -2.311404624444611589, -6.861505862736159145 ) ) ;
#17366=DIRECTION ( 'NONE',  ( -0.000000000000000000, 1.000000000000000000, -0.000000000000000000 ) ) ;
#17371=CARTESIAN_POINT ( 'NONE',  ( 31.66250999073069750, -5.675955295111851484, -3.283357778048667797 ) ) ;
#17372=ORIENTED_EDGE ( 'NONE', *, *, #13595, .T. ) ;
#17373=CARTESIAN_POINT ( 'NONE',  ( 25.72395281601508898, -4.937620572523835349, -7.939653947423662039 ) ) ;
#17385=CARTESIAN_POINT ( 'NONE',  ( 33.95908713831676096, -3.945449517755638791, -3.283357778048664688 ) ) ;
#17386=CIRCLE ( 'NONE', #12426, 14.00000000000000178 ) ;
#17390=CARTESIAN_POINT ( 'NONE',  ( 32.07220196432898263, -5.426722983814484813, -3.627061608673668225 ) ) ;
#17393=CIRCLE ( 'NONE', #15622, 2.000000000000001776 ) ;
#17394=CARTESIAN_POINT ( 'NONE',  ( 28.72797218747911074, -6.756415940301135237, -4.533357778048668685 ) ) ;
#17403=VECTOR ( 'NONE', #10480, 1000.000000000000227 ) ;
#17405=LINE ( 'NONE', #10784, #9047 ) ;
#17407=ORIENTED_EDGE ( 'NONE', *, *, #14606, .F. ) ;
#17411=ORIENTED_EDGE ( 'NONE', *, *, #5600, .F. ) ;
#17412=CARTESIAN_POINT ( 'NONE',  ( 26.31175009776946538, -7.352777558617343168, -6.181997573440047411 ) ) ;
#17415=CARTESIAN_POINT ( 'NONE',  ( 33.43363050022580296, -2.127845067243429256, -4.705209693361160461 ) ) ;
#17416=EDGE_CURVE ( 'NONE', #8021, #1670, #11561, .T. ) ;
#17422=CARTESIAN_POINT ( 'NONE',  ( 31.34233605952372415, -6.778795339760710803, -5.783357778048663356 ) ) ;
#17423=CARTESIAN_POINT ( 'NONE',  ( 31.84257795004536007, -2.746633492292519296, -3.283357778048662023 ) ) ;
#17425=ORIENTED_EDGE ( 'NONE', *, *, #6293, .F. ) ;
#17427=ORIENTED_EDGE ( 'NONE', *, *, #6917, .T. ) ;
#17430=EDGE_CURVE ( 'NONE', #548, #2553, #6353, .T. ) ;
#17432=CARTESIAN_POINT ( 'NONE',  ( 23.02601376483258022, 3.965314980223224151, 0.000000000000000000 ) ) ;
#17434=ORIENTED_EDGE ( 'NONE', *, *, #1433, .F. ) ;
#17438=CARTESIAN_POINT ( 'NONE',  ( -17.59998316743469715, -19.37170218437266200, -15.90983619775817459 ) ) ;
#17441=CARTESIAN_POINT ( 'NONE',  ( 35.74085044863416982, -18.73429073671341172, -11.27079897466147251 ) ) ;
#17443=LINE ( 'NONE', #6526, #11039 ) ;
#17445=AXIS2_PLACEMENT_3D ( 'NONE', #15526, #10069, #16994 ) ;
#17447=CARTESIAN_POINT ( 'NONE',  ( 28.24571643650507369, -4.633797857156355171, -7.939653947423662039 ) ) ;
#17449=ORIENTED_EDGE ( 'NONE', *, *, #12039, .T. ) ;
#17450=DIRECTION ( 'NONE',  ( -0.1196152422706611984, 0.9928203230275510771, 0.000000000000000000 ) ) ;
#17453=EDGE_CURVE ( 'NONE', #15678, #15612, #14668, .T. ) ;
#17456=EDGE_CURVE ( 'NONE', #17637, #12969, #206, .T. ) ;
#17457=CIRCLE ( 'NONE', #1207, 2.749999999999988454 ) ;
#17458=CARTESIAN_POINT ( 'NONE',  ( 33.38562051666750818, -5.268481986227246949, -7.939653947423662927 ) ) ;
#17460=CARTESIAN_POINT ( 'NONE',  ( 29.16815758536418102, -2.004582921727632971, -5.783357778048664244 ) ) ;
#17465=CARTESIAN_POINT ( 'NONE',  ( 31.94023320572814484, -7.096308717197083560, -5.783357778048669573 ) ) ;
#17467=CARTESIAN_POINT ( 'NONE',  ( 28.97253418081003673, -5.800171738120336151, -7.939653947423664704 ) ) ;
#17472=ORIENTED_EDGE ( 'NONE', *, *, #13518, .F. ) ;
#17477=EDGE_CURVE ( 'NONE', #15522, #10591, #5374, .T. ) ;
#17478=B_SPLINE_CURVE_WITH_KNOTS ( 'NONE', 3,
 ( #17105, #12911, #15455, #8837 ),
 .UNSPECIFIED., .F., .F.,
 ( 4, 4 ),
 ( 0.004328141481285538092, 0.004974662558709086295 ),
 .UNSPECIFIED. ) ;
#17487=CARTESIAN_POINT ( 'NONE',  ( 33.56062403295735663, -2.739515387291123982, -3.627061608673662008 ) ) ;
#17492=ADVANCED_FACE ( 'NONE', ( #17768 ), #9376, .F. ) ;
#17493=CARTESIAN_POINT ( 'NONE',  ( 27.23057351405260818, -1.848475362037681480, -5.783357778048658027 ) ) ;
#17501=CARTESIAN_POINT ( 'NONE',  ( 27.11643206945770146, -20.93856092459426677, -13.95341982493238753 ) ) ;
#17502=AXIS2_PLACEMENT_3D ( 'NONE', #7329, #12846, #6028 ) ;
#17505=( BOUNDED_CURVE ( )  B_SPLINE_CURVE ( 2, ( #181, #12602, #5604, #8607, #11120, #1729, #16779, #7259, #16689 ),
 .UNSPECIFIED., .F., .T. ) 
 B_SPLINE_CURVE_WITH_KNOTS ( ( 3, 2, 2, 2, 3 ),
 ( 0.2115384615384615641, 0.2179487179487179516, 0.2307692307692307820, 0.2435897435897435848, 0.2500000000000000000 ),
 .UNSPECIFIED. ) 
 CURVE ( )  GEOMETRIC_REPRESENTATION_ITEM ( )  RATIONAL_B_SPLINE_CURVE ( ( 0.9330127018922194093, 0.9330127018922196314, 1.000000000000000000, 0.8660254037844387076, 1.000000000000000000, 0.8660254037844387076, 1.000000000000000000, 0.9330127018922191873, 0.9330127018922194093 ) ) 
 REPRESENTATION_ITEM ( '' )  );
#17512=ORIENTED_EDGE ( 'NONE', *, *, #9645, .T. ) ;
#17517=CARTESIAN_POINT ( 'NONE',  ( 32.30426898124760982, -6.025734024055190652, -6.861505862736167138 ) ) ;
#17519=CYLINDRICAL_SURFACE ( 'NONE', #6032, 2.749999999999992006 ) ;
#17520=CIRCLE ( 'NONE', #15746, 5.000000000000000000 ) ;
#17521=LINE ( 'NONE', #9136, #17403 ) ;
#17526=DIRECTION ( 'NONE',  ( 0.000000000000000000, 0.000000000000000000, -1.000000000000000000 ) ) ;
#17533=CARTESIAN_POINT ( 'NONE',  ( 26.01652455409633902, -4.902371455920928156, -5.783357778048663356 ) ) ;
#17534=VECTOR ( 'NONE', #17225, 1000.000000000000000 ) ;
#17546=CARTESIAN_POINT ( 'NONE',  ( 31.45915434921569798, -2.992700983430681028, -7.939653947423660263 ) ) ;
#17551=EDGE_CURVE ( 'NONE', #4281, #11111, #7027, .T. ) ;
#17553=VERTEX_POINT ( 'NONE', #970 ) ;
#17555=CARTESIAN_POINT ( 'NONE',  ( 33.17547354829333983, -5.293800545841212291, -3.627061608673667781 ) ) ;
#17559=CARTESIAN_POINT ( 'NONE',  ( 26.16909369068367752, -6.168712907020689862, -7.925803108758818105 ) ) ;
#17562=CARTESIAN_POINT ( 'NONE',  ( 33.06225340847440464, -6.234220648470727433, -4.533357778048668685 ) ) ;
#17563=ORIENTED_EDGE ( 'NONE', *, *, #11046, .F. ) ;
#17564=CARTESIAN_POINT ( 'NONE',  ( 32.75517961154501023, -5.344437665069116328, -7.939653947423664704 ) ) ;
#17567=CARTESIAN_POINT ( 'NONE',  ( 13.34918303132433692, 14.15390528054681596, -16.46429318744779025 ) ) ;
#17570=EDGE_CURVE ( 'NONE', #2553, #17048, #13478, .T. ) ;
#17571=ORIENTED_EDGE ( 'NONE', *, *, #13855, .F. ) ;
#17574=VERTEX_POINT ( 'NONE', #5825 ) ;
#17575=DIRECTION ( 'NONE',  ( 0.000000000000000000, 0.000000000000000000, 1.000000000000000000 ) ) ;
#17578=DIRECTION ( 'NONE',  ( -0.000000000000000000, 1.000000000000000000, -0.000000000000000000 ) ) ;
#17580=CARTESIAN_POINT ( 'NONE',  ( 30.06013935859953534, -5.869009311960810216, -8.283357778048662468 ) ) ;
#17582=CARTESIAN_POINT ( 'NONE',  ( -3.248936832696171617, -20.49508120620799900, 78.00000000000000000 ) ) ;
#17587=CARTESIAN_POINT ( 'NONE',  ( 27.69265652961275848, -20.36619546179435503, -13.80192434669152490 ) ) ;
#17598=ORIENTED_EDGE ( 'NONE', *, *, #17456, .T. ) ;
#17600=FACE_OUTER_BOUND ( 'NONE', #167, .T. ) ;
#17613=ORIENTED_EDGE ( 'NONE', *, *, #12370, .F. ) ;
#17614=EDGE_LOOP ( 'NONE', ( #11944, #15929, #13495 ) ) ;
#17617=AXIS2_PLACEMENT_3D ( 'NONE', #15157, #11048, #1559 ) ;
#17618=EDGE_LOOP ( 'NONE', ( #14578, #4382 ) ) ;
#17628=CARTESIAN_POINT ( 'NONE',  ( 26.41562710823574278, -3.600346414165641828, -7.939653947423660263 ) ) ;
#17631=CARTESIAN_POINT ( 'NONE',  ( 30.82871344409320713, -3.068656662272551738, -7.939653947423660263 ) ) ;
#17634=DIRECTION ( 'NONE',  ( -0.1196152422706611984, 0.9928203230275510771, 0.000000000000000000 ) ) ;
#17637=VERTEX_POINT ( 'NONE', #4126 ) ;
#17639=CARTESIAN_POINT ( 'NONE',  ( 29.64681518302145946, -6.972875258987813574, -5.783357778048668685 ) ) ;
#17640=EDGE_CURVE ( 'NONE', #6789, #1845, #16907, .T. ) ;
#17643=DIRECTION ( 'NONE',  ( -0.7866107318554605987, 0.6174492339697383869, 8.659560562354860135E-17 ) ) ;
#17645=CARTESIAN_POINT ( 'NONE',  ( 31.75254397038802878, -4.211294393702175398, -8.283357778048662468 ) ) ;
#17646=EDGE_CURVE ( 'NONE', #15348, #5172, #10882, .T. ) ;
#17655=AXIS2_PLACEMENT_3D ( 'NONE', #270, #5875, #538 ) ;
#17657=DIRECTION ( 'NONE',  ( 0.000000000000000000, 0.000000000000000000, 1.000000000000000000 ) ) ;
#17658=CARTESIAN_POINT ( 'NONE',  ( -28.41103551745680633, -13.06362195986656616, -13.60745115249024728 ) ) ;
#17663=CARTESIAN_POINT ( 'NONE',  ( 32.29974222271236073, -2.891426744974864071, -3.627061608673662008 ) ) ;
#17665=CARTESIAN_POINT ( 'NONE',  ( 26.60013260893011378, -1.924431040879551746, -5.783357778048658027 ) ) ;
#17680=VERTEX_POINT ( 'NONE', #4744 ) ;
#17684=EDGE_LOOP ( 'NONE', ( #8019, #16886, #13286, #9627, #15722, #16782, #170, #2356, #3723, #14520, #10183, #14134, #17512, #754, #8594 ) ) ;
#17686=CARTESIAN_POINT ( 'NONE',  ( 29.80442540930208750, -6.953886339277345563, -5.783357778048669573 ) ) ;
#17687=CARTESIAN_POINT ( 'NONE',  ( 30.74004950963507810, -6.851358974801540214, -6.453230759126470595 ) ) ;
#17690=AXIS2_PLACEMENT_3D ( 'NONE', #15254, #16911, #16813 ) ;
#17693=CARTESIAN_POINT ( 'NONE',  ( 31.31418170428987224, -6.782187383561751659, -5.113484796970860558 ) ) ;
#17702=EDGE_CURVE ( 'NONE', #15783, #8066, #762, .T. ) ;
#17708=CARTESIAN_POINT ( 'NONE',  ( 29.84999239022537409, -5.894327871574777333, -3.283357778048667797 ) ) ;
#17716=EDGE_CURVE ( 'NONE', #4517, #11475, #77, .T. ) ;
#17717=CARTESIAN_POINT ( 'NONE',  ( 30.60986983071443390, -4.348964061499348333, -3.627061608673664672 ) ) ;
#17721=CYLINDRICAL_SURFACE ( 'NONE', #15304, 2.499999999999999112 ) ;
#17722=DIRECTION ( 'NONE',  ( -0.000000000000000000, -1.000000000000000000, -0.000000000000000000 ) ) ;
#17727=CARTESIAN_POINT ( 'NONE',  ( 27.51889869220010354, -3.467423976192371526, -7.939653947423660263 ) ) ;
#17733=CARTESIAN_POINT ( 'NONE',  ( 32.93004296264515318, -25.68697430340742471, -12.29384923381407546 ) ) ;
#17734=CARTESIAN_POINT ( 'NONE',  ( 29.95125523467787687, -2.974500528818130096, -3.283357778048662023 ) ) ;
#17739=CARTESIAN_POINT ( 'NONE',  ( 30.61177514885986639, -5.802548093181622235, -8.283357778048664244 ) ) ;
#17748=DIRECTION ( 'NONE',  ( 1.000000000000000000, 0.000000000000000000, 0.000000000000000000 ) ) ;
#17749=VERTEX_POINT ( 'NONE', #17385 ) ;
#17750=CARTESIAN_POINT ( 'NONE',  ( 30.40841950734487753, -3.119293781500474427, -3.627061608673662008 ) ) ;
#17753=CARTESIAN_POINT ( 'NONE',  ( 33.17094678975809074, -2.159493266760871499, -6.861505862736159145 ) ) ;
#17760=CARTESIAN_POINT ( 'NONE',  ( 29.08710323061924896, -17.65086537115787380, -13.41876697690134179 ) ) ;
#17762=ORIENTED_EDGE ( 'NONE', *, *, #16280, .T. ) ;
#17768=FACE_OUTER_BOUND ( 'NONE', #13178, .T. ) ;
#17772=DIRECTION ( 'NONE',  ( 0.9928203230275512992, 0.1196152422706614898, -0.000000000000000000 ) ) ;
#17774=ORIENTED_EDGE ( 'NONE', *, *, #7991, .F. ) ;
#17776=DIRECTION ( 'NONE',  ( 0.1196152422706621143, 0.9928203230275509661, 0.000000000000000000 ) ) ;
#17777=CARTESIAN_POINT ( 'NONE',  ( 29.13014440709066832, -5.781182818409868140, -7.939653947423664704 ) ) ;
#17778=FACE_OUTER_BOUND ( 'NONE', #3498, .T. ) ;
#17779=FACE_OUTER_BOUND ( 'NONE', #12366, .T. ) ;
#17785=VECTOR ( 'NONE', #6019, 1000.000000000000000 ) ;
#17787=ORIENTED_EDGE ( 'NONE', *, *, #11835, .T. ) ;
#17802=CARTESIAN_POINT ( 'NONE',  ( 29.04511322243489602, -14.57839366656647506, -13.43065377816253481 ) ) ;
#17803=DIRECTION ( 'NONE',  ( -0.000000000000000000, -0.000000000000000000, -1.000000000000000000 ) ) ;
#17806=CARTESIAN_POINT ( 'NONE',  ( 31.43723430067123914, -2.368371383576012956, -6.861505862736158257 ) ) ;
#17808=DIRECTION ( 'NONE',  ( -0.000000000000000000, 0.000000000000000000, -1.000000000000000000 ) ) ;
#17811=( BOUNDED_CURVE ( )  B_SPLINE_CURVE ( 2, ( #13270, #17487, #10618, #16190, #14901, #9274, #3664, #3484, #9189, #7662, #14816, #5015, #2406, #10702, #11812, #7928, #13461, #13544, #1120, #6644, #6557, #12077, #2144, #12172, #11904, #17663, #4830, #765, #15911, #9015, #14566, #9107, #16010, #13187, #3585, #17390, #4923, #10451, #14647, #16710, #15170, #11141, #15248, #1387, #9700, #10876, #2829, #4283, #16446, #6732, #5275, #6910, #1574, #9788, #12349, #16369, #3932, #4108, #15341, #2919, #7107, #17750, #5448, #4200, #8270, #13719, #2751, #9530, #26, #9444, #2661, #10792, #14982, #17917, #13802, #4014, #8357, #13888, #6824, #8453, #12439, #11062, #5537, #1477, #2569, #8096, #8193, #10968, #7007, #13631, #16529, #1301, #1217, #12270, #17839, #9616, #16622, #5357, #12532, #116, #5623, #13990, #15075, #5809, #12981, #396, #4727, #1939, #15438, #11425, #9973, #10250, #15800, #14076, #11329, #3021, #1852, #3374, #8543, #5986, #8907, #16905, #4636, #8821, #1755, #14442, #7380, #12706, #2025, #16807, #11614, #10162, #1661, #12621, #7196, #12802, #15711, #7457, #298, #5902, #565, #16990, #4545, #4461, #11512, #3290, #6085, #15523, #17082 ),
 .UNSPECIFIED., .F., .T. ) 
 B_SPLINE_CURVE_WITH_KNOTS ( ( 3, 2, 2, 2, 2, 2, 2, 2, 2, 2, 2, 2, 2, 2, 2, 2, 2, 2, 2, 2, 2, 2, 2, 2, 2, 2, 2, 2, 2, 2, 2, 2, 2, 2, 2, 2, 2, 2, 2, 2, 2, 2, 2, 2, 2, 2, 2, 2, 2, 2, 2, 2, 2, 2, 2, 2, 2, 2, 2, 2, 2, 2, 2, 2, 2, 2, 2, 2, 2, 2, 2, 2, 2, 2, 3 ),
 ( 0.000000000000000000, 0.01322951878407230102, 0.02645903756814460203, 0.03968855635221691519, 0.05291807513628920406, 0.06614759392036151375, 0.07937711270443383038, 0.09260663148850611925, 0.1058361502725784081, 0.1190656690566507248, 0.1322951878407230275, 0.1455247066247953303, 0.1587542254088676608, 0.1719837441929399358, 0.1852132629770122385, 0.1984427817610845690, 0.2116723005451568163, 0.2249018193292291468, 0.2381313381133014495, 0.2513608568973737523, 0.2645903756814460550, 0.2778198944655183578, 0.2910494132495906605, 0.3042789320336629633, 0.3175084508177353215, 0.3307379696018076243, 0.3439674883858798715, 0.3571970071699521743, 0.3704265259540244770, 0.3836560447380968353, 0.3968855635221691380, 0.4101150823062413853, 0.4233446010903136325, 0.4365741198743859908, 0.4498036386584582935, 0.4630331574425305963, 0.4762626762266028990, 0.4894921950106752018, 0.5027217137947475045, 0.5159512325788198073, 0.5291807513628921100, 0.5424102701469644128, 0.5556397889310367155, 0.5688693077151090183, 0.5820988264991813210, 0.5953283452832536238, 0.6085578640673259265, 0.6217873828513982293, 0.6350169016354706431, 0.6482464204195428348, 0.6614759392036152486, 0.6747054579876874403, 0.6879349767717597430, 0.7011644955558321568, 0.7143940143399043485, 0.7276235331239767623, 0.7408530519080489540, 0.7540825706921212568, 0.7673120894761936706, 0.7805416082602658623, 0.7937711270443382761, 0.8070006458284105788, 0.8202301646124827705, 0.8334596833965551843, 0.8466892021806272650, 0.8599187209646996788, 0.8731482397487719815, 0.8863777585328441733, 0.8996072773169165870, 0.9128367961009887788, 0.9260663148850611925, 0.9392958336691334953, 0.9525253524532057980, 0.9657548712372781008, 0.9750618896629086318 ),
 .UNSPECIFIED. ) 
 CURVE ( )  GEOMETRIC_REPRESENTATION_ITEM ( )  RATIONAL_B_SPLINE_CURVE ( ( 1.000000000000000000, 0.8660254037844387076, 1.000000000000000000, 0.8660254037844387076, 1.000000000000000000, 0.8660254037844387076, 1.000000000000000000, 0.8660254037844387076, 1.000000000000000000, 0.8660254037844387076, 1.000000000000000000, 0.8660254037844387076, 1.000000000000000000, 0.8660254037844387076, 1.000000000000000000, 0.8660254037844387076, 1.000000000000000000, 0.8660254037844387076, 1.000000000000000000, 0.8660254037844387076, 1.000000000000000000, 0.8660254037844387076, 1.000000000000000000, 0.8660254037844387076, 1.000000000000000000, 0.8660254037844387076, 1.000000000000000000, 0.8660254037844387076, 1.000000000000000000, 0.8660254037844387076, 1.000000000000000000, 0.8660254037844387076, 1.000000000000000000, 0.8660254037844387076, 1.000000000000000000, 0.8660254037844387076, 1.000000000000000000, 0.8660254037844387076, 1.000000000000000000, 0.8660254037844387076, 1.000000000000000000, 0.8660254037844387076, 1.000000000000000000, 0.8660254037844387076, 1.000000000000000000, 0.8660254037844387076, 1.000000000000000000, 0.8660254037844387076, 1.000000000000000000, 0.8660254037844387076, 1.000000000000000000, 0.8660254037844387076, 1.000000000000000000, 0.8660254037844387076, 1.000000000000000000, 0.8660254037844387076, 1.000000000000000000, 0.8660254037844387076, 1.000000000000000000, 0.8660254037844387076, 1.000000000000000000, 0.8660254037844387076, 1.000000000000000000, 0.8660254037844387076, 1.000000000000000000, 0.8660254037844387076, 1.000000000000000000, 0.8660254037844387076, 1.000000000000000000, 0.8660254037844387076, 1.000000000000000000, 0.8660254037844387076, 1.000000000000000000, 0.8660254037844387076, 1.000000000000000000, 0.8660254037844387076, 1.000000000000000000, 0.8660254037844387076, 1.000000000000000000, 0.8660254037844387076, 1.000000000000000000, 0.8660254037844387076, 1.000000000000000000, 0.8660254037844387076, 1.000000000000000000, 0.8660254037844387076, 1.000000000000000000, 0.8660254037844387076, 1.000000000000000000, 0.8660254037844387076, 1.000000000000000000, 0.8660254037844387076, 1.000000000000000000, 0.8660254037844387076, 1.000000000000000000, 0.8660254037844387076, 1.000000000000000000, 0.8660254037844387076, 1.000000000000000000, 0.8660254037844387076, 1.000000000000000000, 0.8660254037844387076, 1.000000000000000000, 0.8660254037844387076, 1.000000000000000000, 0.8660254037844387076, 1.000000000000000000, 0.8660254037844387076, 1.000000000000000000, 0.8660254037844387076, 1.000000000000000000, 0.8660254037844387076, 1.000000000000000000, 0.8660254037844387076, 1.000000000000000000, 0.8660254037844387076, 1.000000000000000000, 0.8660254037844387076, 1.000000000000000000, 0.8660254037844387076, 1.000000000000000000, 0.8660254037844387076, 1.000000000000000000, 0.8660254037844387076, 1.000000000000000000, 0.8660254037844387076, 1.000000000000000000, 0.8660254037844387076, 1.000000000000000000, 0.8660254037844387076, 1.000000000000000000, 0.8660254037844387076, 1.000000000000000000, 0.8660254037844387076, 1.000000000000000000, 0.8660254037844387076, 1.000000000000000000, 0.8660254037844387076, 1.000000000000000000, 0.8660254037844387076, 1.000000000000000000, 0.8660254037844387076, 1.000000000000000000, 0.8660254037844387076, 1.000000000000000000, 0.8660254037844387076, 1.000000000000000000, 0.9057483453558528019, 0.9441095091726994237 ) ) 
 REPRESENTATION_ITEM ( '' )  );
#17814=CARTESIAN_POINT ( 'NONE',  ( 30.27725608814395386, -6.896919580145944195, -5.783357778048668685 ) ) ;
#17820=CARTESIAN_POINT ( 'NONE',  ( 28.36392410707646761, -4.619556167269785796, -3.283357778048664688 ) ) ;
#17821=CARTESIAN_POINT ( 'NONE',  ( -29.25000000000000000, -16.21813761408365195, -13.00000000000000178 ) ) ;
#17822=CARTESIAN_POINT ( 'NONE',  ( 26.70901672940806648, -4.818939824437135755, -8.283357778048662468 ) ) ;
#17823=ORIENTED_EDGE ( 'NONE', *, *, #14, .F. ) ;
#17830=B_SPLINE_CURVE_WITH_KNOTS ( 'NONE', 3,
 ( #8268, #7921, #6821, #9270, #5271, #12347, #13455, #8091, #17658, #17913, #16527, #5179, #14898, #3929, #13627, #6727, #2916, #4541, #11327, #14074, #16803, #3102, #9882, #13988, #8629, #1474, #4280, #5713, #9971, #1752, #11423, #294, #5806, #5535, #7281, #15435, #12529, #1848, #3189, #12799, #11060, #8355, #15611, #7005 ),
 .UNSPECIFIED., .F., .F.,
 ( 4, 2, 2, 2, 2, 2, 2, 2, 2, 2, 2, 2, 2, 2, 2, 2, 2, 2, 2, 2, 2, 4 ),
 ( 0.000000000000000000, 0.001235571410315390150, 0.001853357115473088478, 0.002471142820630786805, 0.003706714230946187797, 0.004324499936103893064, 0.004942285641261598764, 0.006177857051577013633, 0.007413428461892427636, 0.008031214167050130734, 0.008648999872207834699, 0.009884571282523253039, 0.01112014269283866964, 0.01235571410315408972, 0.01297349980831179542, 0.01359128551346949765, 0.01482685692378490731, 0.01606242833410031698, 0.01668021403925802268, 0.01729799974441572491, 0.01853357115473113284, 0.01976914256504654077 ),
 .UNSPECIFIED. ) ;
#17834=CARTESIAN_POINT ( 'NONE',  ( 8.632250723006720250, -18.84644399697197770, -16.84735068286506987 ) ) ;
#17835=ORIENTED_EDGE ( 'NONE', *, *, #17118, .T. ) ;
#17838=ADVANCED_FACE ( 'NONE', ( #492 ), #15908, .F. ) ;
#17839=CARTESIAN_POINT ( 'NONE',  ( 29.04699097144805364, -6.418171698071525100, -4.705209693361169343 ) ) ;
#17840=CARTESIAN_POINT ( 'NONE',  ( -6.935828204433864386, -17.68137362934027479, -16.94363565911716663 ) ) ;
#17841=EDGE_LOOP ( 'NONE', ( #12433, #13510, #11604, #25 ) ) ;
#17842=CARTESIAN_POINT ( 'NONE',  ( 33.19286683830256379, -2.783822866615540903, -7.939653947423660263 ) ) ;
#17849=VERTEX_POINT ( 'NONE', #8835 ) ;
#17852=CARTESIAN_POINT ( 'NONE',  ( 23.00000000000000000, -16.21813761408365195, -13.00000000000000355 ) ) ;
#17853=ORIENTED_EDGE ( 'NONE', *, *, #5600, .T. ) ;
#17854=CARTESIAN_POINT ( 'NONE',  ( 0.000000000000000000, 0.000000000000000000, -8.700000000000001066 ) ) ;
#17860=CARTESIAN_POINT ( 'NONE',  ( 28.26310972651430120, -2.123820177930694442, -5.783357778048658027 ) ) ;
#17867=DIRECTION ( 'NONE',  ( 1.000000000000000000, 0.000000000000000000, 0.000000000000000000 ) ) ;
#17878=CARTESIAN_POINT ( 'NONE',  ( 27.57216386142120257, -6.895668018177890879, -7.033357778048666908 ) ) ;
#17883=CARTESIAN_POINT ( 'NONE',  ( 18.90607966454165734, -11.47788193099826692, -15.70134094032044736 ) ) ;
#17884=DIRECTION ( 'NONE',  ( -1.000000000000000000, 0.000000000000000000, 0.000000000000000000 ) ) ;
#17886=CARTESIAN_POINT ( 'NONE',  ( 32.91278983782564183, -5.325448745358647429, -7.939653947423664704 ) ) ;
#17888=CARTESIAN_POINT ( 'NONE',  ( 25.71748644841968456, -2.420320648352051851, -5.783357778048663356 ) ) ;
#17893=CARTESIAN_POINT ( 'NONE',  ( 27.10313151398701947, -6.652368374500619908, -6.861505862736166250 ) ) ;
#17899=LINE ( 'NONE', #9768, #7003 ) ;
#17900=CARTESIAN_POINT ( 'NONE',  ( 27.92107091181166467, -2.492190854301117753, -4.533357778048659803 ) ) ;
#17901=PRODUCT_DEFINITION_FORMATION_WITH_SPECIFIED_SOURCE ( 'ANY', '', #11993, .NOT_KNOWN. ) ;
#17904=CARTESIAN_POINT ( 'NONE',  ( 27.90727577511918867, -2.156494279411373061, -5.783357778048670461 ) ) ;
#17905=FACE_OUTER_BOUND ( 'NONE', #9906, .T. ) ;
#17909=EDGE_CURVE ( 'NONE', #4619, #7917, #4715, .T. ) ;
#17912=EDGE_LOOP ( 'NONE', ( #5829, #7139 ) ) ;
#17913=CARTESIAN_POINT ( 'NONE',  ( -28.06754645621478517, -12.55420304724502323, -13.70087619851170757 ) ) ;
#17917=CARTESIAN_POINT ( 'NONE',  ( 29.77797860222238313, -3.195249460342344250, -3.627061608673662008 ) ) ;
#17920=EDGE_LOOP ( 'NONE', ( #17472, #2377, #4770, #2985 ) ) ;
#17921=CARTESIAN_POINT ( 'NONE',  ( 26.24741491880507027, -3.420740141806666745, -3.283357778048662023 ) ) ;
#17922=CARTESIAN_POINT ( 'NONE',  ( -15.92260893619738837, -28.39189527176317540, -16.15082599432113142 ) ) ;
#17926=CARTESIAN_POINT ( 'NONE',  ( 29.18195272205665347, -2.340279496617377664, -4.533357778048659803 ) ) ;
#17929=AXIS2_PLACEMENT_3D ( 'NONE', #5479, #12472, #15196 ) ;
#17934=AXIS2_PLACEMENT_3D ( 'NONE', #8717, #15514, #3096 ) ;
#17937=CARTESIAN_POINT ( 'NONE',  ( 30.28142597461332741, -2.507623461452779701, -4.705209693361160461 ) ) ;
#17949=CIRCLE ( 'NONE', #7514, 6.249999999999998224 ) ;
#17959=CARTESIAN_POINT ( 'NONE',  ( 33.59503905791412137, -1.808589744724287129, -4.533357778048659803 ) ) ;
#17962=AXIS2_PLACEMENT_3D ( 'NONE', #14044, #1441, #11110 ) ;
#17965=CARTESIAN_POINT ( 'NONE',  ( 25.01746843935482190, -10.28886876799018246, -14.47312570928799680 ) ) ;
#17967=CARTESIAN_POINT ( 'NONE',  ( 25.89388370423996832, -3.884438240559767053, -3.881334880282079514 ) ) ;
ENDSEC;
END-ISO-10303-21;
